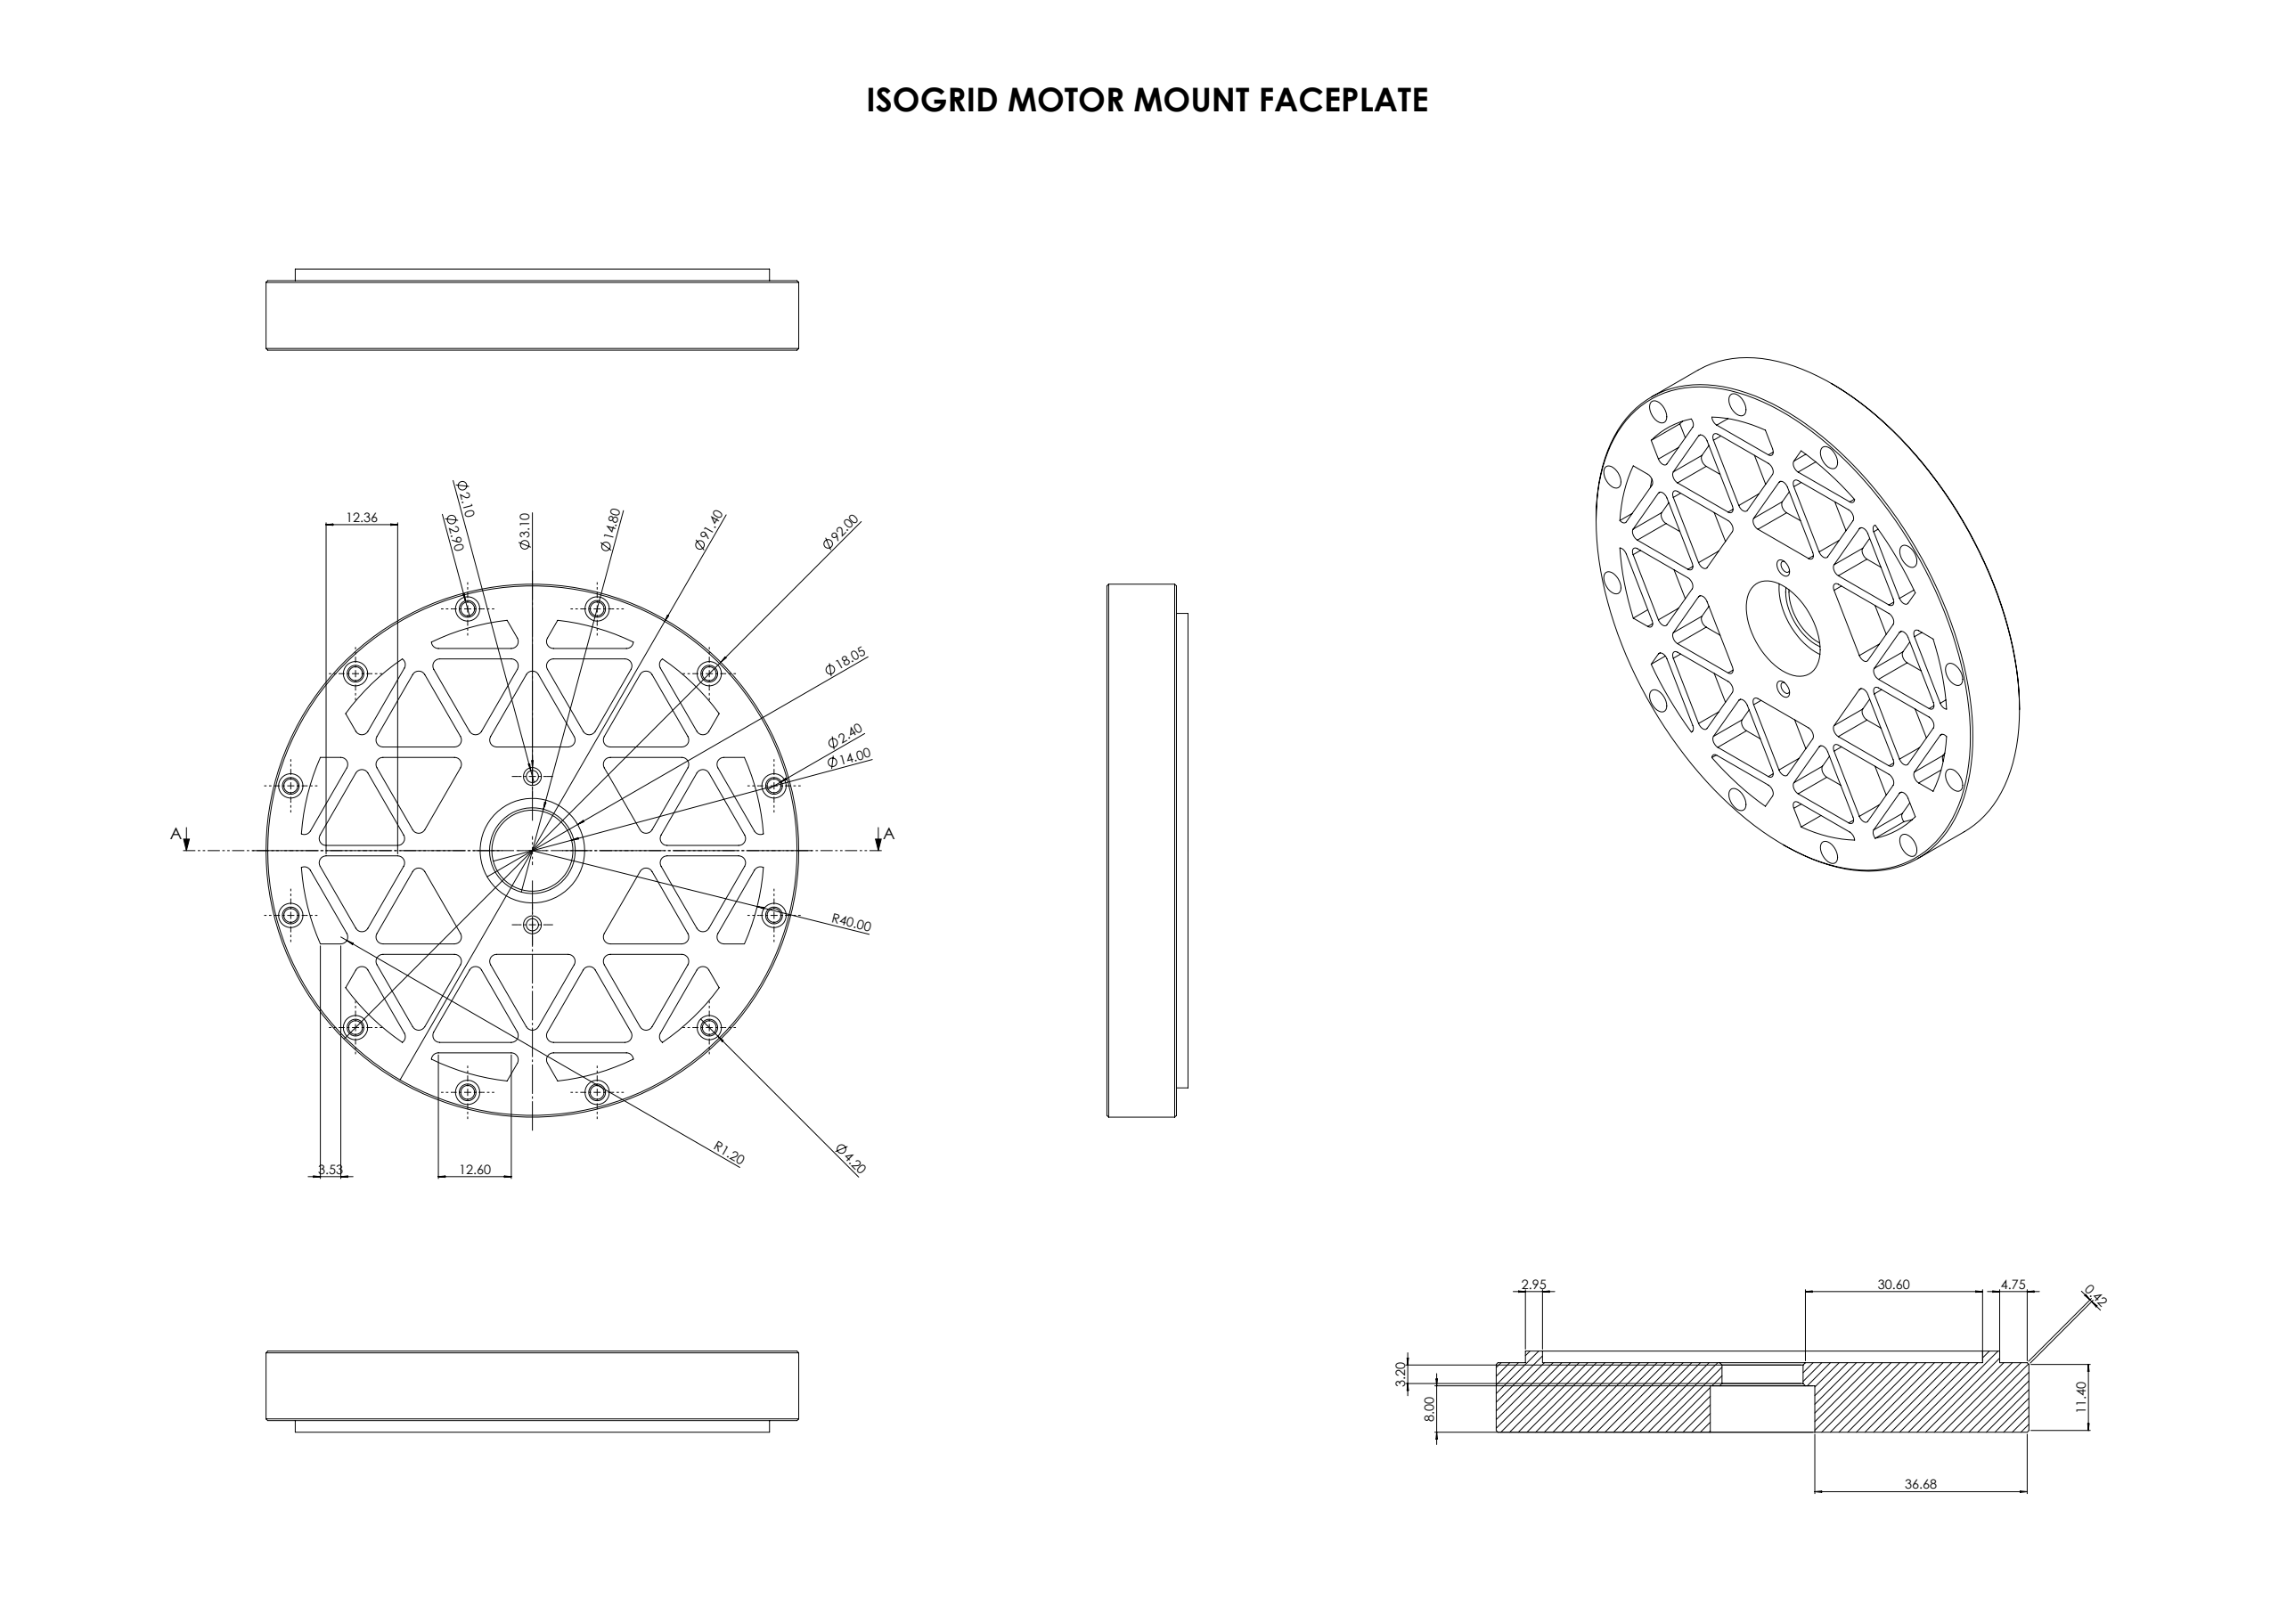
ISO-10303-21;
HEADER;
/* Generated by software containing ST-Developer
 * from STEP Tools, Inc. (www.steptools.com) 
 */

FILE_DESCRIPTION(
/* description */ (''),
/* implementation_level */ '2;1');

FILE_NAME(
/* name */ '03_Isogrid_Motor_Mount_Faceplate.step',
/* time_stamp */ '2026-10-19T23:00:43-07:00',
/* author */ (''),
/* organization */ (''),
/* preprocessor_version */ 'ST-DEVELOPER v20.2',
/* originating_system */ 'Autodesk Translation Framework v15.15.0.0',
/* authorisation */ '');

FILE_SCHEMA (('AUTOMOTIVE_DESIGN { 1 0 10303 214 3 1 1 }'));
ENDSEC;

DATA;
#10=MECHANICAL_DESIGN_GEOMETRIC_PRESENTATION_REPRESENTATION('',(#998),#55002);
#958=SHAPE_REPRESENTATION_RELATIONSHIP('SRR','None',#55106,#978);
#978=ADVANCED_BREP_SHAPE_REPRESENTATION('',(#1018),#54984);
#998=STYLED_ITEM('',(#55400),#1018);
#1018=MANIFOLD_SOLID_BREP('Isogrid Faceplate',#24531);
#1082=FACE_BOUND('',#3973,.T.);
#1083=FACE_BOUND('',#3979,.T.);
#1084=FACE_BOUND('',#3985,.T.);
#1085=FACE_BOUND('',#3991,.T.);
#1086=FACE_BOUND('',#3997,.T.);
#1087=FACE_BOUND('',#4003,.T.);
#1088=FACE_BOUND('',#4009,.T.);
#1089=FACE_BOUND('',#4015,.T.);
#1090=FACE_BOUND('',#4021,.T.);
#1091=FACE_BOUND('',#4027,.T.);
#1092=FACE_BOUND('',#4033,.T.);
#1093=FACE_BOUND('',#4039,.T.);
#1094=FACE_BOUND('',#4044,.T.);
#1095=FACE_BOUND('',#4045,.T.);
#1096=FACE_BOUND('',#4046,.T.);
#1097=FACE_BOUND('',#4047,.T.);
#1098=FACE_BOUND('',#4050,.T.);
#1099=FACE_BOUND('',#4054,.T.);
#1100=FACE_BOUND('',#4055,.T.);
#1101=FACE_BOUND('',#4056,.T.);
#1102=FACE_BOUND('',#4057,.T.);
#1103=FACE_BOUND('',#4058,.T.);
#1104=FACE_BOUND('',#4059,.T.);
#1105=FACE_BOUND('',#4060,.T.);
#1106=FACE_BOUND('',#4061,.T.);
#1107=FACE_BOUND('',#4062,.T.);
#1108=FACE_BOUND('',#4063,.T.);
#1109=FACE_BOUND('',#4064,.T.);
#1110=FACE_BOUND('',#4065,.T.);
#1111=FACE_BOUND('',#4066,.T.);
#1112=FACE_BOUND('',#4069,.T.);
#1113=FACE_BOUND('',#4070,.T.);
#1114=FACE_BOUND('',#4071,.T.);
#1115=FACE_BOUND('',#4072,.T.);
#1116=FACE_BOUND('',#4073,.T.);
#1117=FACE_BOUND('',#4074,.T.);
#1118=FACE_BOUND('',#4075,.T.);
#1119=FACE_BOUND('',#4076,.T.);
#1120=FACE_BOUND('',#4077,.T.);
#1121=FACE_BOUND('',#4078,.T.);
#1122=FACE_BOUND('',#4079,.T.);
#1123=FACE_BOUND('',#4080,.T.);
#1124=FACE_BOUND('',#4081,.T.);
#1125=FACE_BOUND('',#4082,.T.);
#1126=FACE_BOUND('',#4083,.T.);
#1127=FACE_BOUND('',#4084,.T.);
#1128=FACE_BOUND('',#4085,.T.);
#1129=FACE_BOUND('',#4086,.T.);
#1130=FACE_BOUND('',#4087,.T.);
#1131=FACE_BOUND('',#4088,.T.);
#1132=FACE_BOUND('',#4089,.T.);
#1133=FACE_BOUND('',#4090,.T.);
#1134=FACE_BOUND('',#4091,.T.);
#1135=FACE_BOUND('',#4092,.T.);
#1136=FACE_BOUND('',#4093,.T.);
#1137=FACE_BOUND('',#4094,.T.);
#1138=FACE_BOUND('',#4095,.T.);
#1139=FACE_BOUND('',#4096,.T.);
#1140=FACE_BOUND('',#4097,.T.);
#1141=FACE_BOUND('',#4098,.T.);
#1142=FACE_BOUND('',#4099,.T.);
#1143=FACE_BOUND('',#4100,.T.);
#1144=FACE_BOUND('',#4101,.T.);
#1145=FACE_BOUND('',#4102,.T.);
#1146=FACE_BOUND('',#4103,.T.);
#1147=FACE_BOUND('',#4104,.T.);
#1148=FACE_BOUND('',#4105,.T.);
#1149=FACE_BOUND('',#4106,.T.);
#1150=FACE_BOUND('',#4107,.T.);
#1151=FACE_BOUND('',#4108,.T.);
#1152=FACE_BOUND('',#4109,.T.);
#1153=FACE_BOUND('',#4110,.T.);
#1154=FACE_BOUND('',#4111,.T.);
#1155=FACE_BOUND('',#4112,.T.);
#1156=FACE_BOUND('',#4113,.T.);
#1157=FACE_BOUND('',#4314,.T.);
#1289=PLANE('',#25096);
#1290=PLANE('',#25107);
#1291=PLANE('',#25118);
#1292=PLANE('',#25129);
#1293=PLANE('',#25140);
#1294=PLANE('',#25151);
#1295=PLANE('',#25162);
#1296=PLANE('',#25173);
#1297=PLANE('',#25184);
#1298=PLANE('',#25195);
#1299=PLANE('',#25206);
#1300=PLANE('',#25217);
#1301=PLANE('',#25228);
#1302=PLANE('',#25232);
#1303=PLANE('',#25241);
#1304=PLANE('',#25245);
#1305=PLANE('',#25341);
#1306=PLANE('',#25344);
#1307=PLANE('',#25348);
#1308=PLANE('',#25351);
#1309=PLANE('',#25353);
#1310=PLANE('',#25357);
#1311=PLANE('',#25360);
#1312=PLANE('',#25362);
#1313=PLANE('',#25368);
#1314=PLANE('',#25371);
#1315=PLANE('',#25373);
#1316=PLANE('',#25377);
#1317=PLANE('',#25380);
#1318=PLANE('',#25382);
#1319=PLANE('',#25386);
#1320=PLANE('',#25389);
#1321=PLANE('',#25392);
#1322=PLANE('',#25396);
#1323=PLANE('',#25399);
#1324=PLANE('',#25401);
#1325=PLANE('',#25405);
#1326=PLANE('',#25408);
#1327=PLANE('',#25410);
#1328=PLANE('',#25414);
#1329=PLANE('',#25417);
#1330=PLANE('',#25419);
#1331=PLANE('',#25422);
#1332=PLANE('',#25425);
#1333=PLANE('',#25427);
#1334=PLANE('',#25431);
#1335=PLANE('',#25434);
#1336=PLANE('',#25436);
#1337=PLANE('',#25440);
#1338=PLANE('',#25443);
#1339=PLANE('',#25446);
#1340=PLANE('',#25450);
#1341=PLANE('',#25453);
#1342=PLANE('',#25455);
#1343=PLANE('',#25459);
#1344=PLANE('',#25462);
#1345=PLANE('',#25464);
#1346=PLANE('',#25468);
#1347=PLANE('',#25471);
#1348=PLANE('',#25473);
#1349=PLANE('',#25479);
#1350=PLANE('',#25482);
#1351=PLANE('',#25484);
#1352=PLANE('',#25488);
#1353=PLANE('',#25491);
#1354=PLANE('',#25493);
#1355=PLANE('',#25497);
#1356=PLANE('',#25500);
#1357=PLANE('',#25502);
#1358=PLANE('',#25505);
#1359=PLANE('',#25508);
#1360=PLANE('',#25510);
#1361=PLANE('',#25514);
#1362=PLANE('',#25517);
#1363=PLANE('',#25519);
#1364=PLANE('',#25525);
#1365=PLANE('',#25527);
#1366=PLANE('',#25530);
#1367=PLANE('',#25533);
#1368=PLANE('',#25535);
#1369=PLANE('',#25539);
#1370=PLANE('',#25542);
#1371=PLANE('',#25544);
#1372=PLANE('',#25548);
#1373=PLANE('',#25551);
#1374=PLANE('',#25553);
#1375=PLANE('',#25557);
#1376=PLANE('',#25559);
#1377=PLANE('',#25562);
#1378=PLANE('',#25565);
#1379=PLANE('',#25569);
#1380=PLANE('',#25571);
#1381=PLANE('',#25574);
#1382=PLANE('',#25578);
#1383=PLANE('',#25580);
#1384=PLANE('',#25583);
#1385=PLANE('',#25597);
#1386=PLANE('',#25598);
#1387=PLANE('',#25599);
#1388=PLANE('',#25600);
#1389=PLANE('',#25601);
#1390=PLANE('',#25602);
#1391=PLANE('',#25603);
#1392=PLANE('',#25604);
#1393=PLANE('',#25605);
#1394=PLANE('',#25606);
#1395=PLANE('',#25607);
#1396=PLANE('',#25608);
#1397=PLANE('',#25609);
#1398=PLANE('',#25610);
#1399=PLANE('',#25611);
#1400=PLANE('',#25612);
#1401=PLANE('',#25613);
#1402=PLANE('',#25614);
#1403=PLANE('',#25615);
#1404=PLANE('',#25616);
#1405=PLANE('',#25617);
#1406=PLANE('',#25618);
#1407=PLANE('',#25619);
#1408=PLANE('',#25620);
#1409=PLANE('',#25621);
#1410=PLANE('',#25622);
#1411=PLANE('',#25623);
#1412=PLANE('',#25624);
#1413=PLANE('',#25627);
#1992=CYLINDRICAL_SURFACE('',#25061,0.105);
#1993=CYLINDRICAL_SURFACE('',#25067,0.105);
#1994=CYLINDRICAL_SURFACE('',#25073,0.13);
#1995=CYLINDRICAL_SURFACE('',#25079,0.13);
#1996=CYLINDRICAL_SURFACE('',#25085,0.13);
#1997=CYLINDRICAL_SURFACE('',#25092,0.12);
#1998=CYLINDRICAL_SURFACE('',#25098,0.21);
#1999=CYLINDRICAL_SURFACE('',#25103,0.12);
#2000=CYLINDRICAL_SURFACE('',#25109,0.21);
#2001=CYLINDRICAL_SURFACE('',#25114,0.12);
#2002=CYLINDRICAL_SURFACE('',#25120,0.21);
#2003=CYLINDRICAL_SURFACE('',#25125,0.12);
#2004=CYLINDRICAL_SURFACE('',#25131,0.21);
#2005=CYLINDRICAL_SURFACE('',#25136,0.12);
#2006=CYLINDRICAL_SURFACE('',#25142,0.21);
#2007=CYLINDRICAL_SURFACE('',#25147,0.120000000000001);
#2008=CYLINDRICAL_SURFACE('',#25153,0.21);
#2009=CYLINDRICAL_SURFACE('',#25158,0.12);
#2010=CYLINDRICAL_SURFACE('',#25164,0.21);
#2011=CYLINDRICAL_SURFACE('',#25169,0.12);
#2012=CYLINDRICAL_SURFACE('',#25175,0.21);
#2013=CYLINDRICAL_SURFACE('',#25180,0.12);
#2014=CYLINDRICAL_SURFACE('',#25186,0.21);
#2015=CYLINDRICAL_SURFACE('',#25191,0.12);
#2016=CYLINDRICAL_SURFACE('',#25197,0.21);
#2017=CYLINDRICAL_SURFACE('',#25202,0.12);
#2018=CYLINDRICAL_SURFACE('',#25208,0.21);
#2019=CYLINDRICAL_SURFACE('',#25213,0.12);
#2020=CYLINDRICAL_SURFACE('',#25219,0.21);
#2021=CYLINDRICAL_SURFACE('',#25225,0.7);
#2022=CYLINDRICAL_SURFACE('',#25238,4.6);
#2023=CYLINDRICAL_SURFACE('',#25337,0.12);
#2024=CYLINDRICAL_SURFACE('',#25339,0.12);
#2025=CYLINDRICAL_SURFACE('',#25342,0.12);
#2026=CYLINDRICAL_SURFACE('',#25346,0.12);
#2027=CYLINDRICAL_SURFACE('',#25349,0.12);
#2028=CYLINDRICAL_SURFACE('',#25354,0.12);
#2029=CYLINDRICAL_SURFACE('',#25355,0.12);
#2030=CYLINDRICAL_SURFACE('',#25358,0.12);
#2031=CYLINDRICAL_SURFACE('',#25363,0.12);
#2032=CYLINDRICAL_SURFACE('',#25364,0.12);
#2033=CYLINDRICAL_SURFACE('',#25366,0.12);
#2034=CYLINDRICAL_SURFACE('',#25369,0.12);
#2035=CYLINDRICAL_SURFACE('',#25374,0.12);
#2036=CYLINDRICAL_SURFACE('',#25375,0.12);
#2037=CYLINDRICAL_SURFACE('',#25378,0.12);
#2038=CYLINDRICAL_SURFACE('',#25383,0.12);
#2039=CYLINDRICAL_SURFACE('',#25384,0.12);
#2040=CYLINDRICAL_SURFACE('',#25387,0.12);
#2041=CYLINDRICAL_SURFACE('',#25393,0.12);
#2042=CYLINDRICAL_SURFACE('',#25394,0.12);
#2043=CYLINDRICAL_SURFACE('',#25397,0.12);
#2044=CYLINDRICAL_SURFACE('',#25402,0.12);
#2045=CYLINDRICAL_SURFACE('',#25403,0.12);
#2046=CYLINDRICAL_SURFACE('',#25406,0.12);
#2047=CYLINDRICAL_SURFACE('',#25411,0.12);
#2048=CYLINDRICAL_SURFACE('',#25412,0.12);
#2049=CYLINDRICAL_SURFACE('',#25418,0.12);
#2050=CYLINDRICAL_SURFACE('',#25420,0.12);
#2051=CYLINDRICAL_SURFACE('',#25423,0.12);
#2052=CYLINDRICAL_SURFACE('',#25428,0.12);
#2053=CYLINDRICAL_SURFACE('',#25429,0.12);
#2054=CYLINDRICAL_SURFACE('',#25432,0.12);
#2055=CYLINDRICAL_SURFACE('',#25437,0.12);
#2056=CYLINDRICAL_SURFACE('',#25438,0.12);
#2057=CYLINDRICAL_SURFACE('',#25441,0.12);
#2058=CYLINDRICAL_SURFACE('',#25447,0.12);
#2059=CYLINDRICAL_SURFACE('',#25448,0.12);
#2060=CYLINDRICAL_SURFACE('',#25451,0.12);
#2061=CYLINDRICAL_SURFACE('',#25456,0.12);
#2062=CYLINDRICAL_SURFACE('',#25457,0.12);
#2063=CYLINDRICAL_SURFACE('',#25460,0.12);
#2064=CYLINDRICAL_SURFACE('',#25465,0.12);
#2065=CYLINDRICAL_SURFACE('',#25466,0.12);
#2066=CYLINDRICAL_SURFACE('',#25469,0.12);
#2067=CYLINDRICAL_SURFACE('',#25474,0.12);
#2068=CYLINDRICAL_SURFACE('',#25475,0.12);
#2069=CYLINDRICAL_SURFACE('',#25477,0.12);
#2070=CYLINDRICAL_SURFACE('',#25480,0.12);
#2071=CYLINDRICAL_SURFACE('',#25485,0.12);
#2072=CYLINDRICAL_SURFACE('',#25486,0.12);
#2073=CYLINDRICAL_SURFACE('',#25489,0.12);
#2074=CYLINDRICAL_SURFACE('',#25494,0.12);
#2075=CYLINDRICAL_SURFACE('',#25495,0.12);
#2076=CYLINDRICAL_SURFACE('',#25501,0.12);
#2077=CYLINDRICAL_SURFACE('',#25503,0.12);
#2078=CYLINDRICAL_SURFACE('',#25506,0.12);
#2079=CYLINDRICAL_SURFACE('',#25511,0.12);
#2080=CYLINDRICAL_SURFACE('',#25512,0.12);
#2081=CYLINDRICAL_SURFACE('',#25515,0.12);
#2082=CYLINDRICAL_SURFACE('',#25520,0.12);
#2083=CYLINDRICAL_SURFACE('',#25521,0.12);
#2084=CYLINDRICAL_SURFACE('',#25523,0.12);
#2085=CYLINDRICAL_SURFACE('',#25528,0.12);
#2086=CYLINDRICAL_SURFACE('',#25531,0.12);
#2087=CYLINDRICAL_SURFACE('',#25536,0.12);
#2088=CYLINDRICAL_SURFACE('',#25537,0.12);
#2089=CYLINDRICAL_SURFACE('',#25540,0.12);
#2090=CYLINDRICAL_SURFACE('',#25545,0.12);
#2091=CYLINDRICAL_SURFACE('',#25546,0.12);
#2092=CYLINDRICAL_SURFACE('',#25549,0.12);
#2093=CYLINDRICAL_SURFACE('',#25554,0.12);
#2094=CYLINDRICAL_SURFACE('',#25555,0.12);
#2095=CYLINDRICAL_SURFACE('',#25560,0.12);
#2096=CYLINDRICAL_SURFACE('',#25563,0.12);
#2097=CYLINDRICAL_SURFACE('',#25567,0.12);
#2098=CYLINDRICAL_SURFACE('',#25572,0.12);
#2099=CYLINDRICAL_SURFACE('',#25576,0.12);
#2100=CYLINDRICAL_SURFACE('',#25581,0.12);
#2101=CYLINDRICAL_SURFACE('',#25585,4.);
#2102=CYLINDRICAL_SURFACE('',#25586,4.);
#2103=CYLINDRICAL_SURFACE('',#25587,4.);
#2104=CYLINDRICAL_SURFACE('',#25588,4.);
#2105=CYLINDRICAL_SURFACE('',#25589,4.);
#2106=CYLINDRICAL_SURFACE('',#25590,4.);
#2107=CYLINDRICAL_SURFACE('',#25591,4.);
#2108=CYLINDRICAL_SURFACE('',#25592,4.);
#2109=CYLINDRICAL_SURFACE('',#25593,4.);
#2110=CYLINDRICAL_SURFACE('',#25594,4.);
#2111=CYLINDRICAL_SURFACE('',#25595,4.);
#2112=CYLINDRICAL_SURFACE('',#25596,4.);
#2113=CYLINDRICAL_SURFACE('',#25625,3.8);
#2114=CYLINDRICAL_SURFACE('',#25629,4.095);
#2115=CYLINDRICAL_SURFACE('',#25630,0.9025);
#2544=FACE_OUTER_BOUND('',#3954,.T.);
#2545=FACE_OUTER_BOUND('',#3955,.T.);
#2546=FACE_OUTER_BOUND('',#3956,.T.);
#2547=FACE_OUTER_BOUND('',#3957,.T.);
#2548=FACE_OUTER_BOUND('',#3958,.T.);
#2549=FACE_OUTER_BOUND('',#3959,.T.);
#2550=FACE_OUTER_BOUND('',#3960,.T.);
#2551=FACE_OUTER_BOUND('',#3961,.T.);
#2552=FACE_OUTER_BOUND('',#3962,.T.);
#2553=FACE_OUTER_BOUND('',#3963,.T.);
#2554=FACE_OUTER_BOUND('',#3964,.T.);
#2555=FACE_OUTER_BOUND('',#3965,.T.);
#2556=FACE_OUTER_BOUND('',#3966,.T.);
#2557=FACE_OUTER_BOUND('',#3967,.T.);
#2558=FACE_OUTER_BOUND('',#3968,.T.);
#2559=FACE_OUTER_BOUND('',#3969,.T.);
#2560=FACE_OUTER_BOUND('',#3970,.T.);
#2561=FACE_OUTER_BOUND('',#3971,.T.);
#2562=FACE_OUTER_BOUND('',#3972,.T.);
#2563=FACE_OUTER_BOUND('',#3974,.T.);
#2564=FACE_OUTER_BOUND('',#3975,.T.);
#2565=FACE_OUTER_BOUND('',#3976,.T.);
#2566=FACE_OUTER_BOUND('',#3977,.T.);
#2567=FACE_OUTER_BOUND('',#3978,.T.);
#2568=FACE_OUTER_BOUND('',#3980,.T.);
#2569=FACE_OUTER_BOUND('',#3981,.T.);
#2570=FACE_OUTER_BOUND('',#3982,.T.);
#2571=FACE_OUTER_BOUND('',#3983,.T.);
#2572=FACE_OUTER_BOUND('',#3984,.T.);
#2573=FACE_OUTER_BOUND('',#3986,.T.);
#2574=FACE_OUTER_BOUND('',#3987,.T.);
#2575=FACE_OUTER_BOUND('',#3988,.T.);
#2576=FACE_OUTER_BOUND('',#3989,.T.);
#2577=FACE_OUTER_BOUND('',#3990,.T.);
#2578=FACE_OUTER_BOUND('',#3992,.T.);
#2579=FACE_OUTER_BOUND('',#3993,.T.);
#2580=FACE_OUTER_BOUND('',#3994,.T.);
#2581=FACE_OUTER_BOUND('',#3995,.T.);
#2582=FACE_OUTER_BOUND('',#3996,.T.);
#2583=FACE_OUTER_BOUND('',#3998,.T.);
#2584=FACE_OUTER_BOUND('',#3999,.T.);
#2585=FACE_OUTER_BOUND('',#4000,.T.);
#2586=FACE_OUTER_BOUND('',#4001,.T.);
#2587=FACE_OUTER_BOUND('',#4002,.T.);
#2588=FACE_OUTER_BOUND('',#4004,.T.);
#2589=FACE_OUTER_BOUND('',#4005,.T.);
#2590=FACE_OUTER_BOUND('',#4006,.T.);
#2591=FACE_OUTER_BOUND('',#4007,.T.);
#2592=FACE_OUTER_BOUND('',#4008,.T.);
#2593=FACE_OUTER_BOUND('',#4010,.T.);
#2594=FACE_OUTER_BOUND('',#4011,.T.);
#2595=FACE_OUTER_BOUND('',#4012,.T.);
#2596=FACE_OUTER_BOUND('',#4013,.T.);
#2597=FACE_OUTER_BOUND('',#4014,.T.);
#2598=FACE_OUTER_BOUND('',#4016,.T.);
#2599=FACE_OUTER_BOUND('',#4017,.T.);
#2600=FACE_OUTER_BOUND('',#4018,.T.);
#2601=FACE_OUTER_BOUND('',#4019,.T.);
#2602=FACE_OUTER_BOUND('',#4020,.T.);
#2603=FACE_OUTER_BOUND('',#4022,.T.);
#2604=FACE_OUTER_BOUND('',#4023,.T.);
#2605=FACE_OUTER_BOUND('',#4024,.T.);
#2606=FACE_OUTER_BOUND('',#4025,.T.);
#2607=FACE_OUTER_BOUND('',#4026,.T.);
#2608=FACE_OUTER_BOUND('',#4028,.T.);
#2609=FACE_OUTER_BOUND('',#4029,.T.);
#2610=FACE_OUTER_BOUND('',#4030,.T.);
#2611=FACE_OUTER_BOUND('',#4031,.T.);
#2612=FACE_OUTER_BOUND('',#4032,.T.);
#2613=FACE_OUTER_BOUND('',#4034,.T.);
#2614=FACE_OUTER_BOUND('',#4035,.T.);
#2615=FACE_OUTER_BOUND('',#4036,.T.);
#2616=FACE_OUTER_BOUND('',#4037,.T.);
#2617=FACE_OUTER_BOUND('',#4038,.T.);
#2618=FACE_OUTER_BOUND('',#4040,.T.);
#2619=FACE_OUTER_BOUND('',#4041,.T.);
#2620=FACE_OUTER_BOUND('',#4042,.T.);
#2621=FACE_OUTER_BOUND('',#4043,.T.);
#2622=FACE_OUTER_BOUND('',#4048,.T.);
#2623=FACE_OUTER_BOUND('',#4049,.T.);
#2624=FACE_OUTER_BOUND('',#4051,.T.);
#2625=FACE_OUTER_BOUND('',#4052,.T.);
#2626=FACE_OUTER_BOUND('',#4053,.T.);
#2627=FACE_OUTER_BOUND('',#4067,.T.);
#2628=FACE_OUTER_BOUND('',#4068,.T.);
#2629=FACE_OUTER_BOUND('',#4114,.T.);
#2630=FACE_OUTER_BOUND('',#4115,.T.);
#2631=FACE_OUTER_BOUND('',#4116,.T.);
#2632=FACE_OUTER_BOUND('',#4117,.T.);
#2633=FACE_OUTER_BOUND('',#4118,.T.);
#2634=FACE_OUTER_BOUND('',#4119,.T.);
#2635=FACE_OUTER_BOUND('',#4120,.T.);
#2636=FACE_OUTER_BOUND('',#4121,.T.);
#2637=FACE_OUTER_BOUND('',#4122,.T.);
#2638=FACE_OUTER_BOUND('',#4123,.T.);
#2639=FACE_OUTER_BOUND('',#4124,.T.);
#2640=FACE_OUTER_BOUND('',#4125,.T.);
#2641=FACE_OUTER_BOUND('',#4126,.T.);
#2642=FACE_OUTER_BOUND('',#4127,.T.);
#2643=FACE_OUTER_BOUND('',#4128,.T.);
#2644=FACE_OUTER_BOUND('',#4129,.T.);
#2645=FACE_OUTER_BOUND('',#4130,.T.);
#2646=FACE_OUTER_BOUND('',#4131,.T.);
#2647=FACE_OUTER_BOUND('',#4132,.T.);
#2648=FACE_OUTER_BOUND('',#4133,.T.);
#2649=FACE_OUTER_BOUND('',#4134,.T.);
#2650=FACE_OUTER_BOUND('',#4135,.T.);
#2651=FACE_OUTER_BOUND('',#4136,.T.);
#2652=FACE_OUTER_BOUND('',#4137,.T.);
#2653=FACE_OUTER_BOUND('',#4138,.T.);
#2654=FACE_OUTER_BOUND('',#4139,.T.);
#2655=FACE_OUTER_BOUND('',#4140,.T.);
#2656=FACE_OUTER_BOUND('',#4141,.T.);
#2657=FACE_OUTER_BOUND('',#4142,.T.);
#2658=FACE_OUTER_BOUND('',#4143,.T.);
#2659=FACE_OUTER_BOUND('',#4144,.T.);
#2660=FACE_OUTER_BOUND('',#4145,.T.);
#2661=FACE_OUTER_BOUND('',#4146,.T.);
#2662=FACE_OUTER_BOUND('',#4147,.T.);
#2663=FACE_OUTER_BOUND('',#4148,.T.);
#2664=FACE_OUTER_BOUND('',#4149,.T.);
#2665=FACE_OUTER_BOUND('',#4150,.T.);
#2666=FACE_OUTER_BOUND('',#4151,.T.);
#2667=FACE_OUTER_BOUND('',#4152,.T.);
#2668=FACE_OUTER_BOUND('',#4153,.T.);
#2669=FACE_OUTER_BOUND('',#4154,.T.);
#2670=FACE_OUTER_BOUND('',#4155,.T.);
#2671=FACE_OUTER_BOUND('',#4156,.T.);
#2672=FACE_OUTER_BOUND('',#4157,.T.);
#2673=FACE_OUTER_BOUND('',#4158,.T.);
#2674=FACE_OUTER_BOUND('',#4159,.T.);
#2675=FACE_OUTER_BOUND('',#4160,.T.);
#2676=FACE_OUTER_BOUND('',#4161,.T.);
#2677=FACE_OUTER_BOUND('',#4162,.T.);
#2678=FACE_OUTER_BOUND('',#4163,.T.);
#2679=FACE_OUTER_BOUND('',#4164,.T.);
#2680=FACE_OUTER_BOUND('',#4165,.T.);
#2681=FACE_OUTER_BOUND('',#4166,.T.);
#2682=FACE_OUTER_BOUND('',#4167,.T.);
#2683=FACE_OUTER_BOUND('',#4168,.T.);
#2684=FACE_OUTER_BOUND('',#4169,.T.);
#2685=FACE_OUTER_BOUND('',#4170,.T.);
#2686=FACE_OUTER_BOUND('',#4171,.T.);
#2687=FACE_OUTER_BOUND('',#4172,.T.);
#2688=FACE_OUTER_BOUND('',#4173,.T.);
#2689=FACE_OUTER_BOUND('',#4174,.T.);
#2690=FACE_OUTER_BOUND('',#4175,.T.);
#2691=FACE_OUTER_BOUND('',#4176,.T.);
#2692=FACE_OUTER_BOUND('',#4177,.T.);
#2693=FACE_OUTER_BOUND('',#4178,.T.);
#2694=FACE_OUTER_BOUND('',#4179,.T.);
#2695=FACE_OUTER_BOUND('',#4180,.T.);
#2696=FACE_OUTER_BOUND('',#4181,.T.);
#2697=FACE_OUTER_BOUND('',#4182,.T.);
#2698=FACE_OUTER_BOUND('',#4183,.T.);
#2699=FACE_OUTER_BOUND('',#4184,.T.);
#2700=FACE_OUTER_BOUND('',#4185,.T.);
#2701=FACE_OUTER_BOUND('',#4186,.T.);
#2702=FACE_OUTER_BOUND('',#4187,.T.);
#2703=FACE_OUTER_BOUND('',#4188,.T.);
#2704=FACE_OUTER_BOUND('',#4189,.T.);
#2705=FACE_OUTER_BOUND('',#4190,.T.);
#2706=FACE_OUTER_BOUND('',#4191,.T.);
#2707=FACE_OUTER_BOUND('',#4192,.T.);
#2708=FACE_OUTER_BOUND('',#4193,.T.);
#2709=FACE_OUTER_BOUND('',#4194,.T.);
#2710=FACE_OUTER_BOUND('',#4195,.T.);
#2711=FACE_OUTER_BOUND('',#4196,.T.);
#2712=FACE_OUTER_BOUND('',#4197,.T.);
#2713=FACE_OUTER_BOUND('',#4198,.T.);
#2714=FACE_OUTER_BOUND('',#4199,.T.);
#2715=FACE_OUTER_BOUND('',#4200,.T.);
#2716=FACE_OUTER_BOUND('',#4201,.T.);
#2717=FACE_OUTER_BOUND('',#4202,.T.);
#2718=FACE_OUTER_BOUND('',#4203,.T.);
#2719=FACE_OUTER_BOUND('',#4204,.T.);
#2720=FACE_OUTER_BOUND('',#4205,.T.);
#2721=FACE_OUTER_BOUND('',#4206,.T.);
#2722=FACE_OUTER_BOUND('',#4207,.T.);
#2723=FACE_OUTER_BOUND('',#4208,.T.);
#2724=FACE_OUTER_BOUND('',#4209,.T.);
#2725=FACE_OUTER_BOUND('',#4210,.T.);
#2726=FACE_OUTER_BOUND('',#4211,.T.);
#2727=FACE_OUTER_BOUND('',#4212,.T.);
#2728=FACE_OUTER_BOUND('',#4213,.T.);
#2729=FACE_OUTER_BOUND('',#4214,.T.);
#2730=FACE_OUTER_BOUND('',#4215,.T.);
#2731=FACE_OUTER_BOUND('',#4216,.T.);
#2732=FACE_OUTER_BOUND('',#4217,.T.);
#2733=FACE_OUTER_BOUND('',#4218,.T.);
#2734=FACE_OUTER_BOUND('',#4219,.T.);
#2735=FACE_OUTER_BOUND('',#4220,.T.);
#2736=FACE_OUTER_BOUND('',#4221,.T.);
#2737=FACE_OUTER_BOUND('',#4222,.T.);
#2738=FACE_OUTER_BOUND('',#4223,.T.);
#2739=FACE_OUTER_BOUND('',#4224,.T.);
#2740=FACE_OUTER_BOUND('',#4225,.T.);
#2741=FACE_OUTER_BOUND('',#4226,.T.);
#2742=FACE_OUTER_BOUND('',#4227,.T.);
#2743=FACE_OUTER_BOUND('',#4228,.T.);
#2744=FACE_OUTER_BOUND('',#4229,.T.);
#2745=FACE_OUTER_BOUND('',#4230,.T.);
#2746=FACE_OUTER_BOUND('',#4231,.T.);
#2747=FACE_OUTER_BOUND('',#4232,.T.);
#2748=FACE_OUTER_BOUND('',#4233,.T.);
#2749=FACE_OUTER_BOUND('',#4234,.T.);
#2750=FACE_OUTER_BOUND('',#4235,.T.);
#2751=FACE_OUTER_BOUND('',#4236,.T.);
#2752=FACE_OUTER_BOUND('',#4237,.T.);
#2753=FACE_OUTER_BOUND('',#4238,.T.);
#2754=FACE_OUTER_BOUND('',#4239,.T.);
#2755=FACE_OUTER_BOUND('',#4240,.T.);
#2756=FACE_OUTER_BOUND('',#4241,.T.);
#2757=FACE_OUTER_BOUND('',#4242,.T.);
#2758=FACE_OUTER_BOUND('',#4243,.T.);
#2759=FACE_OUTER_BOUND('',#4244,.T.);
#2760=FACE_OUTER_BOUND('',#4245,.T.);
#2761=FACE_OUTER_BOUND('',#4246,.T.);
#2762=FACE_OUTER_BOUND('',#4247,.T.);
#2763=FACE_OUTER_BOUND('',#4248,.T.);
#2764=FACE_OUTER_BOUND('',#4249,.T.);
#2765=FACE_OUTER_BOUND('',#4250,.T.);
#2766=FACE_OUTER_BOUND('',#4251,.T.);
#2767=FACE_OUTER_BOUND('',#4252,.T.);
#2768=FACE_OUTER_BOUND('',#4253,.T.);
#2769=FACE_OUTER_BOUND('',#4254,.T.);
#2770=FACE_OUTER_BOUND('',#4255,.T.);
#2771=FACE_OUTER_BOUND('',#4256,.T.);
#2772=FACE_OUTER_BOUND('',#4257,.T.);
#2773=FACE_OUTER_BOUND('',#4258,.T.);
#2774=FACE_OUTER_BOUND('',#4259,.T.);
#2775=FACE_OUTER_BOUND('',#4260,.T.);
#2776=FACE_OUTER_BOUND('',#4261,.T.);
#2777=FACE_OUTER_BOUND('',#4262,.T.);
#2778=FACE_OUTER_BOUND('',#4263,.T.);
#2779=FACE_OUTER_BOUND('',#4264,.T.);
#2780=FACE_OUTER_BOUND('',#4265,.T.);
#2781=FACE_OUTER_BOUND('',#4266,.T.);
#2782=FACE_OUTER_BOUND('',#4267,.T.);
#2783=FACE_OUTER_BOUND('',#4268,.T.);
#2784=FACE_OUTER_BOUND('',#4269,.T.);
#2785=FACE_OUTER_BOUND('',#4270,.T.);
#2786=FACE_OUTER_BOUND('',#4271,.T.);
#2787=FACE_OUTER_BOUND('',#4272,.T.);
#2788=FACE_OUTER_BOUND('',#4273,.T.);
#2789=FACE_OUTER_BOUND('',#4274,.T.);
#2790=FACE_OUTER_BOUND('',#4275,.T.);
#2791=FACE_OUTER_BOUND('',#4276,.T.);
#2792=FACE_OUTER_BOUND('',#4277,.T.);
#2793=FACE_OUTER_BOUND('',#4278,.T.);
#2794=FACE_OUTER_BOUND('',#4279,.T.);
#2795=FACE_OUTER_BOUND('',#4280,.T.);
#2796=FACE_OUTER_BOUND('',#4281,.T.);
#2797=FACE_OUTER_BOUND('',#4282,.T.);
#2798=FACE_OUTER_BOUND('',#4283,.T.);
#2799=FACE_OUTER_BOUND('',#4284,.T.);
#2800=FACE_OUTER_BOUND('',#4285,.T.);
#2801=FACE_OUTER_BOUND('',#4286,.T.);
#2802=FACE_OUTER_BOUND('',#4287,.T.);
#2803=FACE_OUTER_BOUND('',#4288,.T.);
#2804=FACE_OUTER_BOUND('',#4289,.T.);
#2805=FACE_OUTER_BOUND('',#4290,.T.);
#2806=FACE_OUTER_BOUND('',#4291,.T.);
#2807=FACE_OUTER_BOUND('',#4292,.T.);
#2808=FACE_OUTER_BOUND('',#4293,.T.);
#2809=FACE_OUTER_BOUND('',#4294,.T.);
#2810=FACE_OUTER_BOUND('',#4295,.T.);
#2811=FACE_OUTER_BOUND('',#4296,.T.);
#2812=FACE_OUTER_BOUND('',#4297,.T.);
#2813=FACE_OUTER_BOUND('',#4298,.T.);
#2814=FACE_OUTER_BOUND('',#4299,.T.);
#2815=FACE_OUTER_BOUND('',#4300,.T.);
#2816=FACE_OUTER_BOUND('',#4301,.T.);
#2817=FACE_OUTER_BOUND('',#4302,.T.);
#2818=FACE_OUTER_BOUND('',#4303,.T.);
#2819=FACE_OUTER_BOUND('',#4304,.T.);
#2820=FACE_OUTER_BOUND('',#4305,.T.);
#2821=FACE_OUTER_BOUND('',#4306,.T.);
#2822=FACE_OUTER_BOUND('',#4307,.T.);
#2823=FACE_OUTER_BOUND('',#4308,.T.);
#2824=FACE_OUTER_BOUND('',#4309,.T.);
#2825=FACE_OUTER_BOUND('',#4310,.T.);
#2826=FACE_OUTER_BOUND('',#4311,.T.);
#2827=FACE_OUTER_BOUND('',#4312,.T.);
#2828=FACE_OUTER_BOUND('',#4313,.T.);
#2829=FACE_OUTER_BOUND('',#4315,.T.);
#2830=FACE_OUTER_BOUND('',#4316,.T.);
#3954=EDGE_LOOP('',(#16430,#16431,#16432));
#3955=EDGE_LOOP('',(#16433,#16434,#16435,#16436));
#3956=EDGE_LOOP('',(#16437,#16438,#16439,#16440));
#3957=EDGE_LOOP('',(#16441,#16442,#16443));
#3958=EDGE_LOOP('',(#16444,#16445,#16446,#16447));
#3959=EDGE_LOOP('',(#16448,#16449,#16450,#16451));
#3960=EDGE_LOOP('',(#16452,#16453,#16454));
#3961=EDGE_LOOP('',(#16455,#16456,#16457,#16458));
#3962=EDGE_LOOP('',(#16459,#16460,#16461,#16462));
#3963=EDGE_LOOP('',(#16463,#16464,#16465));
#3964=EDGE_LOOP('',(#16466,#16467,#16468,#16469));
#3965=EDGE_LOOP('',(#16470,#16471,#16472,#16473));
#3966=EDGE_LOOP('',(#16474,#16475,#16476));
#3967=EDGE_LOOP('',(#16477,#16478,#16479,#16480));
#3968=EDGE_LOOP('',(#16481,#16482,#16483,#16484));
#3969=EDGE_LOOP('',(#16485,#16486,#16487,#16488));
#3970=EDGE_LOOP('',(#16489,#16490,#16491,#16492));
#3971=EDGE_LOOP('',(#16493,#16494,#16495,#16496));
#3972=EDGE_LOOP('',(#16497));
#3973=EDGE_LOOP('',(#16498));
#3974=EDGE_LOOP('',(#16499,#16500,#16501,#16502));
#3975=EDGE_LOOP('',(#16503,#16504,#16505,#16506));
#3976=EDGE_LOOP('',(#16507,#16508,#16509,#16510));
#3977=EDGE_LOOP('',(#16511,#16512,#16513,#16514));
#3978=EDGE_LOOP('',(#16515));
#3979=EDGE_LOOP('',(#16516));
#3980=EDGE_LOOP('',(#16517,#16518,#16519,#16520));
#3981=EDGE_LOOP('',(#16521,#16522,#16523,#16524));
#3982=EDGE_LOOP('',(#16525,#16526,#16527,#16528));
#3983=EDGE_LOOP('',(#16529,#16530,#16531,#16532));
#3984=EDGE_LOOP('',(#16533));
#3985=EDGE_LOOP('',(#16534));
#3986=EDGE_LOOP('',(#16535,#16536,#16537,#16538));
#3987=EDGE_LOOP('',(#16539,#16540,#16541,#16542));
#3988=EDGE_LOOP('',(#16543,#16544,#16545,#16546));
#3989=EDGE_LOOP('',(#16547,#16548,#16549,#16550));
#3990=EDGE_LOOP('',(#16551));
#3991=EDGE_LOOP('',(#16552));
#3992=EDGE_LOOP('',(#16553,#16554,#16555,#16556));
#3993=EDGE_LOOP('',(#16557,#16558,#16559,#16560));
#3994=EDGE_LOOP('',(#16561,#16562,#16563,#16564));
#3995=EDGE_LOOP('',(#16565,#16566,#16567,#16568));
#3996=EDGE_LOOP('',(#16569));
#3997=EDGE_LOOP('',(#16570));
#3998=EDGE_LOOP('',(#16571,#16572,#16573,#16574));
#3999=EDGE_LOOP('',(#16575,#16576,#16577,#16578));
#4000=EDGE_LOOP('',(#16579,#16580,#16581,#16582));
#4001=EDGE_LOOP('',(#16583,#16584,#16585,#16586));
#4002=EDGE_LOOP('',(#16587));
#4003=EDGE_LOOP('',(#16588));
#4004=EDGE_LOOP('',(#16589,#16590,#16591,#16592));
#4005=EDGE_LOOP('',(#16593,#16594,#16595,#16596));
#4006=EDGE_LOOP('',(#16597,#16598,#16599,#16600));
#4007=EDGE_LOOP('',(#16601,#16602,#16603,#16604));
#4008=EDGE_LOOP('',(#16605));
#4009=EDGE_LOOP('',(#16606));
#4010=EDGE_LOOP('',(#16607,#16608,#16609,#16610));
#4011=EDGE_LOOP('',(#16611,#16612,#16613,#16614));
#4012=EDGE_LOOP('',(#16615,#16616,#16617,#16618));
#4013=EDGE_LOOP('',(#16619,#16620,#16621,#16622));
#4014=EDGE_LOOP('',(#16623));
#4015=EDGE_LOOP('',(#16624));
#4016=EDGE_LOOP('',(#16625,#16626,#16627,#16628));
#4017=EDGE_LOOP('',(#16629,#16630,#16631,#16632));
#4018=EDGE_LOOP('',(#16633,#16634,#16635,#16636));
#4019=EDGE_LOOP('',(#16637,#16638,#16639,#16640));
#4020=EDGE_LOOP('',(#16641));
#4021=EDGE_LOOP('',(#16642));
#4022=EDGE_LOOP('',(#16643,#16644,#16645,#16646));
#4023=EDGE_LOOP('',(#16647,#16648,#16649,#16650));
#4024=EDGE_LOOP('',(#16651,#16652,#16653,#16654));
#4025=EDGE_LOOP('',(#16655,#16656,#16657,#16658));
#4026=EDGE_LOOP('',(#16659));
#4027=EDGE_LOOP('',(#16660));
#4028=EDGE_LOOP('',(#16661,#16662,#16663,#16664));
#4029=EDGE_LOOP('',(#16665,#16666,#16667,#16668));
#4030=EDGE_LOOP('',(#16669,#16670,#16671,#16672));
#4031=EDGE_LOOP('',(#16673,#16674,#16675,#16676));
#4032=EDGE_LOOP('',(#16677));
#4033=EDGE_LOOP('',(#16678));
#4034=EDGE_LOOP('',(#16679,#16680,#16681,#16682));
#4035=EDGE_LOOP('',(#16683,#16684,#16685,#16686));
#4036=EDGE_LOOP('',(#16687,#16688,#16689,#16690));
#4037=EDGE_LOOP('',(#16691,#16692,#16693,#16694));
#4038=EDGE_LOOP('',(#16695));
#4039=EDGE_LOOP('',(#16696));
#4040=EDGE_LOOP('',(#16697,#16698,#16699,#16700));
#4041=EDGE_LOOP('',(#16701,#16702,#16703,#16704,#16705));
#4042=EDGE_LOOP('',(#16706,#16707,#16708,#16709,#16710,#16711));
#4043=EDGE_LOOP('',(#16712));
#4044=EDGE_LOOP('',(#16713));
#4045=EDGE_LOOP('',(#16714));
#4046=EDGE_LOOP('',(#16715));
#4047=EDGE_LOOP('',(#16716));
#4048=EDGE_LOOP('',(#16717,#16718,#16719,#16720,#16721));
#4049=EDGE_LOOP('',(#16722));
#4050=EDGE_LOOP('',(#16723));
#4051=EDGE_LOOP('',(#16724,#16725,#16726,#16727,#16728));
#4052=EDGE_LOOP('',(#16729,#16730,#16731,#16732,#16733,#16734));
#4053=EDGE_LOOP('',(#16735));
#4054=EDGE_LOOP('',(#16736));
#4055=EDGE_LOOP('',(#16737));
#4056=EDGE_LOOP('',(#16738));
#4057=EDGE_LOOP('',(#16739));
#4058=EDGE_LOOP('',(#16740));
#4059=EDGE_LOOP('',(#16741));
#4060=EDGE_LOOP('',(#16742));
#4061=EDGE_LOOP('',(#16743));
#4062=EDGE_LOOP('',(#16744));
#4063=EDGE_LOOP('',(#16745));
#4064=EDGE_LOOP('',(#16746));
#4065=EDGE_LOOP('',(#16747));
#4066=EDGE_LOOP('',(#16748));
#4067=EDGE_LOOP('',(#16749,#16750,#16751,#16752,#16753));
#4068=EDGE_LOOP('',(#16754));
#4069=EDGE_LOOP('',(#16755));
#4070=EDGE_LOOP('',(#16756));
#4071=EDGE_LOOP('',(#16757));
#4072=EDGE_LOOP('',(#16758));
#4073=EDGE_LOOP('',(#16759));
#4074=EDGE_LOOP('',(#16760));
#4075=EDGE_LOOP('',(#16761));
#4076=EDGE_LOOP('',(#16762,#16763,#16764,#16765,#16766));
#4077=EDGE_LOOP('',(#16767,#16768,#16769,#16770,#16771));
#4078=EDGE_LOOP('',(#16772,#16773,#16774,#16775,#16776));
#4079=EDGE_LOOP('',(#16777,#16778,#16779,#16780,#16781));
#4080=EDGE_LOOP('',(#16782,#16783,#16784,#16785,#16786));
#4081=EDGE_LOOP('',(#16787,#16788,#16789,#16790,#16791));
#4082=EDGE_LOOP('',(#16792,#16793,#16794,#16795,#16796));
#4083=EDGE_LOOP('',(#16797,#16798,#16799,#16800,#16801));
#4084=EDGE_LOOP('',(#16802,#16803,#16804,#16805,#16806));
#4085=EDGE_LOOP('',(#16807,#16808,#16809,#16810,#16811));
#4086=EDGE_LOOP('',(#16812,#16813,#16814,#16815,#16816));
#4087=EDGE_LOOP('',(#16817,#16818,#16819,#16820,#16821));
#4088=EDGE_LOOP('',(#16822,#16823,#16824,#16825,#16826,#16827));
#4089=EDGE_LOOP('',(#16828,#16829,#16830,#16831,#16832,#16833));
#4090=EDGE_LOOP('',(#16834,#16835,#16836,#16837,#16838,#16839));
#4091=EDGE_LOOP('',(#16840,#16841,#16842,#16843,#16844,#16845));
#4092=EDGE_LOOP('',(#16846,#16847,#16848,#16849,#16850,#16851));
#4093=EDGE_LOOP('',(#16852,#16853,#16854,#16855,#16856,#16857));
#4094=EDGE_LOOP('',(#16858,#16859,#16860,#16861,#16862,#16863));
#4095=EDGE_LOOP('',(#16864,#16865,#16866,#16867,#16868,#16869));
#4096=EDGE_LOOP('',(#16870,#16871,#16872,#16873,#16874,#16875));
#4097=EDGE_LOOP('',(#16876,#16877,#16878,#16879,#16880,#16881));
#4098=EDGE_LOOP('',(#16882,#16883,#16884,#16885,#16886,#16887));
#4099=EDGE_LOOP('',(#16888,#16889,#16890,#16891,#16892,#16893));
#4100=EDGE_LOOP('',(#16894,#16895,#16896,#16897,#16898,#16899));
#4101=EDGE_LOOP('',(#16900,#16901,#16902,#16903,#16904,#16905));
#4102=EDGE_LOOP('',(#16906,#16907,#16908,#16909,#16910,#16911));
#4103=EDGE_LOOP('',(#16912,#16913,#16914,#16915,#16916,#16917));
#4104=EDGE_LOOP('',(#16918,#16919,#16920,#16921,#16922,#16923));
#4105=EDGE_LOOP('',(#16924,#16925,#16926,#16927,#16928,#16929));
#4106=EDGE_LOOP('',(#16930));
#4107=EDGE_LOOP('',(#16931));
#4108=EDGE_LOOP('',(#16932));
#4109=EDGE_LOOP('',(#16933));
#4110=EDGE_LOOP('',(#16934));
#4111=EDGE_LOOP('',(#16935));
#4112=EDGE_LOOP('',(#16936));
#4113=EDGE_LOOP('',(#16937));
#4114=EDGE_LOOP('',(#16938,#16939,#16940,#16941));
#4115=EDGE_LOOP('',(#16942,#16943,#16944,#16945));
#4116=EDGE_LOOP('',(#16946,#16947,#16948,#16949));
#4117=EDGE_LOOP('',(#16950,#16951,#16952,#16953));
#4118=EDGE_LOOP('',(#16954,#16955,#16956,#16957,#16958));
#4119=EDGE_LOOP('',(#16959,#16960,#16961,#16962));
#4120=EDGE_LOOP('',(#16963,#16964,#16965,#16966));
#4121=EDGE_LOOP('',(#16967,#16968,#16969,#16970));
#4122=EDGE_LOOP('',(#16971,#16972,#16973,#16974,#16975,#16976));
#4123=EDGE_LOOP('',(#16977,#16978,#16979,#16980));
#4124=EDGE_LOOP('',(#16981,#16982,#16983,#16984));
#4125=EDGE_LOOP('',(#16985,#16986,#16987,#16988));
#4126=EDGE_LOOP('',(#16989,#16990,#16991,#16992));
#4127=EDGE_LOOP('',(#16993,#16994,#16995,#16996));
#4128=EDGE_LOOP('',(#16997,#16998,#16999,#17000,#17001,#17002));
#4129=EDGE_LOOP('',(#17003,#17004,#17005,#17006));
#4130=EDGE_LOOP('',(#17007,#17008,#17009,#17010));
#4131=EDGE_LOOP('',(#17011,#17012,#17013,#17014));
#4132=EDGE_LOOP('',(#17015,#17016,#17017,#17018));
#4133=EDGE_LOOP('',(#17019,#17020,#17021,#17022));
#4134=EDGE_LOOP('',(#17023,#17024,#17025,#17026));
#4135=EDGE_LOOP('',(#17027,#17028,#17029,#17030,#17031,#17032));
#4136=EDGE_LOOP('',(#17033,#17034,#17035,#17036));
#4137=EDGE_LOOP('',(#17037,#17038,#17039,#17040));
#4138=EDGE_LOOP('',(#17041,#17042,#17043,#17044));
#4139=EDGE_LOOP('',(#17045,#17046,#17047,#17048));
#4140=EDGE_LOOP('',(#17049,#17050,#17051,#17052));
#4141=EDGE_LOOP('',(#17053,#17054,#17055,#17056,#17057,#17058));
#4142=EDGE_LOOP('',(#17059,#17060,#17061,#17062));
#4143=EDGE_LOOP('',(#17063,#17064,#17065,#17066));
#4144=EDGE_LOOP('',(#17067,#17068,#17069,#17070));
#4145=EDGE_LOOP('',(#17071,#17072,#17073,#17074));
#4146=EDGE_LOOP('',(#17075,#17076,#17077,#17078));
#4147=EDGE_LOOP('',(#17079,#17080,#17081,#17082,#17083));
#4148=EDGE_LOOP('',(#17084,#17085,#17086,#17087));
#4149=EDGE_LOOP('',(#17088,#17089,#17090,#17091));
#4150=EDGE_LOOP('',(#17092,#17093,#17094,#17095));
#4151=EDGE_LOOP('',(#17096,#17097,#17098,#17099));
#4152=EDGE_LOOP('',(#17100,#17101,#17102,#17103));
#4153=EDGE_LOOP('',(#17104,#17105,#17106,#17107,#17108,#17109));
#4154=EDGE_LOOP('',(#17110,#17111,#17112,#17113));
#4155=EDGE_LOOP('',(#17114,#17115,#17116,#17117));
#4156=EDGE_LOOP('',(#17118,#17119,#17120,#17121));
#4157=EDGE_LOOP('',(#17122,#17123,#17124,#17125));
#4158=EDGE_LOOP('',(#17126,#17127,#17128,#17129));
#4159=EDGE_LOOP('',(#17130,#17131,#17132,#17133,#17134,#17135));
#4160=EDGE_LOOP('',(#17136,#17137,#17138,#17139));
#4161=EDGE_LOOP('',(#17140,#17141,#17142,#17143));
#4162=EDGE_LOOP('',(#17144,#17145,#17146,#17147));
#4163=EDGE_LOOP('',(#17148,#17149,#17150,#17151,#17152));
#4164=EDGE_LOOP('',(#17153,#17154,#17155,#17156));
#4165=EDGE_LOOP('',(#17157,#17158,#17159,#17160));
#4166=EDGE_LOOP('',(#17161,#17162,#17163,#17164));
#4167=EDGE_LOOP('',(#17165,#17166,#17167,#17168));
#4168=EDGE_LOOP('',(#17169,#17170,#17171,#17172));
#4169=EDGE_LOOP('',(#17173,#17174,#17175,#17176));
#4170=EDGE_LOOP('',(#17177,#17178,#17179,#17180,#17181,#17182));
#4171=EDGE_LOOP('',(#17183,#17184,#17185,#17186));
#4172=EDGE_LOOP('',(#17187,#17188,#17189,#17190));
#4173=EDGE_LOOP('',(#17191,#17192,#17193,#17194));
#4174=EDGE_LOOP('',(#17195,#17196,#17197,#17198));
#4175=EDGE_LOOP('',(#17199,#17200,#17201,#17202));
#4176=EDGE_LOOP('',(#17203,#17204,#17205,#17206,#17207,#17208));
#4177=EDGE_LOOP('',(#17209,#17210,#17211,#17212));
#4178=EDGE_LOOP('',(#17213,#17214,#17215,#17216));
#4179=EDGE_LOOP('',(#17217,#17218,#17219,#17220));
#4180=EDGE_LOOP('',(#17221,#17222,#17223,#17224));
#4181=EDGE_LOOP('',(#17225,#17226,#17227,#17228));
#4182=EDGE_LOOP('',(#17229,#17230,#17231,#17232,#17233));
#4183=EDGE_LOOP('',(#17234,#17235,#17236,#17237));
#4184=EDGE_LOOP('',(#17238,#17239,#17240,#17241));
#4185=EDGE_LOOP('',(#17242,#17243,#17244,#17245));
#4186=EDGE_LOOP('',(#17246,#17247,#17248,#17249));
#4187=EDGE_LOOP('',(#17250,#17251,#17252,#17253));
#4188=EDGE_LOOP('',(#17254,#17255,#17256,#17257,#17258,#17259));
#4189=EDGE_LOOP('',(#17260,#17261,#17262,#17263));
#4190=EDGE_LOOP('',(#17264,#17265,#17266,#17267));
#4191=EDGE_LOOP('',(#17268,#17269,#17270,#17271));
#4192=EDGE_LOOP('',(#17272,#17273,#17274,#17275));
#4193=EDGE_LOOP('',(#17276,#17277,#17278,#17279));
#4194=EDGE_LOOP('',(#17280,#17281,#17282,#17283,#17284,#17285));
#4195=EDGE_LOOP('',(#17286,#17287,#17288,#17289));
#4196=EDGE_LOOP('',(#17290,#17291,#17292,#17293));
#4197=EDGE_LOOP('',(#17294,#17295,#17296,#17297));
#4198=EDGE_LOOP('',(#17298,#17299,#17300,#17301));
#4199=EDGE_LOOP('',(#17302,#17303,#17304,#17305));
#4200=EDGE_LOOP('',(#17306,#17307,#17308,#17309,#17310,#17311));
#4201=EDGE_LOOP('',(#17312,#17313,#17314,#17315));
#4202=EDGE_LOOP('',(#17316,#17317,#17318,#17319));
#4203=EDGE_LOOP('',(#17320,#17321,#17322,#17323));
#4204=EDGE_LOOP('',(#17324,#17325,#17326,#17327));
#4205=EDGE_LOOP('',(#17328,#17329,#17330,#17331));
#4206=EDGE_LOOP('',(#17332,#17333,#17334,#17335));
#4207=EDGE_LOOP('',(#17336,#17337,#17338,#17339,#17340,#17341));
#4208=EDGE_LOOP('',(#17342,#17343,#17344,#17345));
#4209=EDGE_LOOP('',(#17346,#17347,#17348,#17349));
#4210=EDGE_LOOP('',(#17350,#17351,#17352,#17353));
#4211=EDGE_LOOP('',(#17354,#17355,#17356,#17357));
#4212=EDGE_LOOP('',(#17358,#17359,#17360,#17361));
#4213=EDGE_LOOP('',(#17362,#17363,#17364,#17365,#17366,#17367));
#4214=EDGE_LOOP('',(#17368,#17369,#17370,#17371));
#4215=EDGE_LOOP('',(#17372,#17373,#17374,#17375));
#4216=EDGE_LOOP('',(#17376,#17377,#17378,#17379));
#4217=EDGE_LOOP('',(#17380,#17381,#17382,#17383,#17384));
#4218=EDGE_LOOP('',(#17385,#17386,#17387,#17388));
#4219=EDGE_LOOP('',(#17389,#17390,#17391,#17392));
#4220=EDGE_LOOP('',(#17393,#17394,#17395,#17396));
#4221=EDGE_LOOP('',(#17397,#17398,#17399,#17400));
#4222=EDGE_LOOP('',(#17401,#17402,#17403,#17404));
#4223=EDGE_LOOP('',(#17405,#17406,#17407,#17408));
#4224=EDGE_LOOP('',(#17409,#17410,#17411,#17412,#17413,#17414));
#4225=EDGE_LOOP('',(#17415,#17416,#17417,#17418));
#4226=EDGE_LOOP('',(#17419,#17420,#17421,#17422));
#4227=EDGE_LOOP('',(#17423,#17424,#17425,#17426));
#4228=EDGE_LOOP('',(#17427,#17428,#17429,#17430));
#4229=EDGE_LOOP('',(#17431,#17432,#17433,#17434));
#4230=EDGE_LOOP('',(#17435,#17436,#17437,#17438,#17439,#17440));
#4231=EDGE_LOOP('',(#17441,#17442,#17443,#17444));
#4232=EDGE_LOOP('',(#17445,#17446,#17447,#17448));
#4233=EDGE_LOOP('',(#17449,#17450,#17451,#17452));
#4234=EDGE_LOOP('',(#17453,#17454,#17455,#17456));
#4235=EDGE_LOOP('',(#17457,#17458,#17459,#17460,#17461));
#4236=EDGE_LOOP('',(#17462,#17463,#17464,#17465));
#4237=EDGE_LOOP('',(#17466,#17467,#17468,#17469));
#4238=EDGE_LOOP('',(#17470,#17471,#17472,#17473));
#4239=EDGE_LOOP('',(#17474,#17475,#17476,#17477));
#4240=EDGE_LOOP('',(#17478,#17479,#17480,#17481,#17482,#17483));
#4241=EDGE_LOOP('',(#17484,#17485,#17486,#17487));
#4242=EDGE_LOOP('',(#17488,#17489,#17490,#17491));
#4243=EDGE_LOOP('',(#17492,#17493,#17494,#17495));
#4244=EDGE_LOOP('',(#17496,#17497,#17498,#17499));
#4245=EDGE_LOOP('',(#17500,#17501,#17502,#17503));
#4246=EDGE_LOOP('',(#17504,#17505,#17506,#17507,#17508,#17509));
#4247=EDGE_LOOP('',(#17510,#17511,#17512,#17513));
#4248=EDGE_LOOP('',(#17514,#17515,#17516,#17517));
#4249=EDGE_LOOP('',(#17518,#17519,#17520,#17521));
#4250=EDGE_LOOP('',(#17522,#17523,#17524,#17525));
#4251=EDGE_LOOP('',(#17526,#17527,#17528,#17529));
#4252=EDGE_LOOP('',(#17530,#17531,#17532,#17533,#17534,#17535));
#4253=EDGE_LOOP('',(#17536,#17537,#17538,#17539));
#4254=EDGE_LOOP('',(#17540,#17541,#17542,#17543));
#4255=EDGE_LOOP('',(#17544,#17545,#17546,#17547));
#4256=EDGE_LOOP('',(#17548,#17549,#17550,#17551,#17552));
#4257=EDGE_LOOP('',(#17553,#17554,#17555,#17556));
#4258=EDGE_LOOP('',(#17557,#17558,#17559,#17560));
#4259=EDGE_LOOP('',(#17561,#17562,#17563,#17564));
#4260=EDGE_LOOP('',(#17565,#17566,#17567,#17568));
#4261=EDGE_LOOP('',(#17569,#17570,#17571,#17572,#17573));
#4262=EDGE_LOOP('',(#17574,#17575,#17576,#17577));
#4263=EDGE_LOOP('',(#17578,#17579,#17580,#17581,#17582));
#4264=EDGE_LOOP('',(#17583,#17584,#17585,#17586));
#4265=EDGE_LOOP('',(#17587,#17588,#17589,#17590));
#4266=EDGE_LOOP('',(#17591,#17592,#17593,#17594,#17595));
#4267=EDGE_LOOP('',(#17596,#17597,#17598,#17599));
#4268=EDGE_LOOP('',(#17600,#17601,#17602,#17603,#17604));
#4269=EDGE_LOOP('',(#17605,#17606,#17607,#17608));
#4270=EDGE_LOOP('',(#17609,#17610,#17611,#17612));
#4271=EDGE_LOOP('',(#17613,#17614,#17615,#17616,#17617));
#4272=EDGE_LOOP('',(#17618,#17619,#17620,#17621));
#4273=EDGE_LOOP('',(#17622,#17623,#17624,#17625));
#4274=EDGE_LOOP('',(#17626,#17627,#17628,#17629));
#4275=EDGE_LOOP('',(#17630,#17631,#17632,#17633));
#4276=EDGE_LOOP('',(#17634,#17635,#17636,#17637));
#4277=EDGE_LOOP('',(#17638,#17639,#17640,#17641));
#4278=EDGE_LOOP('',(#17642,#17643,#17644,#17645));
#4279=EDGE_LOOP('',(#17646,#17647,#17648,#17649));
#4280=EDGE_LOOP('',(#17650,#17651,#17652,#17653));
#4281=EDGE_LOOP('',(#17654,#17655,#17656,#17657));
#4282=EDGE_LOOP('',(#17658,#17659,#17660,#17661));
#4283=EDGE_LOOP('',(#17662,#17663,#17664,#17665));
#4284=EDGE_LOOP('',(#17666,#17667,#17668,#17669));
#4285=EDGE_LOOP('',(#17670,#17671,#17672,#17673));
#4286=EDGE_LOOP('',(#17674,#17675,#17676,#17677));
#4287=EDGE_LOOP('',(#17678,#17679,#17680,#17681));
#4288=EDGE_LOOP('',(#17682,#17683,#17684,#17685));
#4289=EDGE_LOOP('',(#17686,#17687,#17688,#17689));
#4290=EDGE_LOOP('',(#17690,#17691,#17692,#17693));
#4291=EDGE_LOOP('',(#17694,#17695,#17696,#17697));
#4292=EDGE_LOOP('',(#17698,#17699,#17700,#17701));
#4293=EDGE_LOOP('',(#17702,#17703,#17704,#17705));
#4294=EDGE_LOOP('',(#17706,#17707,#17708,#17709));
#4295=EDGE_LOOP('',(#17710,#17711,#17712,#17713));
#4296=EDGE_LOOP('',(#17714,#17715,#17716,#17717));
#4297=EDGE_LOOP('',(#17718,#17719,#17720,#17721));
#4298=EDGE_LOOP('',(#17722,#17723,#17724,#17725));
#4299=EDGE_LOOP('',(#17726,#17727,#17728,#17729));
#4300=EDGE_LOOP('',(#17730,#17731,#17732,#17733));
#4301=EDGE_LOOP('',(#17734,#17735,#17736,#17737));
#4302=EDGE_LOOP('',(#17738,#17739,#17740,#17741));
#4303=EDGE_LOOP('',(#17742,#17743,#17744,#17745));
#4304=EDGE_LOOP('',(#17746,#17747,#17748,#17749));
#4305=EDGE_LOOP('',(#17750,#17751,#17752,#17753));
#4306=EDGE_LOOP('',(#17754,#17755,#17756,#17757));
#4307=EDGE_LOOP('',(#17758,#17759,#17760,#17761));
#4308=EDGE_LOOP('',(#17762,#17763,#17764,#17765));
#4309=EDGE_LOOP('',(#17766,#17767,#17768,#17769));
#4310=EDGE_LOOP('',(#17770,#17771,#17772,#17773));
#4311=EDGE_LOOP('',(#17774,#17775,#17776,#17777));
#4312=EDGE_LOOP('',(#17778,#17779,#17780,#17781));
#4313=EDGE_LOOP('',(#17782));
#4314=EDGE_LOOP('',(#17783));
#4315=EDGE_LOOP('',(#17784,#17785,#17786,#17787));
#4316=EDGE_LOOP('',(#17788,#17789,#17790,#17791));
#5499=LINE('',#34454,#7320);
#5500=LINE('',#34458,#7321);
#5501=LINE('',#34462,#7322);
#5502=LINE('',#34467,#7323);
#5503=LINE('',#34471,#7324);
#5504=LINE('',#34475,#7325);
#5505=LINE('',#34480,#7326);
#5506=LINE('',#34484,#7327);
#5507=LINE('',#34488,#7328);
#5508=LINE('',#34493,#7329);
#5509=LINE('',#34497,#7330);
#5510=LINE('',#34501,#7331);
#5511=LINE('',#34506,#7332);
#5512=LINE('',#34510,#7333);
#5513=LINE('',#34514,#7334);
#5514=LINE('',#34520,#7335);
#5515=LINE('',#34524,#7336);
#5516=LINE('',#34528,#7337);
#5517=LINE('',#34535,#7338);
#5518=LINE('',#34541,#7339);
#5519=LINE('',#34545,#7340);
#5520=LINE('',#34549,#7341);
#5521=LINE('',#34556,#7342);
#5522=LINE('',#34562,#7343);
#5523=LINE('',#34566,#7344);
#5524=LINE('',#34570,#7345);
#5525=LINE('',#34577,#7346);
#5526=LINE('',#34583,#7347);
#5527=LINE('',#34587,#7348);
#5528=LINE('',#34591,#7349);
#5529=LINE('',#34598,#7350);
#5530=LINE('',#34604,#7351);
#5531=LINE('',#34608,#7352);
#5532=LINE('',#34612,#7353);
#5533=LINE('',#34619,#7354);
#5534=LINE('',#34625,#7355);
#5535=LINE('',#34629,#7356);
#5536=LINE('',#34633,#7357);
#5537=LINE('',#34640,#7358);
#5538=LINE('',#34646,#7359);
#5539=LINE('',#34650,#7360);
#5540=LINE('',#34654,#7361);
#5541=LINE('',#34661,#7362);
#5542=LINE('',#34667,#7363);
#5543=LINE('',#34671,#7364);
#5544=LINE('',#34675,#7365);
#5545=LINE('',#34682,#7366);
#5546=LINE('',#34688,#7367);
#5547=LINE('',#34692,#7368);
#5548=LINE('',#34696,#7369);
#5549=LINE('',#34703,#7370);
#5550=LINE('',#34709,#7371);
#5551=LINE('',#34713,#7372);
#5552=LINE('',#34717,#7373);
#5553=LINE('',#34724,#7374);
#5554=LINE('',#34730,#7375);
#5555=LINE('',#34734,#7376);
#5556=LINE('',#34738,#7377);
#5557=LINE('',#34745,#7378);
#5558=LINE('',#34751,#7379);
#5559=LINE('',#34755,#7380);
#5560=LINE('',#34759,#7381);
#5561=LINE('',#34766,#7382);
#5562=LINE('',#34772,#7383);
#5563=LINE('',#34781,#7384);
#5564=LINE('',#34787,#7385);
#5565=LINE('',#34798,#7386);
#5566=LINE('',#34805,#7387);
#5567=LINE('',#34812,#7388);
#5568=LINE('',#34816,#7389);
#5569=LINE('',#34820,#7390);
#5570=LINE('',#34828,#7391);
#5571=LINE('',#34832,#7392);
#5572=LINE('',#34836,#7393);
#5573=LINE('',#34840,#7394);
#5574=LINE('',#34850,#7395);
#5575=LINE('',#34853,#7396);
#5576=LINE('',#34856,#7397);
#5577=LINE('',#34860,#7398);
#5578=LINE('',#34868,#7399);
#5579=LINE('',#34872,#7400);
#5580=LINE('',#34876,#7401);
#5581=LINE('',#34880,#7402);
#5582=LINE('',#34890,#7403);
#5583=LINE('',#34893,#7404);
#5584=LINE('',#34896,#7405);
#5585=LINE('',#34900,#7406);
#5586=LINE('',#34908,#7407);
#5587=LINE('',#34912,#7408);
#5588=LINE('',#34916,#7409);
#5589=LINE('',#34920,#7410);
#5590=LINE('',#34930,#7411);
#5591=LINE('',#34933,#7412);
#5592=LINE('',#34936,#7413);
#5593=LINE('',#34940,#7414);
#5594=LINE('',#34944,#7415);
#5595=LINE('',#34948,#7416);
#5596=LINE('',#34952,#7417);
#5597=LINE('',#34956,#7418);
#5598=LINE('',#34960,#7419);
#5599=LINE('',#34964,#7420);
#5600=LINE('',#34968,#7421);
#5601=LINE('',#34972,#7422);
#5602=LINE('',#34976,#7423);
#5603=LINE('',#34980,#7424);
#5604=LINE('',#34984,#7425);
#5605=LINE('',#34988,#7426);
#5606=LINE('',#34992,#7427);
#5607=LINE('',#34996,#7428);
#5608=LINE('',#35000,#7429);
#5609=LINE('',#35004,#7430);
#5610=LINE('',#35008,#7431);
#5611=LINE('',#35012,#7432);
#5612=LINE('',#35016,#7433);
#5613=LINE('',#35020,#7434);
#5614=LINE('',#35024,#7435);
#5615=LINE('',#35028,#7436);
#5616=LINE('',#35032,#7437);
#5617=LINE('',#35036,#7438);
#5618=LINE('',#35040,#7439);
#5619=LINE('',#35044,#7440);
#5620=LINE('',#35048,#7441);
#5621=LINE('',#35052,#7442);
#5622=LINE('',#35056,#7443);
#5623=LINE('',#35060,#7444);
#5624=LINE('',#35064,#7445);
#5625=LINE('',#35068,#7446);
#5626=LINE('',#35072,#7447);
#5627=LINE('',#35076,#7448);
#5628=LINE('',#35080,#7449);
#5629=LINE('',#35084,#7450);
#5630=LINE('',#35088,#7451);
#5631=LINE('',#35092,#7452);
#5632=LINE('',#35096,#7453);
#5633=LINE('',#35100,#7454);
#5634=LINE('',#35104,#7455);
#5635=LINE('',#35108,#7456);
#5636=LINE('',#35112,#7457);
#5637=LINE('',#35116,#7458);
#5638=LINE('',#35120,#7459);
#5639=LINE('',#35124,#7460);
#5640=LINE('',#35128,#7461);
#5641=LINE('',#35132,#7462);
#5642=LINE('',#35136,#7463);
#5643=LINE('',#35140,#7464);
#5644=LINE('',#35144,#7465);
#5645=LINE('',#35148,#7466);
#5646=LINE('',#35154,#7467);
#5647=LINE('',#35157,#7468);
#5648=LINE('',#35162,#7469);
#5649=LINE('',#35163,#7470);
#5650=LINE('',#35166,#7471);
#5651=LINE('',#35167,#7472);
#5652=LINE('',#35172,#7473);
#5653=LINE('',#35173,#7474);
#5654=LINE('',#35175,#7475);
#5655=LINE('',#35181,#7476);
#5656=LINE('',#35182,#7477);
#5657=LINE('',#35185,#7478);
#5658=LINE('',#35186,#7479);
#5659=LINE('',#35191,#7480);
#5660=LINE('',#35192,#7481);
#5661=LINE('',#35194,#7482);
#5662=LINE('',#35196,#7483);
#5663=LINE('',#35199,#7484);
#5664=LINE('',#35205,#7485);
#5665=LINE('',#35206,#7486);
#5666=LINE('',#35209,#7487);
#5667=LINE('',#35210,#7488);
#5668=LINE('',#35215,#7489);
#5669=LINE('',#35216,#7490);
#5670=LINE('',#35218,#7491);
#5671=LINE('',#35220,#7492);
#5672=LINE('',#35223,#7493);
#5673=LINE('',#35227,#7494);
#5674=LINE('',#35230,#7495);
#5675=LINE('',#35235,#7496);
#5676=LINE('',#35236,#7497);
#5677=LINE('',#35239,#7498);
#5678=LINE('',#35240,#7499);
#5679=LINE('',#35245,#7500);
#5680=LINE('',#35246,#7501);
#5681=LINE('',#35248,#7502);
#5682=LINE('',#35250,#7503);
#5683=LINE('',#35253,#7504);
#5684=LINE('',#35259,#7505);
#5685=LINE('',#35260,#7506);
#5686=LINE('',#35263,#7507);
#5687=LINE('',#35264,#7508);
#5688=LINE('',#35269,#7509);
#5689=LINE('',#35270,#7510);
#5690=LINE('',#35272,#7511);
#5691=LINE('',#35274,#7512);
#5692=LINE('',#35277,#7513);
#5693=LINE('',#35283,#7514);
#5694=LINE('',#35284,#7515);
#5695=LINE('',#35287,#7516);
#5696=LINE('',#35288,#7517);
#5697=LINE('',#35293,#7518);
#5698=LINE('',#35294,#7519);
#5699=LINE('',#35297,#7520);
#5700=LINE('',#35302,#7521);
#5701=LINE('',#35304,#7522);
#5702=LINE('',#35306,#7523);
#5703=LINE('',#35311,#7524);
#5704=LINE('',#35312,#7525);
#5705=LINE('',#35315,#7526);
#5706=LINE('',#35316,#7527);
#5707=LINE('',#35321,#7528);
#5708=LINE('',#35322,#7529);
#5709=LINE('',#35324,#7530);
#5710=LINE('',#35326,#7531);
#5711=LINE('',#35329,#7532);
#5712=LINE('',#35335,#7533);
#5713=LINE('',#35336,#7534);
#5714=LINE('',#35339,#7535);
#5715=LINE('',#35340,#7536);
#5716=LINE('',#35345,#7537);
#5717=LINE('',#35346,#7538);
#5718=LINE('',#35348,#7539);
#5719=LINE('',#35350,#7540);
#5720=LINE('',#35353,#7541);
#5721=LINE('',#35357,#7542);
#5722=LINE('',#35360,#7543);
#5723=LINE('',#35363,#7544);
#5724=LINE('',#35367,#7545);
#5725=LINE('',#35370,#7546);
#5726=LINE('',#35372,#7547);
#5727=LINE('',#35374,#7548);
#5728=LINE('',#35379,#7549);
#5729=LINE('',#35380,#7550);
#5730=LINE('',#35383,#7551);
#5731=LINE('',#35384,#7552);
#5732=LINE('',#35389,#7553);
#5733=LINE('',#35390,#7554);
#5734=LINE('',#35392,#7555);
#5735=LINE('',#35394,#7556);
#5736=LINE('',#35397,#7557);
#5737=LINE('',#35403,#7558);
#5738=LINE('',#35404,#7559);
#5739=LINE('',#35407,#7560);
#5740=LINE('',#35408,#7561);
#5741=LINE('',#35413,#7562);
#5742=LINE('',#35414,#7563);
#5743=LINE('',#35416,#7564);
#5744=LINE('',#35418,#7565);
#5745=LINE('',#35421,#7566);
#5746=LINE('',#35427,#7567);
#5747=LINE('',#35428,#7568);
#5748=LINE('',#35431,#7569);
#5749=LINE('',#35432,#7570);
#5750=LINE('',#35437,#7571);
#5751=LINE('',#35438,#7572);
#5752=LINE('',#35441,#7573);
#5753=LINE('',#35446,#7574);
#5754=LINE('',#35448,#7575);
#5755=LINE('',#35450,#7576);
#5756=LINE('',#35455,#7577);
#5757=LINE('',#35456,#7578);
#5758=LINE('',#35459,#7579);
#5759=LINE('',#35460,#7580);
#5760=LINE('',#35465,#7581);
#5761=LINE('',#35466,#7582);
#5762=LINE('',#35468,#7583);
#5763=LINE('',#35470,#7584);
#5764=LINE('',#35473,#7585);
#5765=LINE('',#35479,#7586);
#5766=LINE('',#35480,#7587);
#5767=LINE('',#35483,#7588);
#5768=LINE('',#35484,#7589);
#5769=LINE('',#35489,#7590);
#5770=LINE('',#35490,#7591);
#5771=LINE('',#35492,#7592);
#5772=LINE('',#35494,#7593);
#5773=LINE('',#35497,#7594);
#5774=LINE('',#35503,#7595);
#5775=LINE('',#35504,#7596);
#5776=LINE('',#35507,#7597);
#5777=LINE('',#35508,#7598);
#5778=LINE('',#35513,#7599);
#5779=LINE('',#35514,#7600);
#5780=LINE('',#35516,#7601);
#5781=LINE('',#35518,#7602);
#5782=LINE('',#35521,#7603);
#5783=LINE('',#35525,#7604);
#5784=LINE('',#35528,#7605);
#5785=LINE('',#35533,#7606);
#5786=LINE('',#35534,#7607);
#5787=LINE('',#35537,#7608);
#5788=LINE('',#35538,#7609);
#5789=LINE('',#35543,#7610);
#5790=LINE('',#35544,#7611);
#5791=LINE('',#35546,#7612);
#5792=LINE('',#35548,#7613);
#5793=LINE('',#35551,#7614);
#5794=LINE('',#35557,#7615);
#5795=LINE('',#35558,#7616);
#5796=LINE('',#35561,#7617);
#5797=LINE('',#35562,#7618);
#5798=LINE('',#35567,#7619);
#5799=LINE('',#35568,#7620);
#5800=LINE('',#35570,#7621);
#5801=LINE('',#35572,#7622);
#5802=LINE('',#35575,#7623);
#5803=LINE('',#35579,#7624);
#5804=LINE('',#35582,#7625);
#5805=LINE('',#35585,#7626);
#5806=LINE('',#35589,#7627);
#5807=LINE('',#35592,#7628);
#5808=LINE('',#35594,#7629);
#5809=LINE('',#35596,#7630);
#5810=LINE('',#35601,#7631);
#5811=LINE('',#35602,#7632);
#5812=LINE('',#35605,#7633);
#5813=LINE('',#35606,#7634);
#5814=LINE('',#35611,#7635);
#5815=LINE('',#35612,#7636);
#5816=LINE('',#35614,#7637);
#5817=LINE('',#35616,#7638);
#5818=LINE('',#35619,#7639);
#5819=LINE('',#35625,#7640);
#5820=LINE('',#35626,#7641);
#5821=LINE('',#35629,#7642);
#5822=LINE('',#35630,#7643);
#5823=LINE('',#35635,#7644);
#5824=LINE('',#35636,#7645);
#5825=LINE('',#35638,#7646);
#5826=LINE('',#35640,#7647);
#5827=LINE('',#35643,#7648);
#5828=LINE('',#35647,#7649);
#5829=LINE('',#35650,#7650);
#5830=LINE('',#35655,#7651);
#5831=LINE('',#35656,#7652);
#5832=LINE('',#35658,#7653);
#5833=LINE('',#35660,#7654);
#5834=LINE('',#35663,#7655);
#5835=LINE('',#35668,#7656);
#5836=LINE('',#35669,#7657);
#5837=LINE('',#35672,#7658);
#5838=LINE('',#35673,#7659);
#5839=LINE('',#35678,#7660);
#5840=LINE('',#35679,#7661);
#5841=LINE('',#35681,#7662);
#5842=LINE('',#35683,#7663);
#5843=LINE('',#35686,#7664);
#5844=LINE('',#35692,#7665);
#5845=LINE('',#35693,#7666);
#5846=LINE('',#35696,#7667);
#5847=LINE('',#35697,#7668);
#5848=LINE('',#35702,#7669);
#5849=LINE('',#35703,#7670);
#5850=LINE('',#35705,#7671);
#5851=LINE('',#35707,#7672);
#5852=LINE('',#35710,#7673);
#5853=LINE('',#35716,#7674);
#5854=LINE('',#35717,#7675);
#5855=LINE('',#35720,#7676);
#5856=LINE('',#35721,#7677);
#5857=LINE('',#35726,#7678);
#5858=LINE('',#35727,#7679);
#5859=LINE('',#35729,#7680);
#5860=LINE('',#35731,#7681);
#5861=LINE('',#35734,#7682);
#5862=LINE('',#35740,#7683);
#5863=LINE('',#35741,#7684);
#5864=LINE('',#35743,#7685);
#5865=LINE('',#35745,#7686);
#5866=LINE('',#35748,#7687);
#5867=LINE('',#35753,#7688);
#5868=LINE('',#35754,#7689);
#5869=LINE('',#35757,#7690);
#5870=LINE('',#35758,#7691);
#5871=LINE('',#35763,#7692);
#5872=LINE('',#35764,#7693);
#5873=LINE('',#35766,#7694);
#5874=LINE('',#35772,#7695);
#5875=LINE('',#35773,#7696);
#5876=LINE('',#35775,#7697);
#5877=LINE('',#35777,#7698);
#5878=LINE('',#35780,#7699);
#5879=LINE('',#35785,#7700);
#5880=LINE('',#35786,#7701);
#5881=LINE('',#35788,#7702);
#5882=LINE('',#35794,#7703);
#5883=LINE('',#35795,#7704);
#5884=LINE('',#35797,#7705);
#5885=LINE('',#35799,#7706);
#5886=LINE('',#35802,#7707);
#5887=LINE('',#35807,#7708);
#5888=LINE('',#35808,#7709);
#5889=LINE('',#35810,#7710);
#5890=LINE('',#35818,#7711);
#5891=LINE('',#35823,#7712);
#5892=LINE('',#35856,#7713);
#5893=LINE('',#35862,#7714);
#5894=LINE('',#35864,#7715);
#7320=VECTOR('',#27895,0.0525);
#7321=VECTOR('',#27900,0.105);
#7322=VECTOR('',#27905,0.155);
#7323=VECTOR('',#27910,0.0525);
#7324=VECTOR('',#27915,0.105);
#7325=VECTOR('',#27920,0.155);
#7326=VECTOR('',#27925,0.0650000000000004);
#7327=VECTOR('',#27930,0.13);
#7328=VECTOR('',#27935,0.180000000000001);
#7329=VECTOR('',#27940,0.0649999999999999);
#7330=VECTOR('',#27945,0.13);
#7331=VECTOR('',#27950,0.18);
#7332=VECTOR('',#27955,0.065);
#7333=VECTOR('',#27960,0.13);
#7334=VECTOR('',#27965,0.18);
#7335=VECTOR('',#27972,0.1325);
#7336=VECTOR('',#27977,0.12);
#7337=VECTOR('',#27982,0.1325);
#7338=VECTOR('',#27991,0.21);
#7339=VECTOR('',#27998,0.1325);
#7340=VECTOR('',#28003,0.12);
#7341=VECTOR('',#28008,0.1325);
#7342=VECTOR('',#28017,0.21);
#7343=VECTOR('',#28024,0.1325);
#7344=VECTOR('',#28029,0.12);
#7345=VECTOR('',#28034,0.1325);
#7346=VECTOR('',#28043,0.21);
#7347=VECTOR('',#28050,0.1325);
#7348=VECTOR('',#28055,0.12);
#7349=VECTOR('',#28060,0.1325);
#7350=VECTOR('',#28069,0.21);
#7351=VECTOR('',#28076,0.1325);
#7352=VECTOR('',#28081,0.12);
#7353=VECTOR('',#28086,0.1325);
#7354=VECTOR('',#28095,0.21);
#7355=VECTOR('',#28102,0.1325);
#7356=VECTOR('',#28107,0.120000000000001);
#7357=VECTOR('',#28112,0.1325);
#7358=VECTOR('',#28121,0.21);
#7359=VECTOR('',#28128,0.1325);
#7360=VECTOR('',#28133,0.12);
#7361=VECTOR('',#28138,0.1325);
#7362=VECTOR('',#28147,0.21);
#7363=VECTOR('',#28154,0.132499999999999);
#7364=VECTOR('',#28159,0.12);
#7365=VECTOR('',#28164,0.132499999999999);
#7366=VECTOR('',#28173,0.21);
#7367=VECTOR('',#28180,0.1325);
#7368=VECTOR('',#28185,0.12);
#7369=VECTOR('',#28190,0.1325);
#7370=VECTOR('',#28199,0.21);
#7371=VECTOR('',#28206,0.1325);
#7372=VECTOR('',#28211,0.12);
#7373=VECTOR('',#28216,0.1325);
#7374=VECTOR('',#28225,0.21);
#7375=VECTOR('',#28232,0.1325);
#7376=VECTOR('',#28237,0.12);
#7377=VECTOR('',#28242,0.1325);
#7378=VECTOR('',#28251,0.21);
#7379=VECTOR('',#28258,0.1325);
#7380=VECTOR('',#28263,0.12);
#7381=VECTOR('',#28268,0.1325);
#7382=VECTOR('',#28277,0.21);
#7383=VECTOR('',#28284,0.72);
#7384=VECTOR('',#28295,0.7);
#7385=VECTOR('',#28302,0.72);
#7386=VECTOR('',#28315,4.585);
#7387=VECTOR('',#28324,4.6);
#7388=VECTOR('',#28333,4.585);
#7389=VECTOR('',#28336,1.);
#7390=VECTOR('',#28339,1.);
#7391=VECTOR('',#28346,1.);
#7392=VECTOR('',#28349,1.);
#7393=VECTOR('',#28352,1.);
#7394=VECTOR('',#28355,1.);
#7395=VECTOR('',#28364,1.);
#7396=VECTOR('',#28367,1.);
#7397=VECTOR('',#28368,1.);
#7398=VECTOR('',#28371,1.);
#7399=VECTOR('',#28378,1.);
#7400=VECTOR('',#28381,1.);
#7401=VECTOR('',#28384,1.);
#7402=VECTOR('',#28387,1.);
#7403=VECTOR('',#28396,1.);
#7404=VECTOR('',#28399,1.);
#7405=VECTOR('',#28400,1.);
#7406=VECTOR('',#28403,1.);
#7407=VECTOR('',#28410,1.);
#7408=VECTOR('',#28413,1.);
#7409=VECTOR('',#28416,1.);
#7410=VECTOR('',#28419,1.);
#7411=VECTOR('',#28428,1.);
#7412=VECTOR('',#28431,1.);
#7413=VECTOR('',#28432,1.);
#7414=VECTOR('',#28435,1.);
#7415=VECTOR('',#28438,1.);
#7416=VECTOR('',#28441,1.);
#7417=VECTOR('',#28444,1.);
#7418=VECTOR('',#28447,1.);
#7419=VECTOR('',#28450,1.);
#7420=VECTOR('',#28453,1.);
#7421=VECTOR('',#28456,1.);
#7422=VECTOR('',#28459,1.);
#7423=VECTOR('',#28462,1.);
#7424=VECTOR('',#28465,1.);
#7425=VECTOR('',#28468,1.);
#7426=VECTOR('',#28471,1.);
#7427=VECTOR('',#28474,1.);
#7428=VECTOR('',#28477,1.);
#7429=VECTOR('',#28480,1.);
#7430=VECTOR('',#28483,1.);
#7431=VECTOR('',#28486,1.);
#7432=VECTOR('',#28489,1.);
#7433=VECTOR('',#28492,1.);
#7434=VECTOR('',#28495,1.);
#7435=VECTOR('',#28498,1.);
#7436=VECTOR('',#28501,1.);
#7437=VECTOR('',#28504,1.);
#7438=VECTOR('',#28507,1.);
#7439=VECTOR('',#28510,1.);
#7440=VECTOR('',#28513,1.);
#7441=VECTOR('',#28516,1.);
#7442=VECTOR('',#28519,1.);
#7443=VECTOR('',#28522,1.);
#7444=VECTOR('',#28525,1.);
#7445=VECTOR('',#28528,1.);
#7446=VECTOR('',#28531,1.);
#7447=VECTOR('',#28534,1.);
#7448=VECTOR('',#28537,1.);
#7449=VECTOR('',#28540,1.);
#7450=VECTOR('',#28543,1.);
#7451=VECTOR('',#28546,1.);
#7452=VECTOR('',#28549,1.);
#7453=VECTOR('',#28552,1.);
#7454=VECTOR('',#28555,1.);
#7455=VECTOR('',#28558,1.);
#7456=VECTOR('',#28561,1.);
#7457=VECTOR('',#28564,1.);
#7458=VECTOR('',#28567,1.);
#7459=VECTOR('',#28570,1.);
#7460=VECTOR('',#28573,1.);
#7461=VECTOR('',#28576,1.);
#7462=VECTOR('',#28579,1.);
#7463=VECTOR('',#28582,1.);
#7464=VECTOR('',#28585,1.);
#7465=VECTOR('',#28588,1.);
#7466=VECTOR('',#28591,1.);
#7467=VECTOR('',#28598,0.12);
#7468=VECTOR('',#28601,1.);
#7469=VECTOR('',#28606,1.);
#7470=VECTOR('',#28607,1.);
#7471=VECTOR('',#28610,1.);
#7472=VECTOR('',#28611,1.);
#7473=VECTOR('',#28616,0.12);
#7474=VECTOR('',#28617,1.);
#7475=VECTOR('',#28620,1.);
#7476=VECTOR('',#28627,1.);
#7477=VECTOR('',#28628,1.);
#7478=VECTOR('',#28631,1.);
#7479=VECTOR('',#28632,1.);
#7480=VECTOR('',#28637,1.);
#7481=VECTOR('',#28638,1.);
#7482=VECTOR('',#28641,1.);
#7483=VECTOR('',#28642,1.);
#7484=VECTOR('',#28647,1.);
#7485=VECTOR('',#28654,1.);
#7486=VECTOR('',#28655,1.);
#7487=VECTOR('',#28658,1.);
#7488=VECTOR('',#28659,1.);
#7489=VECTOR('',#28664,1.);
#7490=VECTOR('',#28665,1.);
#7491=VECTOR('',#28668,1.);
#7492=VECTOR('',#28669,1.);
#7493=VECTOR('',#28674,1.);
#7494=VECTOR('',#28679,0.12);
#7495=VECTOR('',#28682,1.);
#7496=VECTOR('',#28687,1.);
#7497=VECTOR('',#28688,1.);
#7498=VECTOR('',#28691,1.);
#7499=VECTOR('',#28692,1.);
#7500=VECTOR('',#28697,1.);
#7501=VECTOR('',#28698,1.);
#7502=VECTOR('',#28701,1.);
#7503=VECTOR('',#28702,1.);
#7504=VECTOR('',#28707,1.);
#7505=VECTOR('',#28714,1.);
#7506=VECTOR('',#28715,1.);
#7507=VECTOR('',#28718,1.);
#7508=VECTOR('',#28719,1.);
#7509=VECTOR('',#28724,1.);
#7510=VECTOR('',#28725,1.);
#7511=VECTOR('',#28728,1.);
#7512=VECTOR('',#28729,1.);
#7513=VECTOR('',#28734,1.);
#7514=VECTOR('',#28741,1.);
#7515=VECTOR('',#28742,1.);
#7516=VECTOR('',#28745,1.);
#7517=VECTOR('',#28746,1.);
#7518=VECTOR('',#28751,1.);
#7519=VECTOR('',#28752,1.);
#7520=VECTOR('',#28755,1.);
#7521=VECTOR('',#28760,1.);
#7522=VECTOR('',#28763,0.12);
#7523=VECTOR('',#28766,1.);
#7524=VECTOR('',#28771,1.);
#7525=VECTOR('',#28772,1.);
#7526=VECTOR('',#28775,1.);
#7527=VECTOR('',#28776,1.);
#7528=VECTOR('',#28781,1.);
#7529=VECTOR('',#28782,1.);
#7530=VECTOR('',#28785,1.);
#7531=VECTOR('',#28786,1.);
#7532=VECTOR('',#28791,1.);
#7533=VECTOR('',#28798,1.);
#7534=VECTOR('',#28799,1.);
#7535=VECTOR('',#28802,1.);
#7536=VECTOR('',#28803,1.);
#7537=VECTOR('',#28808,1.);
#7538=VECTOR('',#28809,1.);
#7539=VECTOR('',#28812,1.);
#7540=VECTOR('',#28813,1.);
#7541=VECTOR('',#28818,1.);
#7542=VECTOR('',#28823,0.12);
#7543=VECTOR('',#28826,1.);
#7544=VECTOR('',#28829,1.);
#7545=VECTOR('',#28832,1.);
#7546=VECTOR('',#28837,1.);
#7547=VECTOR('',#28840,1.);
#7548=VECTOR('',#28843,1.);
#7549=VECTOR('',#28848,1.);
#7550=VECTOR('',#28849,1.);
#7551=VECTOR('',#28852,1.);
#7552=VECTOR('',#28853,1.);
#7553=VECTOR('',#28858,1.);
#7554=VECTOR('',#28859,1.);
#7555=VECTOR('',#28862,1.);
#7556=VECTOR('',#28863,1.);
#7557=VECTOR('',#28868,1.);
#7558=VECTOR('',#28875,1.);
#7559=VECTOR('',#28876,1.);
#7560=VECTOR('',#28879,1.);
#7561=VECTOR('',#28880,1.);
#7562=VECTOR('',#28885,1.);
#7563=VECTOR('',#28886,1.);
#7564=VECTOR('',#28889,1.);
#7565=VECTOR('',#28890,1.);
#7566=VECTOR('',#28895,1.);
#7567=VECTOR('',#28902,1.);
#7568=VECTOR('',#28903,1.);
#7569=VECTOR('',#28906,1.);
#7570=VECTOR('',#28907,1.);
#7571=VECTOR('',#28912,1.);
#7572=VECTOR('',#28913,1.);
#7573=VECTOR('',#28916,1.);
#7574=VECTOR('',#28921,1.);
#7575=VECTOR('',#28924,0.12);
#7576=VECTOR('',#28927,1.);
#7577=VECTOR('',#28932,1.);
#7578=VECTOR('',#28933,1.);
#7579=VECTOR('',#28936,1.);
#7580=VECTOR('',#28937,1.);
#7581=VECTOR('',#28942,1.);
#7582=VECTOR('',#28943,1.);
#7583=VECTOR('',#28946,1.);
#7584=VECTOR('',#28947,1.);
#7585=VECTOR('',#28952,1.);
#7586=VECTOR('',#28959,1.);
#7587=VECTOR('',#28960,1.);
#7588=VECTOR('',#28963,1.);
#7589=VECTOR('',#28964,1.);
#7590=VECTOR('',#28969,1.);
#7591=VECTOR('',#28970,1.);
#7592=VECTOR('',#28973,1.);
#7593=VECTOR('',#28974,1.);
#7594=VECTOR('',#28979,1.);
#7595=VECTOR('',#28986,1.);
#7596=VECTOR('',#28987,1.);
#7597=VECTOR('',#28990,1.);
#7598=VECTOR('',#28991,1.);
#7599=VECTOR('',#28996,1.);
#7600=VECTOR('',#28997,1.);
#7601=VECTOR('',#29000,1.);
#7602=VECTOR('',#29001,1.);
#7603=VECTOR('',#29006,1.);
#7604=VECTOR('',#29011,0.12);
#7605=VECTOR('',#29014,1.);
#7606=VECTOR('',#29019,1.);
#7607=VECTOR('',#29020,1.);
#7608=VECTOR('',#29023,1.);
#7609=VECTOR('',#29024,1.);
#7610=VECTOR('',#29029,1.);
#7611=VECTOR('',#29030,1.);
#7612=VECTOR('',#29033,1.);
#7613=VECTOR('',#29034,1.);
#7614=VECTOR('',#29039,1.);
#7615=VECTOR('',#29046,1.);
#7616=VECTOR('',#29047,1.);
#7617=VECTOR('',#29050,1.);
#7618=VECTOR('',#29051,1.);
#7619=VECTOR('',#29056,1.);
#7620=VECTOR('',#29057,1.);
#7621=VECTOR('',#29060,1.);
#7622=VECTOR('',#29061,1.);
#7623=VECTOR('',#29066,1.);
#7624=VECTOR('',#29071,0.12);
#7625=VECTOR('',#29074,1.);
#7626=VECTOR('',#29077,1.);
#7627=VECTOR('',#29080,1.);
#7628=VECTOR('',#29085,1.);
#7629=VECTOR('',#29088,1.);
#7630=VECTOR('',#29091,1.);
#7631=VECTOR('',#29096,1.);
#7632=VECTOR('',#29097,1.);
#7633=VECTOR('',#29100,1.);
#7634=VECTOR('',#29101,1.);
#7635=VECTOR('',#29106,1.);
#7636=VECTOR('',#29107,1.);
#7637=VECTOR('',#29110,1.);
#7638=VECTOR('',#29111,1.);
#7639=VECTOR('',#29116,1.);
#7640=VECTOR('',#29123,1.);
#7641=VECTOR('',#29124,1.);
#7642=VECTOR('',#29127,1.);
#7643=VECTOR('',#29128,1.);
#7644=VECTOR('',#29133,1.);
#7645=VECTOR('',#29134,1.);
#7646=VECTOR('',#29137,1.);
#7647=VECTOR('',#29138,1.);
#7648=VECTOR('',#29143,1.);
#7649=VECTOR('',#29148,0.12);
#7650=VECTOR('',#29151,1.);
#7651=VECTOR('',#29156,1.);
#7652=VECTOR('',#29157,1.);
#7653=VECTOR('',#29160,1.);
#7654=VECTOR('',#29161,1.);
#7655=VECTOR('',#29166,1.);
#7656=VECTOR('',#29171,1.);
#7657=VECTOR('',#29172,1.);
#7658=VECTOR('',#29175,1.);
#7659=VECTOR('',#29176,1.);
#7660=VECTOR('',#29181,1.);
#7661=VECTOR('',#29182,1.);
#7662=VECTOR('',#29185,1.);
#7663=VECTOR('',#29186,1.);
#7664=VECTOR('',#29191,1.);
#7665=VECTOR('',#29198,1.);
#7666=VECTOR('',#29199,1.);
#7667=VECTOR('',#29202,1.);
#7668=VECTOR('',#29203,1.);
#7669=VECTOR('',#29208,1.);
#7670=VECTOR('',#29209,1.);
#7671=VECTOR('',#29212,1.);
#7672=VECTOR('',#29213,1.);
#7673=VECTOR('',#29218,1.);
#7674=VECTOR('',#29225,1.);
#7675=VECTOR('',#29226,1.);
#7676=VECTOR('',#29229,1.);
#7677=VECTOR('',#29230,1.);
#7678=VECTOR('',#29235,1.);
#7679=VECTOR('',#29236,1.);
#7680=VECTOR('',#29239,1.);
#7681=VECTOR('',#29240,1.);
#7682=VECTOR('',#29245,1.);
#7683=VECTOR('',#29252,1.);
#7684=VECTOR('',#29253,1.);
#7685=VECTOR('',#29256,1.);
#7686=VECTOR('',#29257,1.);
#7687=VECTOR('',#29262,1.);
#7688=VECTOR('',#29267,1.);
#7689=VECTOR('',#29268,1.);
#7690=VECTOR('',#29271,1.);
#7691=VECTOR('',#29272,1.);
#7692=VECTOR('',#29277,0.12);
#7693=VECTOR('',#29278,1.);
#7694=VECTOR('',#29281,1.);
#7695=VECTOR('',#29288,1.);
#7696=VECTOR('',#29289,1.);
#7697=VECTOR('',#29292,1.);
#7698=VECTOR('',#29293,1.);
#7699=VECTOR('',#29298,1.);
#7700=VECTOR('',#29303,0.12);
#7701=VECTOR('',#29304,1.);
#7702=VECTOR('',#29307,1.);
#7703=VECTOR('',#29314,1.);
#7704=VECTOR('',#29315,1.);
#7705=VECTOR('',#29318,1.);
#7706=VECTOR('',#29319,1.);
#7707=VECTOR('',#29324,1.);
#7708=VECTOR('',#29329,0.12);
#7709=VECTOR('',#29330,1.);
#7710=VECTOR('',#29333,1.);
#7711=VECTOR('',#29348,1.);
#7712=VECTOR('',#29357,1.);
#7713=VECTOR('',#29420,3.8);
#7714=VECTOR('',#29429,4.095);
#7715=VECTOR('',#29432,0.9025);
#9175=CIRCLE('',#25060,0.105);
#9176=CIRCLE('',#25062,0.105);
#9177=CIRCLE('',#25064,0.155);
#9178=CIRCLE('',#25066,0.105);
#9179=CIRCLE('',#25068,0.105);
#9180=CIRCLE('',#25070,0.155);
#9181=CIRCLE('',#25072,0.13);
#9182=CIRCLE('',#25074,0.13);
#9183=CIRCLE('',#25076,0.180000000000001);
#9184=CIRCLE('',#25078,0.13);
#9185=CIRCLE('',#25080,0.13);
#9186=CIRCLE('',#25082,0.18);
#9187=CIRCLE('',#25084,0.13);
#9188=CIRCLE('',#25086,0.13);
#9189=CIRCLE('',#25088,0.18);
#9190=CIRCLE('',#25090,0.128333333333333);
#9191=CIRCLE('',#25091,0.12);
#9192=CIRCLE('',#25093,0.12);
#9193=CIRCLE('',#25095,0.145);
#9194=CIRCLE('',#25097,0.21);
#9195=CIRCLE('',#25099,0.21);
#9196=CIRCLE('',#25101,0.128333333333333);
#9197=CIRCLE('',#25102,0.12);
#9198=CIRCLE('',#25104,0.12);
#9199=CIRCLE('',#25106,0.145);
#9200=CIRCLE('',#25108,0.21);
#9201=CIRCLE('',#25110,0.21);
#9202=CIRCLE('',#25112,0.128333333333333);
#9203=CIRCLE('',#25113,0.12);
#9204=CIRCLE('',#25115,0.12);
#9205=CIRCLE('',#25117,0.145);
#9206=CIRCLE('',#25119,0.21);
#9207=CIRCLE('',#25121,0.21);
#9208=CIRCLE('',#25123,0.128333333333333);
#9209=CIRCLE('',#25124,0.12);
#9210=CIRCLE('',#25126,0.12);
#9211=CIRCLE('',#25128,0.145);
#9212=CIRCLE('',#25130,0.21);
#9213=CIRCLE('',#25132,0.21);
#9214=CIRCLE('',#25134,0.128333333333333);
#9215=CIRCLE('',#25135,0.12);
#9216=CIRCLE('',#25137,0.12);
#9217=CIRCLE('',#25139,0.145);
#9218=CIRCLE('',#25141,0.21);
#9219=CIRCLE('',#25143,0.21);
#9220=CIRCLE('',#25145,0.128333333333333);
#9221=CIRCLE('',#25146,0.120000000000001);
#9222=CIRCLE('',#25148,0.120000000000001);
#9223=CIRCLE('',#25150,0.145);
#9224=CIRCLE('',#25152,0.21);
#9225=CIRCLE('',#25154,0.21);
#9226=CIRCLE('',#25156,0.128333333333333);
#9227=CIRCLE('',#25157,0.12);
#9228=CIRCLE('',#25159,0.12);
#9229=CIRCLE('',#25161,0.145);
#9230=CIRCLE('',#25163,0.21);
#9231=CIRCLE('',#25165,0.21);
#9232=CIRCLE('',#25167,0.128333333333332);
#9233=CIRCLE('',#25168,0.12);
#9234=CIRCLE('',#25170,0.12);
#9235=CIRCLE('',#25172,0.145);
#9236=CIRCLE('',#25174,0.21);
#9237=CIRCLE('',#25176,0.21);
#9238=CIRCLE('',#25178,0.128333333333333);
#9239=CIRCLE('',#25179,0.12);
#9240=CIRCLE('',#25181,0.12);
#9241=CIRCLE('',#25183,0.145);
#9242=CIRCLE('',#25185,0.21);
#9243=CIRCLE('',#25187,0.21);
#9244=CIRCLE('',#25189,0.128333333333333);
#9245=CIRCLE('',#25190,0.12);
#9246=CIRCLE('',#25192,0.12);
#9247=CIRCLE('',#25194,0.145);
#9248=CIRCLE('',#25196,0.21);
#9249=CIRCLE('',#25198,0.21);
#9250=CIRCLE('',#25200,0.128333333333333);
#9251=CIRCLE('',#25201,0.12);
#9252=CIRCLE('',#25203,0.12);
#9253=CIRCLE('',#25205,0.145);
#9254=CIRCLE('',#25207,0.21);
#9255=CIRCLE('',#25209,0.21);
#9256=CIRCLE('',#25211,0.128333333333333);
#9257=CIRCLE('',#25212,0.12);
#9258=CIRCLE('',#25214,0.12);
#9259=CIRCLE('',#25216,0.145);
#9260=CIRCLE('',#25218,0.21);
#9261=CIRCLE('',#25220,0.21);
#9262=CIRCLE('',#25222,0.74);
#9263=CIRCLE('',#25223,0.7);
#9264=CIRCLE('',#25224,0.7);
#9265=CIRCLE('',#25226,0.7);
#9266=CIRCLE('',#25227,0.7);
#9267=CIRCLE('',#25229,3.8);
#9268=CIRCLE('',#25231,0.74);
#9269=CIRCLE('',#25233,0.9025);
#9270=CIRCLE('',#25235,4.6);
#9271=CIRCLE('',#25236,4.6);
#9272=CIRCLE('',#25237,4.57);
#9273=CIRCLE('',#25239,4.6);
#9274=CIRCLE('',#25240,4.6);
#9275=CIRCLE('',#25242,4.095);
#9276=CIRCLE('',#25244,4.57);
#9277=CIRCLE('',#25246,0.12);
#9278=CIRCLE('',#25247,4.);
#9279=CIRCLE('',#25248,0.12);
#9280=CIRCLE('',#25249,4.);
#9281=CIRCLE('',#25250,0.12);
#9282=CIRCLE('',#25251,0.12);
#9283=CIRCLE('',#25252,0.12);
#9284=CIRCLE('',#25253,0.12);
#9285=CIRCLE('',#25254,4.);
#9286=CIRCLE('',#25255,4.);
#9287=CIRCLE('',#25256,0.12);
#9288=CIRCLE('',#25257,0.12);
#9289=CIRCLE('',#25258,0.12);
#9290=CIRCLE('',#25259,4.);
#9291=CIRCLE('',#25260,0.12);
#9292=CIRCLE('',#25261,4.);
#9293=CIRCLE('',#25262,0.12);
#9294=CIRCLE('',#25263,0.12);
#9295=CIRCLE('',#25264,0.12);
#9296=CIRCLE('',#25265,0.12);
#9297=CIRCLE('',#25266,4.);
#9298=CIRCLE('',#25267,4.);
#9299=CIRCLE('',#25268,0.12);
#9300=CIRCLE('',#25269,0.12);
#9301=CIRCLE('',#25270,0.12);
#9302=CIRCLE('',#25271,4.);
#9303=CIRCLE('',#25272,0.12);
#9304=CIRCLE('',#25273,4.);
#9305=CIRCLE('',#25274,0.12);
#9306=CIRCLE('',#25275,0.12);
#9307=CIRCLE('',#25276,0.12);
#9308=CIRCLE('',#25277,0.12);
#9309=CIRCLE('',#25278,4.);
#9310=CIRCLE('',#25279,4.);
#9311=CIRCLE('',#25280,0.12);
#9312=CIRCLE('',#25281,0.12);
#9313=CIRCLE('',#25282,0.12);
#9314=CIRCLE('',#25283,0.12);
#9315=CIRCLE('',#25284,0.12);
#9316=CIRCLE('',#25285,0.12);
#9317=CIRCLE('',#25286,0.12);
#9318=CIRCLE('',#25287,0.12);
#9319=CIRCLE('',#25288,0.12);
#9320=CIRCLE('',#25289,0.12);
#9321=CIRCLE('',#25290,0.12);
#9322=CIRCLE('',#25291,0.12);
#9323=CIRCLE('',#25292,0.12);
#9324=CIRCLE('',#25293,0.12);
#9325=CIRCLE('',#25294,0.12);
#9326=CIRCLE('',#25295,0.12);
#9327=CIRCLE('',#25296,0.12);
#9328=CIRCLE('',#25297,0.12);
#9329=CIRCLE('',#25298,0.12);
#9330=CIRCLE('',#25299,0.12);
#9331=CIRCLE('',#25300,0.12);
#9332=CIRCLE('',#25301,0.12);
#9333=CIRCLE('',#25302,0.12);
#9334=CIRCLE('',#25303,0.12);
#9335=CIRCLE('',#25304,0.12);
#9336=CIRCLE('',#25305,0.12);
#9337=CIRCLE('',#25306,0.12);
#9338=CIRCLE('',#25307,0.12);
#9339=CIRCLE('',#25308,0.12);
#9340=CIRCLE('',#25309,0.12);
#9341=CIRCLE('',#25310,0.12);
#9342=CIRCLE('',#25311,0.12);
#9343=CIRCLE('',#25312,0.12);
#9344=CIRCLE('',#25313,0.12);
#9345=CIRCLE('',#25314,0.12);
#9346=CIRCLE('',#25315,0.12);
#9347=CIRCLE('',#25316,0.12);
#9348=CIRCLE('',#25317,0.12);
#9349=CIRCLE('',#25318,0.12);
#9350=CIRCLE('',#25319,0.12);
#9351=CIRCLE('',#25320,0.12);
#9352=CIRCLE('',#25321,0.12);
#9353=CIRCLE('',#25322,0.12);
#9354=CIRCLE('',#25323,0.12);
#9355=CIRCLE('',#25324,0.12);
#9356=CIRCLE('',#25325,0.12);
#9357=CIRCLE('',#25326,0.12);
#9358=CIRCLE('',#25327,0.12);
#9359=CIRCLE('',#25328,0.12);
#9360=CIRCLE('',#25329,0.12);
#9361=CIRCLE('',#25330,0.12);
#9362=CIRCLE('',#25331,0.12);
#9363=CIRCLE('',#25332,0.12);
#9364=CIRCLE('',#25333,0.12);
#9365=CIRCLE('',#25334,0.12);
#9366=CIRCLE('',#25335,0.12);
#9367=CIRCLE('',#25336,0.9025);
#9368=CIRCLE('',#25338,0.12);
#9369=CIRCLE('',#25340,0.12);
#9370=CIRCLE('',#25343,0.12);
#9371=CIRCLE('',#25345,4.);
#9372=CIRCLE('',#25347,0.12);
#9373=CIRCLE('',#25350,0.12);
#9374=CIRCLE('',#25352,0.12);
#9375=CIRCLE('',#25356,0.12);
#9376=CIRCLE('',#25359,0.12);
#9377=CIRCLE('',#25361,0.12);
#9378=CIRCLE('',#25365,0.12);
#9379=CIRCLE('',#25367,0.12);
#9380=CIRCLE('',#25370,0.12);
#9381=CIRCLE('',#25372,0.12);
#9382=CIRCLE('',#25376,0.12);
#9383=CIRCLE('',#25379,0.12);
#9384=CIRCLE('',#25381,0.12);
#9385=CIRCLE('',#25385,0.12);
#9386=CIRCLE('',#25388,0.12);
#9387=CIRCLE('',#25390,0.12);
#9388=CIRCLE('',#25391,4.);
#9389=CIRCLE('',#25395,0.12);
#9390=CIRCLE('',#25398,0.12);
#9391=CIRCLE('',#25400,0.12);
#9392=CIRCLE('',#25404,0.12);
#9393=CIRCLE('',#25407,0.12);
#9394=CIRCLE('',#25409,0.12);
#9395=CIRCLE('',#25413,0.12);
#9396=CIRCLE('',#25415,0.12);
#9397=CIRCLE('',#25416,4.);
#9398=CIRCLE('',#25421,0.12);
#9399=CIRCLE('',#25424,0.12);
#9400=CIRCLE('',#25426,0.12);
#9401=CIRCLE('',#25430,0.12);
#9402=CIRCLE('',#25433,0.12);
#9403=CIRCLE('',#25435,0.12);
#9404=CIRCLE('',#25439,0.12);
#9405=CIRCLE('',#25442,0.12);
#9406=CIRCLE('',#25444,0.12);
#9407=CIRCLE('',#25445,4.);
#9408=CIRCLE('',#25449,0.12);
#9409=CIRCLE('',#25452,0.12);
#9410=CIRCLE('',#25454,0.12);
#9411=CIRCLE('',#25458,0.12);
#9412=CIRCLE('',#25461,0.12);
#9413=CIRCLE('',#25463,0.12);
#9414=CIRCLE('',#25467,0.12);
#9415=CIRCLE('',#25470,0.12);
#9416=CIRCLE('',#25472,0.12);
#9417=CIRCLE('',#25476,0.12);
#9418=CIRCLE('',#25478,0.12);
#9419=CIRCLE('',#25481,0.12);
#9420=CIRCLE('',#25483,0.12);
#9421=CIRCLE('',#25487,0.12);
#9422=CIRCLE('',#25490,0.12);
#9423=CIRCLE('',#25492,0.12);
#9424=CIRCLE('',#25496,0.12);
#9425=CIRCLE('',#25498,0.12);
#9426=CIRCLE('',#25499,4.);
#9427=CIRCLE('',#25504,0.12);
#9428=CIRCLE('',#25507,0.12);
#9429=CIRCLE('',#25509,0.12);
#9430=CIRCLE('',#25513,0.12);
#9431=CIRCLE('',#25516,0.12);
#9432=CIRCLE('',#25518,0.12);
#9433=CIRCLE('',#25522,0.12);
#9434=CIRCLE('',#25524,0.12);
#9435=CIRCLE('',#25526,4.);
#9436=CIRCLE('',#25529,0.12);
#9437=CIRCLE('',#25532,0.12);
#9438=CIRCLE('',#25534,0.12);
#9439=CIRCLE('',#25538,0.12);
#9440=CIRCLE('',#25541,0.12);
#9441=CIRCLE('',#25543,0.12);
#9442=CIRCLE('',#25547,0.12);
#9443=CIRCLE('',#25550,0.12);
#9444=CIRCLE('',#25552,0.12);
#9445=CIRCLE('',#25556,0.12);
#9446=CIRCLE('',#25558,4.);
#9447=CIRCLE('',#25561,0.12);
#9448=CIRCLE('',#25564,0.12);
#9449=CIRCLE('',#25566,4.);
#9450=CIRCLE('',#25568,0.12);
#9451=CIRCLE('',#25570,4.);
#9452=CIRCLE('',#25573,0.12);
#9453=CIRCLE('',#25575,4.);
#9454=CIRCLE('',#25577,0.12);
#9455=CIRCLE('',#25579,4.);
#9456=CIRCLE('',#25582,0.12);
#9457=CIRCLE('',#25584,4.);
#9458=CIRCLE('',#25626,3.8);
#9459=CIRCLE('',#25628,4.095);
#10200=VERTEX_POINT('',#34452);
#10201=VERTEX_POINT('',#34453);
#10202=VERTEX_POINT('',#34457);
#10203=VERTEX_POINT('',#34461);
#10204=VERTEX_POINT('',#34465);
#10205=VERTEX_POINT('',#34466);
#10206=VERTEX_POINT('',#34470);
#10207=VERTEX_POINT('',#34474);
#10208=VERTEX_POINT('',#34478);
#10209=VERTEX_POINT('',#34479);
#10210=VERTEX_POINT('',#34483);
#10211=VERTEX_POINT('',#34487);
#10212=VERTEX_POINT('',#34491);
#10213=VERTEX_POINT('',#34492);
#10214=VERTEX_POINT('',#34496);
#10215=VERTEX_POINT('',#34500);
#10216=VERTEX_POINT('',#34504);
#10217=VERTEX_POINT('',#34505);
#10218=VERTEX_POINT('',#34509);
#10219=VERTEX_POINT('',#34513);
#10220=VERTEX_POINT('',#34517);
#10221=VERTEX_POINT('',#34519);
#10222=VERTEX_POINT('',#34523);
#10223=VERTEX_POINT('',#34527);
#10224=VERTEX_POINT('',#34531);
#10225=VERTEX_POINT('',#34534);
#10226=VERTEX_POINT('',#34538);
#10227=VERTEX_POINT('',#34540);
#10228=VERTEX_POINT('',#34544);
#10229=VERTEX_POINT('',#34548);
#10230=VERTEX_POINT('',#34552);
#10231=VERTEX_POINT('',#34555);
#10232=VERTEX_POINT('',#34559);
#10233=VERTEX_POINT('',#34561);
#10234=VERTEX_POINT('',#34565);
#10235=VERTEX_POINT('',#34569);
#10236=VERTEX_POINT('',#34573);
#10237=VERTEX_POINT('',#34576);
#10238=VERTEX_POINT('',#34580);
#10239=VERTEX_POINT('',#34582);
#10240=VERTEX_POINT('',#34586);
#10241=VERTEX_POINT('',#34590);
#10242=VERTEX_POINT('',#34594);
#10243=VERTEX_POINT('',#34597);
#10244=VERTEX_POINT('',#34601);
#10245=VERTEX_POINT('',#34603);
#10246=VERTEX_POINT('',#34607);
#10247=VERTEX_POINT('',#34611);
#10248=VERTEX_POINT('',#34615);
#10249=VERTEX_POINT('',#34618);
#10250=VERTEX_POINT('',#34622);
#10251=VERTEX_POINT('',#34624);
#10252=VERTEX_POINT('',#34628);
#10253=VERTEX_POINT('',#34632);
#10254=VERTEX_POINT('',#34636);
#10255=VERTEX_POINT('',#34639);
#10256=VERTEX_POINT('',#34643);
#10257=VERTEX_POINT('',#34645);
#10258=VERTEX_POINT('',#34649);
#10259=VERTEX_POINT('',#34653);
#10260=VERTEX_POINT('',#34657);
#10261=VERTEX_POINT('',#34660);
#10262=VERTEX_POINT('',#34664);
#10263=VERTEX_POINT('',#34666);
#10264=VERTEX_POINT('',#34670);
#10265=VERTEX_POINT('',#34674);
#10266=VERTEX_POINT('',#34678);
#10267=VERTEX_POINT('',#34681);
#10268=VERTEX_POINT('',#34685);
#10269=VERTEX_POINT('',#34687);
#10270=VERTEX_POINT('',#34691);
#10271=VERTEX_POINT('',#34695);
#10272=VERTEX_POINT('',#34699);
#10273=VERTEX_POINT('',#34702);
#10274=VERTEX_POINT('',#34706);
#10275=VERTEX_POINT('',#34708);
#10276=VERTEX_POINT('',#34712);
#10277=VERTEX_POINT('',#34716);
#10278=VERTEX_POINT('',#34720);
#10279=VERTEX_POINT('',#34723);
#10280=VERTEX_POINT('',#34727);
#10281=VERTEX_POINT('',#34729);
#10282=VERTEX_POINT('',#34733);
#10283=VERTEX_POINT('',#34737);
#10284=VERTEX_POINT('',#34741);
#10285=VERTEX_POINT('',#34744);
#10286=VERTEX_POINT('',#34748);
#10287=VERTEX_POINT('',#34750);
#10288=VERTEX_POINT('',#34754);
#10289=VERTEX_POINT('',#34758);
#10290=VERTEX_POINT('',#34762);
#10291=VERTEX_POINT('',#34765);
#10292=VERTEX_POINT('',#34769);
#10293=VERTEX_POINT('',#34771);
#10294=VERTEX_POINT('',#34773);
#10295=VERTEX_POINT('',#34777);
#10296=VERTEX_POINT('',#34778);
#10297=VERTEX_POINT('',#34783);
#10298=VERTEX_POINT('',#34786);
#10299=VERTEX_POINT('',#34790);
#10300=VERTEX_POINT('',#34793);
#10301=VERTEX_POINT('',#34794);
#10302=VERTEX_POINT('',#34797);
#10303=VERTEX_POINT('',#34801);
#10304=VERTEX_POINT('',#34802);
#10305=VERTEX_POINT('',#34807);
#10306=VERTEX_POINT('',#34810);
#10307=VERTEX_POINT('',#34814);
#10308=VERTEX_POINT('',#34815);
#10309=VERTEX_POINT('',#34817);
#10310=VERTEX_POINT('',#34819);
#10311=VERTEX_POINT('',#34821);
#10312=VERTEX_POINT('',#34824);
#10313=VERTEX_POINT('',#34825);
#10314=VERTEX_POINT('',#34827);
#10315=VERTEX_POINT('',#34829);
#10316=VERTEX_POINT('',#34831);
#10317=VERTEX_POINT('',#34834);
#10318=VERTEX_POINT('',#34835);
#10319=VERTEX_POINT('',#34837);
#10320=VERTEX_POINT('',#34839);
#10321=VERTEX_POINT('',#34841);
#10322=VERTEX_POINT('',#34844);
#10323=VERTEX_POINT('',#34845);
#10324=VERTEX_POINT('',#34847);
#10325=VERTEX_POINT('',#34849);
#10326=VERTEX_POINT('',#34851);
#10327=VERTEX_POINT('',#34854);
#10328=VERTEX_POINT('',#34855);
#10329=VERTEX_POINT('',#34857);
#10330=VERTEX_POINT('',#34859);
#10331=VERTEX_POINT('',#34861);
#10332=VERTEX_POINT('',#34864);
#10333=VERTEX_POINT('',#34865);
#10334=VERTEX_POINT('',#34867);
#10335=VERTEX_POINT('',#34869);
#10336=VERTEX_POINT('',#34871);
#10337=VERTEX_POINT('',#34874);
#10338=VERTEX_POINT('',#34875);
#10339=VERTEX_POINT('',#34877);
#10340=VERTEX_POINT('',#34879);
#10341=VERTEX_POINT('',#34881);
#10342=VERTEX_POINT('',#34884);
#10343=VERTEX_POINT('',#34885);
#10344=VERTEX_POINT('',#34887);
#10345=VERTEX_POINT('',#34889);
#10346=VERTEX_POINT('',#34891);
#10347=VERTEX_POINT('',#34894);
#10348=VERTEX_POINT('',#34895);
#10349=VERTEX_POINT('',#34897);
#10350=VERTEX_POINT('',#34899);
#10351=VERTEX_POINT('',#34901);
#10352=VERTEX_POINT('',#34904);
#10353=VERTEX_POINT('',#34905);
#10354=VERTEX_POINT('',#34907);
#10355=VERTEX_POINT('',#34909);
#10356=VERTEX_POINT('',#34911);
#10357=VERTEX_POINT('',#34914);
#10358=VERTEX_POINT('',#34915);
#10359=VERTEX_POINT('',#34917);
#10360=VERTEX_POINT('',#34919);
#10361=VERTEX_POINT('',#34921);
#10362=VERTEX_POINT('',#34924);
#10363=VERTEX_POINT('',#34925);
#10364=VERTEX_POINT('',#34927);
#10365=VERTEX_POINT('',#34929);
#10366=VERTEX_POINT('',#34931);
#10367=VERTEX_POINT('',#34934);
#10368=VERTEX_POINT('',#34935);
#10369=VERTEX_POINT('',#34937);
#10370=VERTEX_POINT('',#34939);
#10371=VERTEX_POINT('',#34941);
#10372=VERTEX_POINT('',#34943);
#10373=VERTEX_POINT('',#34946);
#10374=VERTEX_POINT('',#34947);
#10375=VERTEX_POINT('',#34949);
#10376=VERTEX_POINT('',#34951);
#10377=VERTEX_POINT('',#34953);
#10378=VERTEX_POINT('',#34955);
#10379=VERTEX_POINT('',#34958);
#10380=VERTEX_POINT('',#34959);
#10381=VERTEX_POINT('',#34961);
#10382=VERTEX_POINT('',#34963);
#10383=VERTEX_POINT('',#34965);
#10384=VERTEX_POINT('',#34967);
#10385=VERTEX_POINT('',#34970);
#10386=VERTEX_POINT('',#34971);
#10387=VERTEX_POINT('',#34973);
#10388=VERTEX_POINT('',#34975);
#10389=VERTEX_POINT('',#34977);
#10390=VERTEX_POINT('',#34979);
#10391=VERTEX_POINT('',#34982);
#10392=VERTEX_POINT('',#34983);
#10393=VERTEX_POINT('',#34985);
#10394=VERTEX_POINT('',#34987);
#10395=VERTEX_POINT('',#34989);
#10396=VERTEX_POINT('',#34991);
#10397=VERTEX_POINT('',#34994);
#10398=VERTEX_POINT('',#34995);
#10399=VERTEX_POINT('',#34997);
#10400=VERTEX_POINT('',#34999);
#10401=VERTEX_POINT('',#35001);
#10402=VERTEX_POINT('',#35003);
#10403=VERTEX_POINT('',#35006);
#10404=VERTEX_POINT('',#35007);
#10405=VERTEX_POINT('',#35009);
#10406=VERTEX_POINT('',#35011);
#10407=VERTEX_POINT('',#35013);
#10408=VERTEX_POINT('',#35015);
#10409=VERTEX_POINT('',#35018);
#10410=VERTEX_POINT('',#35019);
#10411=VERTEX_POINT('',#35021);
#10412=VERTEX_POINT('',#35023);
#10413=VERTEX_POINT('',#35025);
#10414=VERTEX_POINT('',#35027);
#10415=VERTEX_POINT('',#35030);
#10416=VERTEX_POINT('',#35031);
#10417=VERTEX_POINT('',#35033);
#10418=VERTEX_POINT('',#35035);
#10419=VERTEX_POINT('',#35037);
#10420=VERTEX_POINT('',#35039);
#10421=VERTEX_POINT('',#35042);
#10422=VERTEX_POINT('',#35043);
#10423=VERTEX_POINT('',#35045);
#10424=VERTEX_POINT('',#35047);
#10425=VERTEX_POINT('',#35049);
#10426=VERTEX_POINT('',#35051);
#10427=VERTEX_POINT('',#35054);
#10428=VERTEX_POINT('',#35055);
#10429=VERTEX_POINT('',#35057);
#10430=VERTEX_POINT('',#35059);
#10431=VERTEX_POINT('',#35061);
#10432=VERTEX_POINT('',#35063);
#10433=VERTEX_POINT('',#35066);
#10434=VERTEX_POINT('',#35067);
#10435=VERTEX_POINT('',#35069);
#10436=VERTEX_POINT('',#35071);
#10437=VERTEX_POINT('',#35073);
#10438=VERTEX_POINT('',#35075);
#10439=VERTEX_POINT('',#35078);
#10440=VERTEX_POINT('',#35079);
#10441=VERTEX_POINT('',#35081);
#10442=VERTEX_POINT('',#35083);
#10443=VERTEX_POINT('',#35085);
#10444=VERTEX_POINT('',#35087);
#10445=VERTEX_POINT('',#35090);
#10446=VERTEX_POINT('',#35091);
#10447=VERTEX_POINT('',#35093);
#10448=VERTEX_POINT('',#35095);
#10449=VERTEX_POINT('',#35097);
#10450=VERTEX_POINT('',#35099);
#10451=VERTEX_POINT('',#35102);
#10452=VERTEX_POINT('',#35103);
#10453=VERTEX_POINT('',#35105);
#10454=VERTEX_POINT('',#35107);
#10455=VERTEX_POINT('',#35109);
#10456=VERTEX_POINT('',#35111);
#10457=VERTEX_POINT('',#35114);
#10458=VERTEX_POINT('',#35115);
#10459=VERTEX_POINT('',#35117);
#10460=VERTEX_POINT('',#35119);
#10461=VERTEX_POINT('',#35121);
#10462=VERTEX_POINT('',#35123);
#10463=VERTEX_POINT('',#35126);
#10464=VERTEX_POINT('',#35127);
#10465=VERTEX_POINT('',#35129);
#10466=VERTEX_POINT('',#35131);
#10467=VERTEX_POINT('',#35133);
#10468=VERTEX_POINT('',#35135);
#10469=VERTEX_POINT('',#35138);
#10470=VERTEX_POINT('',#35139);
#10471=VERTEX_POINT('',#35141);
#10472=VERTEX_POINT('',#35143);
#10473=VERTEX_POINT('',#35145);
#10474=VERTEX_POINT('',#35147);
#10475=VERTEX_POINT('',#35150);
#10476=VERTEX_POINT('',#35153);
#10477=VERTEX_POINT('',#35155);
#10478=VERTEX_POINT('',#35159);
#10479=VERTEX_POINT('',#35160);
#10480=VERTEX_POINT('',#35165);
#10481=VERTEX_POINT('',#35169);
#10482=VERTEX_POINT('',#35170);
#10483=VERTEX_POINT('',#35178);
#10484=VERTEX_POINT('',#35179);
#10485=VERTEX_POINT('',#35184);
#10486=VERTEX_POINT('',#35188);
#10487=VERTEX_POINT('',#35189);
#10488=VERTEX_POINT('',#35195);
#10489=VERTEX_POINT('',#35202);
#10490=VERTEX_POINT('',#35203);
#10491=VERTEX_POINT('',#35208);
#10492=VERTEX_POINT('',#35212);
#10493=VERTEX_POINT('',#35213);
#10494=VERTEX_POINT('',#35219);
#10495=VERTEX_POINT('',#35226);
#10496=VERTEX_POINT('',#35228);
#10497=VERTEX_POINT('',#35232);
#10498=VERTEX_POINT('',#35233);
#10499=VERTEX_POINT('',#35238);
#10500=VERTEX_POINT('',#35242);
#10501=VERTEX_POINT('',#35243);
#10502=VERTEX_POINT('',#35249);
#10503=VERTEX_POINT('',#35256);
#10504=VERTEX_POINT('',#35257);
#10505=VERTEX_POINT('',#35262);
#10506=VERTEX_POINT('',#35266);
#10507=VERTEX_POINT('',#35267);
#10508=VERTEX_POINT('',#35273);
#10509=VERTEX_POINT('',#35280);
#10510=VERTEX_POINT('',#35281);
#10511=VERTEX_POINT('',#35286);
#10512=VERTEX_POINT('',#35290);
#10513=VERTEX_POINT('',#35291);
#10514=VERTEX_POINT('',#35296);
#10515=VERTEX_POINT('',#35298);
#10516=VERTEX_POINT('',#35300);
#10517=VERTEX_POINT('',#35308);
#10518=VERTEX_POINT('',#35309);
#10519=VERTEX_POINT('',#35314);
#10520=VERTEX_POINT('',#35318);
#10521=VERTEX_POINT('',#35319);
#10522=VERTEX_POINT('',#35325);
#10523=VERTEX_POINT('',#35332);
#10524=VERTEX_POINT('',#35333);
#10525=VERTEX_POINT('',#35338);
#10526=VERTEX_POINT('',#35342);
#10527=VERTEX_POINT('',#35343);
#10528=VERTEX_POINT('',#35349);
#10529=VERTEX_POINT('',#35356);
#10530=VERTEX_POINT('',#35358);
#10531=VERTEX_POINT('',#35362);
#10532=VERTEX_POINT('',#35364);
#10533=VERTEX_POINT('',#35366);
#10534=VERTEX_POINT('',#35376);
#10535=VERTEX_POINT('',#35377);
#10536=VERTEX_POINT('',#35382);
#10537=VERTEX_POINT('',#35386);
#10538=VERTEX_POINT('',#35387);
#10539=VERTEX_POINT('',#35393);
#10540=VERTEX_POINT('',#35400);
#10541=VERTEX_POINT('',#35401);
#10542=VERTEX_POINT('',#35406);
#10543=VERTEX_POINT('',#35410);
#10544=VERTEX_POINT('',#35411);
#10545=VERTEX_POINT('',#35417);
#10546=VERTEX_POINT('',#35424);
#10547=VERTEX_POINT('',#35425);
#10548=VERTEX_POINT('',#35430);
#10549=VERTEX_POINT('',#35434);
#10550=VERTEX_POINT('',#35435);
#10551=VERTEX_POINT('',#35440);
#10552=VERTEX_POINT('',#35442);
#10553=VERTEX_POINT('',#35444);
#10554=VERTEX_POINT('',#35452);
#10555=VERTEX_POINT('',#35453);
#10556=VERTEX_POINT('',#35458);
#10557=VERTEX_POINT('',#35462);
#10558=VERTEX_POINT('',#35463);
#10559=VERTEX_POINT('',#35469);
#10560=VERTEX_POINT('',#35476);
#10561=VERTEX_POINT('',#35477);
#10562=VERTEX_POINT('',#35482);
#10563=VERTEX_POINT('',#35486);
#10564=VERTEX_POINT('',#35487);
#10565=VERTEX_POINT('',#35493);
#10566=VERTEX_POINT('',#35500);
#10567=VERTEX_POINT('',#35501);
#10568=VERTEX_POINT('',#35506);
#10569=VERTEX_POINT('',#35510);
#10570=VERTEX_POINT('',#35511);
#10571=VERTEX_POINT('',#35517);
#10572=VERTEX_POINT('',#35524);
#10573=VERTEX_POINT('',#35526);
#10574=VERTEX_POINT('',#35530);
#10575=VERTEX_POINT('',#35531);
#10576=VERTEX_POINT('',#35536);
#10577=VERTEX_POINT('',#35540);
#10578=VERTEX_POINT('',#35541);
#10579=VERTEX_POINT('',#35547);
#10580=VERTEX_POINT('',#35554);
#10581=VERTEX_POINT('',#35555);
#10582=VERTEX_POINT('',#35560);
#10583=VERTEX_POINT('',#35564);
#10584=VERTEX_POINT('',#35565);
#10585=VERTEX_POINT('',#35571);
#10586=VERTEX_POINT('',#35578);
#10587=VERTEX_POINT('',#35580);
#10588=VERTEX_POINT('',#35584);
#10589=VERTEX_POINT('',#35586);
#10590=VERTEX_POINT('',#35588);
#10591=VERTEX_POINT('',#35598);
#10592=VERTEX_POINT('',#35599);
#10593=VERTEX_POINT('',#35604);
#10594=VERTEX_POINT('',#35608);
#10595=VERTEX_POINT('',#35609);
#10596=VERTEX_POINT('',#35615);
#10597=VERTEX_POINT('',#35622);
#10598=VERTEX_POINT('',#35623);
#10599=VERTEX_POINT('',#35628);
#10600=VERTEX_POINT('',#35632);
#10601=VERTEX_POINT('',#35633);
#10602=VERTEX_POINT('',#35639);
#10603=VERTEX_POINT('',#35646);
#10604=VERTEX_POINT('',#35648);
#10605=VERTEX_POINT('',#35652);
#10606=VERTEX_POINT('',#35653);
#10607=VERTEX_POINT('',#35659);
#10608=VERTEX_POINT('',#35665);
#10609=VERTEX_POINT('',#35666);
#10610=VERTEX_POINT('',#35671);
#10611=VERTEX_POINT('',#35675);
#10612=VERTEX_POINT('',#35676);
#10613=VERTEX_POINT('',#35682);
#10614=VERTEX_POINT('',#35689);
#10615=VERTEX_POINT('',#35690);
#10616=VERTEX_POINT('',#35695);
#10617=VERTEX_POINT('',#35699);
#10618=VERTEX_POINT('',#35700);
#10619=VERTEX_POINT('',#35706);
#10620=VERTEX_POINT('',#35713);
#10621=VERTEX_POINT('',#35714);
#10622=VERTEX_POINT('',#35719);
#10623=VERTEX_POINT('',#35723);
#10624=VERTEX_POINT('',#35724);
#10625=VERTEX_POINT('',#35730);
#10626=VERTEX_POINT('',#35737);
#10627=VERTEX_POINT('',#35738);
#10628=VERTEX_POINT('',#35744);
#10629=VERTEX_POINT('',#35750);
#10630=VERTEX_POINT('',#35751);
#10631=VERTEX_POINT('',#35756);
#10632=VERTEX_POINT('',#35760);
#10633=VERTEX_POINT('',#35761);
#10634=VERTEX_POINT('',#35769);
#10635=VERTEX_POINT('',#35770);
#10636=VERTEX_POINT('',#35776);
#10637=VERTEX_POINT('',#35782);
#10638=VERTEX_POINT('',#35783);
#10639=VERTEX_POINT('',#35791);
#10640=VERTEX_POINT('',#35792);
#10641=VERTEX_POINT('',#35798);
#10642=VERTEX_POINT('',#35804);
#10643=VERTEX_POINT('',#35805);
#10644=VERTEX_POINT('',#35855);
#10645=VERTEX_POINT('',#35859);
#12623=EDGE_CURVE('',#10200,#10201,#5499,.T.);
#12624=EDGE_CURVE('',#10201,#10201,#9175,.T.);
#12625=EDGE_CURVE('',#10201,#10202,#5500,.T.);
#12626=EDGE_CURVE('',#10202,#10202,#9176,.T.);
#12627=EDGE_CURVE('',#10202,#10203,#5501,.T.);
#12628=EDGE_CURVE('',#10203,#10203,#9177,.T.);
#12629=EDGE_CURVE('',#10204,#10205,#5502,.T.);
#12630=EDGE_CURVE('',#10205,#10205,#9178,.T.);
#12631=EDGE_CURVE('',#10205,#10206,#5503,.T.);
#12632=EDGE_CURVE('',#10206,#10206,#9179,.T.);
#12633=EDGE_CURVE('',#10206,#10207,#5504,.T.);
#12634=EDGE_CURVE('',#10207,#10207,#9180,.T.);
#12635=EDGE_CURVE('',#10208,#10209,#5505,.T.);
#12636=EDGE_CURVE('',#10209,#10209,#9181,.T.);
#12637=EDGE_CURVE('',#10209,#10210,#5506,.T.);
#12638=EDGE_CURVE('',#10210,#10210,#9182,.T.);
#12639=EDGE_CURVE('',#10210,#10211,#5507,.T.);
#12640=EDGE_CURVE('',#10211,#10211,#9183,.T.);
#12641=EDGE_CURVE('',#10212,#10213,#5508,.T.);
#12642=EDGE_CURVE('',#10213,#10213,#9184,.T.);
#12643=EDGE_CURVE('',#10213,#10214,#5509,.T.);
#12644=EDGE_CURVE('',#10214,#10214,#9185,.T.);
#12645=EDGE_CURVE('',#10214,#10215,#5510,.T.);
#12646=EDGE_CURVE('',#10215,#10215,#9186,.T.);
#12647=EDGE_CURVE('',#10216,#10217,#5511,.T.);
#12648=EDGE_CURVE('',#10217,#10217,#9187,.T.);
#12649=EDGE_CURVE('',#10217,#10218,#5512,.T.);
#12650=EDGE_CURVE('',#10218,#10218,#9188,.T.);
#12651=EDGE_CURVE('',#10218,#10219,#5513,.T.);
#12652=EDGE_CURVE('',#10219,#10219,#9189,.T.);
#12653=EDGE_CURVE('',#10220,#10220,#9190,.T.);
#12654=EDGE_CURVE('',#10220,#10221,#5514,.T.);
#12655=EDGE_CURVE('',#10221,#10221,#9191,.T.);
#12656=EDGE_CURVE('',#10221,#10222,#5515,.T.);
#12657=EDGE_CURVE('',#10222,#10222,#9192,.T.);
#12658=EDGE_CURVE('',#10222,#10223,#5516,.T.);
#12659=EDGE_CURVE('',#10223,#10223,#9193,.T.);
#12660=EDGE_CURVE('',#10224,#10224,#9194,.T.);
#12661=EDGE_CURVE('',#10224,#10225,#5517,.T.);
#12662=EDGE_CURVE('',#10225,#10225,#9195,.T.);
#12663=EDGE_CURVE('',#10226,#10226,#9196,.T.);
#12664=EDGE_CURVE('',#10226,#10227,#5518,.T.);
#12665=EDGE_CURVE('',#10227,#10227,#9197,.T.);
#12666=EDGE_CURVE('',#10227,#10228,#5519,.T.);
#12667=EDGE_CURVE('',#10228,#10228,#9198,.T.);
#12668=EDGE_CURVE('',#10228,#10229,#5520,.T.);
#12669=EDGE_CURVE('',#10229,#10229,#9199,.T.);
#12670=EDGE_CURVE('',#10230,#10230,#9200,.T.);
#12671=EDGE_CURVE('',#10230,#10231,#5521,.T.);
#12672=EDGE_CURVE('',#10231,#10231,#9201,.T.);
#12673=EDGE_CURVE('',#10232,#10232,#9202,.T.);
#12674=EDGE_CURVE('',#10232,#10233,#5522,.T.);
#12675=EDGE_CURVE('',#10233,#10233,#9203,.T.);
#12676=EDGE_CURVE('',#10233,#10234,#5523,.T.);
#12677=EDGE_CURVE('',#10234,#10234,#9204,.T.);
#12678=EDGE_CURVE('',#10234,#10235,#5524,.T.);
#12679=EDGE_CURVE('',#10235,#10235,#9205,.T.);
#12680=EDGE_CURVE('',#10236,#10236,#9206,.T.);
#12681=EDGE_CURVE('',#10236,#10237,#5525,.T.);
#12682=EDGE_CURVE('',#10237,#10237,#9207,.T.);
#12683=EDGE_CURVE('',#10238,#10238,#9208,.T.);
#12684=EDGE_CURVE('',#10238,#10239,#5526,.T.);
#12685=EDGE_CURVE('',#10239,#10239,#9209,.T.);
#12686=EDGE_CURVE('',#10239,#10240,#5527,.T.);
#12687=EDGE_CURVE('',#10240,#10240,#9210,.T.);
#12688=EDGE_CURVE('',#10240,#10241,#5528,.T.);
#12689=EDGE_CURVE('',#10241,#10241,#9211,.T.);
#12690=EDGE_CURVE('',#10242,#10242,#9212,.T.);
#12691=EDGE_CURVE('',#10242,#10243,#5529,.T.);
#12692=EDGE_CURVE('',#10243,#10243,#9213,.T.);
#12693=EDGE_CURVE('',#10244,#10244,#9214,.T.);
#12694=EDGE_CURVE('',#10244,#10245,#5530,.T.);
#12695=EDGE_CURVE('',#10245,#10245,#9215,.T.);
#12696=EDGE_CURVE('',#10245,#10246,#5531,.T.);
#12697=EDGE_CURVE('',#10246,#10246,#9216,.T.);
#12698=EDGE_CURVE('',#10246,#10247,#5532,.T.);
#12699=EDGE_CURVE('',#10247,#10247,#9217,.T.);
#12700=EDGE_CURVE('',#10248,#10248,#9218,.T.);
#12701=EDGE_CURVE('',#10248,#10249,#5533,.T.);
#12702=EDGE_CURVE('',#10249,#10249,#9219,.T.);
#12703=EDGE_CURVE('',#10250,#10250,#9220,.T.);
#12704=EDGE_CURVE('',#10250,#10251,#5534,.T.);
#12705=EDGE_CURVE('',#10251,#10251,#9221,.T.);
#12706=EDGE_CURVE('',#10251,#10252,#5535,.T.);
#12707=EDGE_CURVE('',#10252,#10252,#9222,.T.);
#12708=EDGE_CURVE('',#10252,#10253,#5536,.T.);
#12709=EDGE_CURVE('',#10253,#10253,#9223,.T.);
#12710=EDGE_CURVE('',#10254,#10254,#9224,.T.);
#12711=EDGE_CURVE('',#10254,#10255,#5537,.T.);
#12712=EDGE_CURVE('',#10255,#10255,#9225,.T.);
#12713=EDGE_CURVE('',#10256,#10256,#9226,.T.);
#12714=EDGE_CURVE('',#10256,#10257,#5538,.T.);
#12715=EDGE_CURVE('',#10257,#10257,#9227,.T.);
#12716=EDGE_CURVE('',#10257,#10258,#5539,.T.);
#12717=EDGE_CURVE('',#10258,#10258,#9228,.T.);
#12718=EDGE_CURVE('',#10258,#10259,#5540,.T.);
#12719=EDGE_CURVE('',#10259,#10259,#9229,.T.);
#12720=EDGE_CURVE('',#10260,#10260,#9230,.T.);
#12721=EDGE_CURVE('',#10260,#10261,#5541,.T.);
#12722=EDGE_CURVE('',#10261,#10261,#9231,.T.);
#12723=EDGE_CURVE('',#10262,#10262,#9232,.T.);
#12724=EDGE_CURVE('',#10262,#10263,#5542,.T.);
#12725=EDGE_CURVE('',#10263,#10263,#9233,.T.);
#12726=EDGE_CURVE('',#10263,#10264,#5543,.T.);
#12727=EDGE_CURVE('',#10264,#10264,#9234,.T.);
#12728=EDGE_CURVE('',#10264,#10265,#5544,.T.);
#12729=EDGE_CURVE('',#10265,#10265,#9235,.T.);
#12730=EDGE_CURVE('',#10266,#10266,#9236,.T.);
#12731=EDGE_CURVE('',#10266,#10267,#5545,.T.);
#12732=EDGE_CURVE('',#10267,#10267,#9237,.T.);
#12733=EDGE_CURVE('',#10268,#10268,#9238,.T.);
#12734=EDGE_CURVE('',#10268,#10269,#5546,.T.);
#12735=EDGE_CURVE('',#10269,#10269,#9239,.T.);
#12736=EDGE_CURVE('',#10269,#10270,#5547,.T.);
#12737=EDGE_CURVE('',#10270,#10270,#9240,.T.);
#12738=EDGE_CURVE('',#10270,#10271,#5548,.T.);
#12739=EDGE_CURVE('',#10271,#10271,#9241,.T.);
#12740=EDGE_CURVE('',#10272,#10272,#9242,.T.);
#12741=EDGE_CURVE('',#10272,#10273,#5549,.T.);
#12742=EDGE_CURVE('',#10273,#10273,#9243,.T.);
#12743=EDGE_CURVE('',#10274,#10274,#9244,.T.);
#12744=EDGE_CURVE('',#10274,#10275,#5550,.T.);
#12745=EDGE_CURVE('',#10275,#10275,#9245,.T.);
#12746=EDGE_CURVE('',#10275,#10276,#5551,.T.);
#12747=EDGE_CURVE('',#10276,#10276,#9246,.T.);
#12748=EDGE_CURVE('',#10276,#10277,#5552,.T.);
#12749=EDGE_CURVE('',#10277,#10277,#9247,.T.);
#12750=EDGE_CURVE('',#10278,#10278,#9248,.T.);
#12751=EDGE_CURVE('',#10278,#10279,#5553,.T.);
#12752=EDGE_CURVE('',#10279,#10279,#9249,.T.);
#12753=EDGE_CURVE('',#10280,#10280,#9250,.T.);
#12754=EDGE_CURVE('',#10280,#10281,#5554,.T.);
#12755=EDGE_CURVE('',#10281,#10281,#9251,.T.);
#12756=EDGE_CURVE('',#10281,#10282,#5555,.T.);
#12757=EDGE_CURVE('',#10282,#10282,#9252,.T.);
#12758=EDGE_CURVE('',#10282,#10283,#5556,.T.);
#12759=EDGE_CURVE('',#10283,#10283,#9253,.T.);
#12760=EDGE_CURVE('',#10284,#10284,#9254,.T.);
#12761=EDGE_CURVE('',#10284,#10285,#5557,.T.);
#12762=EDGE_CURVE('',#10285,#10285,#9255,.T.);
#12763=EDGE_CURVE('',#10286,#10286,#9256,.T.);
#12764=EDGE_CURVE('',#10286,#10287,#5558,.T.);
#12765=EDGE_CURVE('',#10287,#10287,#9257,.T.);
#12766=EDGE_CURVE('',#10287,#10288,#5559,.T.);
#12767=EDGE_CURVE('',#10288,#10288,#9258,.T.);
#12768=EDGE_CURVE('',#10288,#10289,#5560,.T.);
#12769=EDGE_CURVE('',#10289,#10289,#9259,.T.);
#12770=EDGE_CURVE('',#10290,#10290,#9260,.T.);
#12771=EDGE_CURVE('',#10290,#10291,#5561,.T.);
#12772=EDGE_CURVE('',#10291,#10291,#9261,.T.);
#12773=EDGE_CURVE('',#10292,#10292,#9262,.T.);
#12774=EDGE_CURVE('',#10292,#10293,#5562,.T.);
#12775=EDGE_CURVE('',#10293,#10294,#9263,.T.);
#12776=EDGE_CURVE('',#10294,#10293,#9264,.T.);
#12777=EDGE_CURVE('',#10295,#10296,#9265,.T.);
#12778=EDGE_CURVE('',#10296,#10295,#9266,.T.);
#12779=EDGE_CURVE('',#10296,#10294,#5563,.T.);
#12780=EDGE_CURVE('',#10297,#10297,#9267,.T.);
#12781=EDGE_CURVE('',#10295,#10298,#5564,.T.);
#12782=EDGE_CURVE('',#10298,#10298,#9268,.T.);
#12783=EDGE_CURVE('',#10299,#10299,#9269,.T.);
#12784=EDGE_CURVE('',#10300,#10301,#9270,.T.);
#12785=EDGE_CURVE('',#10301,#10300,#9271,.T.);
#12786=EDGE_CURVE('',#10300,#10302,#5565,.T.);
#12787=EDGE_CURVE('',#10302,#10302,#9272,.T.);
#12788=EDGE_CURVE('',#10303,#10304,#9273,.T.);
#12789=EDGE_CURVE('',#10304,#10303,#9274,.T.);
#12790=EDGE_CURVE('',#10304,#10301,#5566,.T.);
#12791=EDGE_CURVE('',#10305,#10305,#9275,.T.);
#12792=EDGE_CURVE('',#10306,#10306,#9276,.T.);
#12793=EDGE_CURVE('',#10306,#10303,#5567,.T.);
#12794=EDGE_CURVE('',#10307,#10308,#5568,.T.);
#12795=EDGE_CURVE('',#10309,#10308,#9277,.T.);
#12796=EDGE_CURVE('',#10309,#10310,#5569,.T.);
#12797=EDGE_CURVE('',#10311,#10310,#9278,.T.);
#12798=EDGE_CURVE('',#10311,#10307,#9279,.F.);
#12799=EDGE_CURVE('',#10312,#10313,#9280,.T.);
#12800=EDGE_CURVE('',#10312,#10314,#5570,.T.);
#12801=EDGE_CURVE('',#10315,#10314,#9281,.T.);
#12802=EDGE_CURVE('',#10315,#10316,#5571,.T.);
#12803=EDGE_CURVE('',#10316,#10313,#9282,.F.);
#12804=EDGE_CURVE('',#10317,#10318,#5572,.T.);
#12805=EDGE_CURVE('',#10319,#10318,#9283,.T.);
#12806=EDGE_CURVE('',#10319,#10320,#5573,.T.);
#12807=EDGE_CURVE('',#10320,#10321,#9284,.F.);
#12808=EDGE_CURVE('',#10317,#10321,#9285,.T.);
#12809=EDGE_CURVE('',#10322,#10323,#9286,.T.);
#12810=EDGE_CURVE('',#10322,#10324,#9287,.F.);
#12811=EDGE_CURVE('',#10324,#10325,#5574,.T.);
#12812=EDGE_CURVE('',#10326,#10325,#9288,.T.);
#12813=EDGE_CURVE('',#10326,#10323,#5575,.T.);
#12814=EDGE_CURVE('',#10327,#10328,#5576,.T.);
#12815=EDGE_CURVE('',#10329,#10328,#9289,.T.);
#12816=EDGE_CURVE('',#10329,#10330,#5577,.T.);
#12817=EDGE_CURVE('',#10331,#10330,#9290,.T.);
#12818=EDGE_CURVE('',#10331,#10327,#9291,.F.);
#12819=EDGE_CURVE('',#10332,#10333,#9292,.T.);
#12820=EDGE_CURVE('',#10332,#10334,#5578,.T.);
#12821=EDGE_CURVE('',#10335,#10334,#9293,.T.);
#12822=EDGE_CURVE('',#10335,#10336,#5579,.T.);
#12823=EDGE_CURVE('',#10336,#10333,#9294,.F.);
#12824=EDGE_CURVE('',#10337,#10338,#5580,.T.);
#12825=EDGE_CURVE('',#10339,#10338,#9295,.T.);
#12826=EDGE_CURVE('',#10339,#10340,#5581,.T.);
#12827=EDGE_CURVE('',#10340,#10341,#9296,.F.);
#12828=EDGE_CURVE('',#10337,#10341,#9297,.T.);
#12829=EDGE_CURVE('',#10342,#10343,#9298,.T.);
#12830=EDGE_CURVE('',#10342,#10344,#9299,.F.);
#12831=EDGE_CURVE('',#10344,#10345,#5582,.T.);
#12832=EDGE_CURVE('',#10346,#10345,#9300,.T.);
#12833=EDGE_CURVE('',#10346,#10343,#5583,.T.);
#12834=EDGE_CURVE('',#10347,#10348,#5584,.T.);
#12835=EDGE_CURVE('',#10349,#10348,#9301,.T.);
#12836=EDGE_CURVE('',#10349,#10350,#5585,.T.);
#12837=EDGE_CURVE('',#10351,#10350,#9302,.T.);
#12838=EDGE_CURVE('',#10351,#10347,#9303,.F.);
#12839=EDGE_CURVE('',#10352,#10353,#9304,.T.);
#12840=EDGE_CURVE('',#10352,#10354,#5586,.T.);
#12841=EDGE_CURVE('',#10355,#10354,#9305,.T.);
#12842=EDGE_CURVE('',#10355,#10356,#5587,.T.);
#12843=EDGE_CURVE('',#10356,#10353,#9306,.F.);
#12844=EDGE_CURVE('',#10357,#10358,#5588,.T.);
#12845=EDGE_CURVE('',#10359,#10358,#9307,.T.);
#12846=EDGE_CURVE('',#10359,#10360,#5589,.T.);
#12847=EDGE_CURVE('',#10360,#10361,#9308,.F.);
#12848=EDGE_CURVE('',#10357,#10361,#9309,.T.);
#12849=EDGE_CURVE('',#10362,#10363,#9310,.T.);
#12850=EDGE_CURVE('',#10362,#10364,#9311,.F.);
#12851=EDGE_CURVE('',#10364,#10365,#5590,.T.);
#12852=EDGE_CURVE('',#10366,#10365,#9312,.T.);
#12853=EDGE_CURVE('',#10366,#10363,#5591,.T.);
#12854=EDGE_CURVE('',#10367,#10368,#5592,.T.);
#12855=EDGE_CURVE('',#10369,#10368,#9313,.T.);
#12856=EDGE_CURVE('',#10369,#10370,#5593,.T.);
#12857=EDGE_CURVE('',#10371,#10370,#9314,.T.);
#12858=EDGE_CURVE('',#10371,#10372,#5594,.T.);
#12859=EDGE_CURVE('',#10367,#10372,#9315,.T.);
#12860=EDGE_CURVE('',#10373,#10374,#5595,.T.);
#12861=EDGE_CURVE('',#10375,#10374,#9316,.T.);
#12862=EDGE_CURVE('',#10375,#10376,#5596,.T.);
#12863=EDGE_CURVE('',#10377,#10376,#9317,.T.);
#12864=EDGE_CURVE('',#10377,#10378,#5597,.T.);
#12865=EDGE_CURVE('',#10373,#10378,#9318,.T.);
#12866=EDGE_CURVE('',#10379,#10380,#5598,.T.);
#12867=EDGE_CURVE('',#10381,#10380,#9319,.T.);
#12868=EDGE_CURVE('',#10381,#10382,#5599,.T.);
#12869=EDGE_CURVE('',#10383,#10382,#9320,.T.);
#12870=EDGE_CURVE('',#10383,#10384,#5600,.T.);
#12871=EDGE_CURVE('',#10379,#10384,#9321,.T.);
#12872=EDGE_CURVE('',#10385,#10386,#5601,.T.);
#12873=EDGE_CURVE('',#10387,#10386,#9322,.T.);
#12874=EDGE_CURVE('',#10387,#10388,#5602,.T.);
#12875=EDGE_CURVE('',#10389,#10388,#9323,.T.);
#12876=EDGE_CURVE('',#10389,#10390,#5603,.T.);
#12877=EDGE_CURVE('',#10385,#10390,#9324,.T.);
#12878=EDGE_CURVE('',#10391,#10392,#5604,.T.);
#12879=EDGE_CURVE('',#10393,#10392,#9325,.T.);
#12880=EDGE_CURVE('',#10393,#10394,#5605,.T.);
#12881=EDGE_CURVE('',#10395,#10394,#9326,.T.);
#12882=EDGE_CURVE('',#10395,#10396,#5606,.T.);
#12883=EDGE_CURVE('',#10391,#10396,#9327,.T.);
#12884=EDGE_CURVE('',#10397,#10398,#5607,.T.);
#12885=EDGE_CURVE('',#10399,#10398,#9328,.T.);
#12886=EDGE_CURVE('',#10399,#10400,#5608,.T.);
#12887=EDGE_CURVE('',#10401,#10400,#9329,.T.);
#12888=EDGE_CURVE('',#10401,#10402,#5609,.T.);
#12889=EDGE_CURVE('',#10397,#10402,#9330,.T.);
#12890=EDGE_CURVE('',#10403,#10404,#5610,.T.);
#12891=EDGE_CURVE('',#10405,#10404,#9331,.T.);
#12892=EDGE_CURVE('',#10405,#10406,#5611,.T.);
#12893=EDGE_CURVE('',#10407,#10406,#9332,.T.);
#12894=EDGE_CURVE('',#10407,#10408,#5612,.T.);
#12895=EDGE_CURVE('',#10403,#10408,#9333,.T.);
#12896=EDGE_CURVE('',#10409,#10410,#5613,.T.);
#12897=EDGE_CURVE('',#10411,#10410,#9334,.T.);
#12898=EDGE_CURVE('',#10411,#10412,#5614,.T.);
#12899=EDGE_CURVE('',#10413,#10412,#9335,.T.);
#12900=EDGE_CURVE('',#10413,#10414,#5615,.T.);
#12901=EDGE_CURVE('',#10409,#10414,#9336,.T.);
#12902=EDGE_CURVE('',#10415,#10416,#5616,.T.);
#12903=EDGE_CURVE('',#10417,#10416,#9337,.T.);
#12904=EDGE_CURVE('',#10417,#10418,#5617,.T.);
#12905=EDGE_CURVE('',#10419,#10418,#9338,.T.);
#12906=EDGE_CURVE('',#10419,#10420,#5618,.T.);
#12907=EDGE_CURVE('',#10415,#10420,#9339,.T.);
#12908=EDGE_CURVE('',#10421,#10422,#5619,.T.);
#12909=EDGE_CURVE('',#10423,#10422,#9340,.T.);
#12910=EDGE_CURVE('',#10423,#10424,#5620,.T.);
#12911=EDGE_CURVE('',#10425,#10424,#9341,.T.);
#12912=EDGE_CURVE('',#10425,#10426,#5621,.T.);
#12913=EDGE_CURVE('',#10421,#10426,#9342,.T.);
#12914=EDGE_CURVE('',#10427,#10428,#5622,.T.);
#12915=EDGE_CURVE('',#10429,#10428,#9343,.T.);
#12916=EDGE_CURVE('',#10429,#10430,#5623,.T.);
#12917=EDGE_CURVE('',#10431,#10430,#9344,.T.);
#12918=EDGE_CURVE('',#10431,#10432,#5624,.T.);
#12919=EDGE_CURVE('',#10427,#10432,#9345,.T.);
#12920=EDGE_CURVE('',#10433,#10434,#5625,.T.);
#12921=EDGE_CURVE('',#10435,#10434,#9346,.T.);
#12922=EDGE_CURVE('',#10435,#10436,#5626,.T.);
#12923=EDGE_CURVE('',#10437,#10436,#9347,.T.);
#12924=EDGE_CURVE('',#10437,#10438,#5627,.T.);
#12925=EDGE_CURVE('',#10433,#10438,#9348,.T.);
#12926=EDGE_CURVE('',#10439,#10440,#5628,.T.);
#12927=EDGE_CURVE('',#10441,#10440,#9349,.T.);
#12928=EDGE_CURVE('',#10441,#10442,#5629,.T.);
#12929=EDGE_CURVE('',#10443,#10442,#9350,.T.);
#12930=EDGE_CURVE('',#10443,#10444,#5630,.T.);
#12931=EDGE_CURVE('',#10439,#10444,#9351,.T.);
#12932=EDGE_CURVE('',#10445,#10446,#5631,.T.);
#12933=EDGE_CURVE('',#10447,#10446,#9352,.T.);
#12934=EDGE_CURVE('',#10447,#10448,#5632,.T.);
#12935=EDGE_CURVE('',#10449,#10448,#9353,.T.);
#12936=EDGE_CURVE('',#10449,#10450,#5633,.T.);
#12937=EDGE_CURVE('',#10445,#10450,#9354,.T.);
#12938=EDGE_CURVE('',#10451,#10452,#5634,.T.);
#12939=EDGE_CURVE('',#10453,#10452,#9355,.T.);
#12940=EDGE_CURVE('',#10453,#10454,#5635,.T.);
#12941=EDGE_CURVE('',#10455,#10454,#9356,.T.);
#12942=EDGE_CURVE('',#10455,#10456,#5636,.T.);
#12943=EDGE_CURVE('',#10451,#10456,#9357,.T.);
#12944=EDGE_CURVE('',#10457,#10458,#5637,.T.);
#12945=EDGE_CURVE('',#10459,#10458,#9358,.T.);
#12946=EDGE_CURVE('',#10459,#10460,#5638,.T.);
#12947=EDGE_CURVE('',#10461,#10460,#9359,.T.);
#12948=EDGE_CURVE('',#10461,#10462,#5639,.T.);
#12949=EDGE_CURVE('',#10457,#10462,#9360,.T.);
#12950=EDGE_CURVE('',#10463,#10464,#5640,.T.);
#12951=EDGE_CURVE('',#10465,#10464,#9361,.T.);
#12952=EDGE_CURVE('',#10465,#10466,#5641,.T.);
#12953=EDGE_CURVE('',#10467,#10466,#9362,.T.);
#12954=EDGE_CURVE('',#10467,#10468,#5642,.T.);
#12955=EDGE_CURVE('',#10463,#10468,#9363,.T.);
#12956=EDGE_CURVE('',#10469,#10470,#5643,.T.);
#12957=EDGE_CURVE('',#10471,#10470,#9364,.T.);
#12958=EDGE_CURVE('',#10471,#10472,#5644,.T.);
#12959=EDGE_CURVE('',#10473,#10472,#9365,.T.);
#12960=EDGE_CURVE('',#10473,#10474,#5645,.T.);
#12961=EDGE_CURVE('',#10469,#10474,#9366,.T.);
#12962=EDGE_CURVE('',#10475,#10475,#9367,.T.);
#12963=EDGE_CURVE('',#10360,#10476,#5646,.T.);
#12964=EDGE_CURVE('',#10477,#10476,#9368,.T.);
#12965=EDGE_CURVE('',#10477,#10361,#5647,.T.);
#12966=EDGE_CURVE('',#10478,#10479,#9369,.T.);
#12967=EDGE_CURVE('',#10478,#10366,#5648,.T.);
#12968=EDGE_CURVE('',#10365,#10479,#5649,.T.);
#12969=EDGE_CURVE('',#10478,#10480,#5650,.T.);
#12970=EDGE_CURVE('',#10480,#10363,#5651,.T.);
#12971=EDGE_CURVE('',#10481,#10482,#9370,.T.);
#12972=EDGE_CURVE('',#10481,#10364,#5652,.T.);
#12973=EDGE_CURVE('',#10362,#10482,#5653,.T.);
#12974=EDGE_CURVE('',#10481,#10479,#5654,.T.);
#12975=EDGE_CURVE('',#10482,#10480,#9371,.T.);
#12976=EDGE_CURVE('',#10483,#10484,#9372,.T.);
#12977=EDGE_CURVE('',#10483,#10473,#5655,.T.);
#12978=EDGE_CURVE('',#10472,#10484,#5656,.T.);
#12979=EDGE_CURVE('',#10483,#10485,#5657,.T.);
#12980=EDGE_CURVE('',#10474,#10485,#5658,.T.);
#12981=EDGE_CURVE('',#10486,#10487,#9373,.T.);
#12982=EDGE_CURVE('',#10486,#10471,#5659,.T.);
#12983=EDGE_CURVE('',#10470,#10487,#5660,.T.);
#12984=EDGE_CURVE('',#10486,#10484,#5661,.T.);
#12985=EDGE_CURVE('',#10488,#10487,#5662,.T.);
#12986=EDGE_CURVE('',#10488,#10485,#9374,.T.);
#12987=EDGE_CURVE('',#10488,#10469,#5663,.T.);
#12988=EDGE_CURVE('',#10489,#10490,#9375,.T.);
#12989=EDGE_CURVE('',#10489,#10467,#5664,.T.);
#12990=EDGE_CURVE('',#10466,#10490,#5665,.T.);
#12991=EDGE_CURVE('',#10489,#10491,#5666,.T.);
#12992=EDGE_CURVE('',#10468,#10491,#5667,.T.);
#12993=EDGE_CURVE('',#10492,#10493,#9376,.T.);
#12994=EDGE_CURVE('',#10492,#10465,#5668,.T.);
#12995=EDGE_CURVE('',#10464,#10493,#5669,.T.);
#12996=EDGE_CURVE('',#10492,#10490,#5670,.T.);
#12997=EDGE_CURVE('',#10494,#10493,#5671,.T.);
#12998=EDGE_CURVE('',#10494,#10491,#9377,.T.);
#12999=EDGE_CURVE('',#10494,#10463,#5672,.T.);
#13000=EDGE_CURVE('',#10340,#10495,#5673,.T.);
#13001=EDGE_CURVE('',#10496,#10495,#9378,.T.);
#13002=EDGE_CURVE('',#10496,#10341,#5674,.T.);
#13003=EDGE_CURVE('',#10497,#10498,#9379,.T.);
#13004=EDGE_CURVE('',#10497,#10461,#5675,.T.);
#13005=EDGE_CURVE('',#10460,#10498,#5676,.T.);
#13006=EDGE_CURVE('',#10497,#10499,#5677,.T.);
#13007=EDGE_CURVE('',#10462,#10499,#5678,.T.);
#13008=EDGE_CURVE('',#10500,#10501,#9380,.T.);
#13009=EDGE_CURVE('',#10500,#10459,#5679,.T.);
#13010=EDGE_CURVE('',#10458,#10501,#5680,.T.);
#13011=EDGE_CURVE('',#10500,#10498,#5681,.T.);
#13012=EDGE_CURVE('',#10502,#10501,#5682,.T.);
#13013=EDGE_CURVE('',#10502,#10499,#9381,.T.);
#13014=EDGE_CURVE('',#10502,#10457,#5683,.T.);
#13015=EDGE_CURVE('',#10503,#10504,#9382,.T.);
#13016=EDGE_CURVE('',#10503,#10455,#5684,.T.);
#13017=EDGE_CURVE('',#10454,#10504,#5685,.T.);
#13018=EDGE_CURVE('',#10503,#10505,#5686,.T.);
#13019=EDGE_CURVE('',#10456,#10505,#5687,.T.);
#13020=EDGE_CURVE('',#10506,#10507,#9383,.T.);
#13021=EDGE_CURVE('',#10506,#10453,#5688,.T.);
#13022=EDGE_CURVE('',#10452,#10507,#5689,.T.);
#13023=EDGE_CURVE('',#10506,#10504,#5690,.T.);
#13024=EDGE_CURVE('',#10508,#10507,#5691,.T.);
#13025=EDGE_CURVE('',#10508,#10505,#9384,.T.);
#13026=EDGE_CURVE('',#10508,#10451,#5692,.T.);
#13027=EDGE_CURVE('',#10509,#10510,#9385,.T.);
#13028=EDGE_CURVE('',#10509,#10329,#5693,.T.);
#13029=EDGE_CURVE('',#10328,#10510,#5694,.T.);
#13030=EDGE_CURVE('',#10509,#10511,#5695,.T.);
#13031=EDGE_CURVE('',#10511,#10330,#5696,.T.);
#13032=EDGE_CURVE('',#10512,#10513,#9386,.T.);
#13033=EDGE_CURVE('',#10512,#10346,#5697,.T.);
#13034=EDGE_CURVE('',#10345,#10513,#5698,.T.);
#13035=EDGE_CURVE('',#10514,#10513,#5699,.T.);
#13036=EDGE_CURVE('',#10514,#10515,#9387,.T.);
#13037=EDGE_CURVE('',#10515,#10516,#9388,.T.);
#13038=EDGE_CURVE('',#10512,#10516,#5700,.T.);
#13039=EDGE_CURVE('',#10514,#10344,#5701,.T.);
#13040=EDGE_CURVE('',#10342,#10515,#5702,.T.);
#13041=EDGE_CURVE('',#10517,#10518,#9389,.T.);
#13042=EDGE_CURVE('',#10517,#10449,#5703,.T.);
#13043=EDGE_CURVE('',#10448,#10518,#5704,.T.);
#13044=EDGE_CURVE('',#10517,#10519,#5705,.T.);
#13045=EDGE_CURVE('',#10450,#10519,#5706,.T.);
#13046=EDGE_CURVE('',#10520,#10521,#9390,.T.);
#13047=EDGE_CURVE('',#10520,#10447,#5707,.T.);
#13048=EDGE_CURVE('',#10446,#10521,#5708,.T.);
#13049=EDGE_CURVE('',#10520,#10518,#5709,.T.);
#13050=EDGE_CURVE('',#10522,#10521,#5710,.T.);
#13051=EDGE_CURVE('',#10522,#10519,#9391,.T.);
#13052=EDGE_CURVE('',#10522,#10445,#5711,.T.);
#13053=EDGE_CURVE('',#10523,#10524,#9392,.T.);
#13054=EDGE_CURVE('',#10523,#10443,#5712,.T.);
#13055=EDGE_CURVE('',#10442,#10524,#5713,.T.);
#13056=EDGE_CURVE('',#10523,#10525,#5714,.T.);
#13057=EDGE_CURVE('',#10444,#10525,#5715,.T.);
#13058=EDGE_CURVE('',#10526,#10527,#9393,.T.);
#13059=EDGE_CURVE('',#10526,#10441,#5716,.T.);
#13060=EDGE_CURVE('',#10440,#10527,#5717,.T.);
#13061=EDGE_CURVE('',#10526,#10524,#5718,.T.);
#13062=EDGE_CURVE('',#10528,#10527,#5719,.T.);
#13063=EDGE_CURVE('',#10528,#10525,#9394,.T.);
#13064=EDGE_CURVE('',#10528,#10439,#5720,.T.);
#13065=EDGE_CURVE('',#10336,#10529,#5721,.T.);
#13066=EDGE_CURVE('',#10530,#10529,#9395,.T.);
#13067=EDGE_CURVE('',#10530,#10333,#5722,.T.);
#13068=EDGE_CURVE('',#10531,#10529,#5723,.T.);
#13069=EDGE_CURVE('',#10531,#10532,#9396,.T.);
#13070=EDGE_CURVE('',#10533,#10532,#5724,.T.);
#13071=EDGE_CURVE('',#10533,#10530,#9397,.T.);
#13072=EDGE_CURVE('',#10531,#10335,#5725,.T.);
#13073=EDGE_CURVE('',#10334,#10532,#5726,.T.);
#13074=EDGE_CURVE('',#10332,#10533,#5727,.T.);
#13075=EDGE_CURVE('',#10534,#10535,#9398,.T.);
#13076=EDGE_CURVE('',#10534,#10437,#5728,.T.);
#13077=EDGE_CURVE('',#10436,#10535,#5729,.T.);
#13078=EDGE_CURVE('',#10534,#10536,#5730,.T.);
#13079=EDGE_CURVE('',#10438,#10536,#5731,.T.);
#13080=EDGE_CURVE('',#10537,#10538,#9399,.T.);
#13081=EDGE_CURVE('',#10537,#10435,#5732,.T.);
#13082=EDGE_CURVE('',#10434,#10538,#5733,.T.);
#13083=EDGE_CURVE('',#10537,#10535,#5734,.T.);
#13084=EDGE_CURVE('',#10539,#10538,#5735,.T.);
#13085=EDGE_CURVE('',#10539,#10536,#9400,.T.);
#13086=EDGE_CURVE('',#10539,#10433,#5736,.T.);
#13087=EDGE_CURVE('',#10540,#10541,#9401,.T.);
#13088=EDGE_CURVE('',#10540,#10431,#5737,.T.);
#13089=EDGE_CURVE('',#10430,#10541,#5738,.T.);
#13090=EDGE_CURVE('',#10540,#10542,#5739,.T.);
#13091=EDGE_CURVE('',#10432,#10542,#5740,.T.);
#13092=EDGE_CURVE('',#10543,#10544,#9402,.T.);
#13093=EDGE_CURVE('',#10543,#10429,#5741,.T.);
#13094=EDGE_CURVE('',#10428,#10544,#5742,.T.);
#13095=EDGE_CURVE('',#10543,#10541,#5743,.T.);
#13096=EDGE_CURVE('',#10545,#10544,#5744,.T.);
#13097=EDGE_CURVE('',#10545,#10542,#9403,.T.);
#13098=EDGE_CURVE('',#10545,#10427,#5745,.T.);
#13099=EDGE_CURVE('',#10546,#10547,#9404,.T.);
#13100=EDGE_CURVE('',#10546,#10309,#5746,.T.);
#13101=EDGE_CURVE('',#10308,#10547,#5747,.T.);
#13102=EDGE_CURVE('',#10546,#10548,#5748,.T.);
#13103=EDGE_CURVE('',#10548,#10310,#5749,.T.);
#13104=EDGE_CURVE('',#10549,#10550,#9405,.T.);
#13105=EDGE_CURVE('',#10549,#10326,#5750,.T.);
#13106=EDGE_CURVE('',#10325,#10550,#5751,.T.);
#13107=EDGE_CURVE('',#10551,#10550,#5752,.T.);
#13108=EDGE_CURVE('',#10551,#10552,#9406,.T.);
#13109=EDGE_CURVE('',#10552,#10553,#9407,.T.);
#13110=EDGE_CURVE('',#10549,#10553,#5753,.T.);
#13111=EDGE_CURVE('',#10551,#10324,#5754,.T.);
#13112=EDGE_CURVE('',#10322,#10552,#5755,.T.);
#13113=EDGE_CURVE('',#10554,#10555,#9408,.T.);
#13114=EDGE_CURVE('',#10554,#10425,#5756,.T.);
#13115=EDGE_CURVE('',#10424,#10555,#5757,.T.);
#13116=EDGE_CURVE('',#10554,#10556,#5758,.T.);
#13117=EDGE_CURVE('',#10426,#10556,#5759,.T.);
#13118=EDGE_CURVE('',#10557,#10558,#9409,.T.);
#13119=EDGE_CURVE('',#10557,#10423,#5760,.T.);
#13120=EDGE_CURVE('',#10422,#10558,#5761,.T.);
#13121=EDGE_CURVE('',#10557,#10555,#5762,.T.);
#13122=EDGE_CURVE('',#10559,#10558,#5763,.T.);
#13123=EDGE_CURVE('',#10559,#10556,#9410,.T.);
#13124=EDGE_CURVE('',#10559,#10421,#5764,.T.);
#13125=EDGE_CURVE('',#10560,#10561,#9411,.T.);
#13126=EDGE_CURVE('',#10560,#10419,#5765,.T.);
#13127=EDGE_CURVE('',#10418,#10561,#5766,.T.);
#13128=EDGE_CURVE('',#10560,#10562,#5767,.T.);
#13129=EDGE_CURVE('',#10420,#10562,#5768,.T.);
#13130=EDGE_CURVE('',#10563,#10564,#9412,.T.);
#13131=EDGE_CURVE('',#10563,#10417,#5769,.T.);
#13132=EDGE_CURVE('',#10416,#10564,#5770,.T.);
#13133=EDGE_CURVE('',#10563,#10561,#5771,.T.);
#13134=EDGE_CURVE('',#10565,#10564,#5772,.T.);
#13135=EDGE_CURVE('',#10565,#10562,#9413,.T.);
#13136=EDGE_CURVE('',#10565,#10415,#5773,.T.);
#13137=EDGE_CURVE('',#10566,#10567,#9414,.T.);
#13138=EDGE_CURVE('',#10566,#10413,#5774,.T.);
#13139=EDGE_CURVE('',#10412,#10567,#5775,.T.);
#13140=EDGE_CURVE('',#10566,#10568,#5776,.T.);
#13141=EDGE_CURVE('',#10414,#10568,#5777,.T.);
#13142=EDGE_CURVE('',#10569,#10570,#9415,.T.);
#13143=EDGE_CURVE('',#10569,#10411,#5778,.T.);
#13144=EDGE_CURVE('',#10410,#10570,#5779,.T.);
#13145=EDGE_CURVE('',#10569,#10567,#5780,.T.);
#13146=EDGE_CURVE('',#10571,#10570,#5781,.T.);
#13147=EDGE_CURVE('',#10571,#10568,#9416,.T.);
#13148=EDGE_CURVE('',#10571,#10409,#5782,.T.);
#13149=EDGE_CURVE('',#10320,#10572,#5783,.T.);
#13150=EDGE_CURVE('',#10573,#10572,#9417,.T.);
#13151=EDGE_CURVE('',#10573,#10321,#5784,.T.);
#13152=EDGE_CURVE('',#10574,#10575,#9418,.T.);
#13153=EDGE_CURVE('',#10574,#10407,#5785,.T.);
#13154=EDGE_CURVE('',#10406,#10575,#5786,.T.);
#13155=EDGE_CURVE('',#10574,#10576,#5787,.T.);
#13156=EDGE_CURVE('',#10408,#10576,#5788,.T.);
#13157=EDGE_CURVE('',#10577,#10578,#9419,.T.);
#13158=EDGE_CURVE('',#10577,#10405,#5789,.T.);
#13159=EDGE_CURVE('',#10404,#10578,#5790,.T.);
#13160=EDGE_CURVE('',#10577,#10575,#5791,.T.);
#13161=EDGE_CURVE('',#10579,#10578,#5792,.T.);
#13162=EDGE_CURVE('',#10579,#10576,#9420,.T.);
#13163=EDGE_CURVE('',#10579,#10403,#5793,.T.);
#13164=EDGE_CURVE('',#10580,#10581,#9421,.T.);
#13165=EDGE_CURVE('',#10580,#10401,#5794,.T.);
#13166=EDGE_CURVE('',#10400,#10581,#5795,.T.);
#13167=EDGE_CURVE('',#10580,#10582,#5796,.T.);
#13168=EDGE_CURVE('',#10402,#10582,#5797,.T.);
#13169=EDGE_CURVE('',#10583,#10584,#9422,.T.);
#13170=EDGE_CURVE('',#10583,#10399,#5798,.T.);
#13171=EDGE_CURVE('',#10398,#10584,#5799,.T.);
#13172=EDGE_CURVE('',#10583,#10581,#5800,.T.);
#13173=EDGE_CURVE('',#10585,#10584,#5801,.T.);
#13174=EDGE_CURVE('',#10585,#10582,#9423,.T.);
#13175=EDGE_CURVE('',#10585,#10397,#5802,.T.);
#13176=EDGE_CURVE('',#10316,#10586,#5803,.T.);
#13177=EDGE_CURVE('',#10587,#10586,#9424,.T.);
#13178=EDGE_CURVE('',#10587,#10313,#5804,.T.);
#13179=EDGE_CURVE('',#10588,#10586,#5805,.T.);
#13180=EDGE_CURVE('',#10588,#10589,#9425,.T.);
#13181=EDGE_CURVE('',#10590,#10589,#5806,.T.);
#13182=EDGE_CURVE('',#10590,#10587,#9426,.T.);
#13183=EDGE_CURVE('',#10588,#10315,#5807,.T.);
#13184=EDGE_CURVE('',#10314,#10589,#5808,.T.);
#13185=EDGE_CURVE('',#10312,#10590,#5809,.T.);
#13186=EDGE_CURVE('',#10591,#10592,#9427,.T.);
#13187=EDGE_CURVE('',#10591,#10395,#5810,.T.);
#13188=EDGE_CURVE('',#10394,#10592,#5811,.T.);
#13189=EDGE_CURVE('',#10591,#10593,#5812,.T.);
#13190=EDGE_CURVE('',#10396,#10593,#5813,.T.);
#13191=EDGE_CURVE('',#10594,#10595,#9428,.T.);
#13192=EDGE_CURVE('',#10594,#10393,#5814,.T.);
#13193=EDGE_CURVE('',#10392,#10595,#5815,.T.);
#13194=EDGE_CURVE('',#10594,#10592,#5816,.T.);
#13195=EDGE_CURVE('',#10596,#10595,#5817,.T.);
#13196=EDGE_CURVE('',#10596,#10593,#9429,.T.);
#13197=EDGE_CURVE('',#10596,#10391,#5818,.T.);
#13198=EDGE_CURVE('',#10597,#10598,#9430,.T.);
#13199=EDGE_CURVE('',#10597,#10389,#5819,.T.);
#13200=EDGE_CURVE('',#10388,#10598,#5820,.T.);
#13201=EDGE_CURVE('',#10597,#10599,#5821,.T.);
#13202=EDGE_CURVE('',#10390,#10599,#5822,.T.);
#13203=EDGE_CURVE('',#10600,#10601,#9431,.T.);
#13204=EDGE_CURVE('',#10600,#10387,#5823,.T.);
#13205=EDGE_CURVE('',#10386,#10601,#5824,.T.);
#13206=EDGE_CURVE('',#10600,#10598,#5825,.T.);
#13207=EDGE_CURVE('',#10602,#10601,#5826,.T.);
#13208=EDGE_CURVE('',#10602,#10599,#9432,.T.);
#13209=EDGE_CURVE('',#10602,#10385,#5827,.T.);
#13210=EDGE_CURVE('',#10356,#10603,#5828,.T.);
#13211=EDGE_CURVE('',#10604,#10603,#9433,.T.);
#13212=EDGE_CURVE('',#10604,#10353,#5829,.T.);
#13213=EDGE_CURVE('',#10605,#10606,#9434,.T.);
#13214=EDGE_CURVE('',#10605,#10355,#5830,.T.);
#13215=EDGE_CURVE('',#10354,#10606,#5831,.T.);
#13216=EDGE_CURVE('',#10605,#10603,#5832,.T.);
#13217=EDGE_CURVE('',#10607,#10606,#5833,.T.);
#13218=EDGE_CURVE('',#10607,#10604,#9435,.T.);
#13219=EDGE_CURVE('',#10352,#10607,#5834,.T.);
#13220=EDGE_CURVE('',#10608,#10609,#9436,.T.);
#13221=EDGE_CURVE('',#10608,#10383,#5835,.T.);
#13222=EDGE_CURVE('',#10382,#10609,#5836,.T.);
#13223=EDGE_CURVE('',#10608,#10610,#5837,.T.);
#13224=EDGE_CURVE('',#10384,#10610,#5838,.T.);
#13225=EDGE_CURVE('',#10611,#10612,#9437,.T.);
#13226=EDGE_CURVE('',#10611,#10381,#5839,.T.);
#13227=EDGE_CURVE('',#10380,#10612,#5840,.T.);
#13228=EDGE_CURVE('',#10611,#10609,#5841,.T.);
#13229=EDGE_CURVE('',#10613,#10612,#5842,.T.);
#13230=EDGE_CURVE('',#10613,#10610,#9438,.T.);
#13231=EDGE_CURVE('',#10613,#10379,#5843,.T.);
#13232=EDGE_CURVE('',#10614,#10615,#9439,.T.);
#13233=EDGE_CURVE('',#10614,#10377,#5844,.T.);
#13234=EDGE_CURVE('',#10376,#10615,#5845,.T.);
#13235=EDGE_CURVE('',#10614,#10616,#5846,.T.);
#13236=EDGE_CURVE('',#10378,#10616,#5847,.T.);
#13237=EDGE_CURVE('',#10617,#10618,#9440,.T.);
#13238=EDGE_CURVE('',#10617,#10375,#5848,.T.);
#13239=EDGE_CURVE('',#10374,#10618,#5849,.T.);
#13240=EDGE_CURVE('',#10617,#10615,#5850,.T.);
#13241=EDGE_CURVE('',#10619,#10618,#5851,.T.);
#13242=EDGE_CURVE('',#10619,#10616,#9441,.T.);
#13243=EDGE_CURVE('',#10619,#10373,#5852,.T.);
#13244=EDGE_CURVE('',#10620,#10621,#9442,.T.);
#13245=EDGE_CURVE('',#10620,#10371,#5853,.T.);
#13246=EDGE_CURVE('',#10370,#10621,#5854,.T.);
#13247=EDGE_CURVE('',#10620,#10622,#5855,.T.);
#13248=EDGE_CURVE('',#10372,#10622,#5856,.T.);
#13249=EDGE_CURVE('',#10623,#10624,#9443,.T.);
#13250=EDGE_CURVE('',#10623,#10369,#5857,.T.);
#13251=EDGE_CURVE('',#10368,#10624,#5858,.T.);
#13252=EDGE_CURVE('',#10623,#10621,#5859,.T.);
#13253=EDGE_CURVE('',#10625,#10624,#5860,.T.);
#13254=EDGE_CURVE('',#10625,#10622,#9444,.T.);
#13255=EDGE_CURVE('',#10625,#10367,#5861,.T.);
#13256=EDGE_CURVE('',#10626,#10627,#9445,.T.);
#13257=EDGE_CURVE('',#10626,#10359,#5862,.T.);
#13258=EDGE_CURVE('',#10358,#10627,#5863,.T.);
#13259=EDGE_CURVE('',#10626,#10476,#5864,.T.);
#13260=EDGE_CURVE('',#10628,#10627,#5865,.T.);
#13261=EDGE_CURVE('',#10628,#10477,#9446,.T.);
#13262=EDGE_CURVE('',#10357,#10628,#5866,.T.);
#13263=EDGE_CURVE('',#10629,#10630,#9447,.T.);
#13264=EDGE_CURVE('',#10629,#10349,#5867,.T.);
#13265=EDGE_CURVE('',#10348,#10630,#5868,.T.);
#13266=EDGE_CURVE('',#10629,#10631,#5869,.T.);
#13267=EDGE_CURVE('',#10631,#10350,#5870,.T.);
#13268=EDGE_CURVE('',#10632,#10633,#9448,.T.);
#13269=EDGE_CURVE('',#10632,#10347,#5871,.T.);
#13270=EDGE_CURVE('',#10351,#10633,#5872,.T.);
#13271=EDGE_CURVE('',#10632,#10630,#5873,.T.);
#13272=EDGE_CURVE('',#10633,#10631,#9449,.T.);
#13273=EDGE_CURVE('',#10634,#10635,#9450,.T.);
#13274=EDGE_CURVE('',#10634,#10339,#5874,.T.);
#13275=EDGE_CURVE('',#10338,#10635,#5875,.T.);
#13276=EDGE_CURVE('',#10634,#10495,#5876,.T.);
#13277=EDGE_CURVE('',#10636,#10635,#5877,.T.);
#13278=EDGE_CURVE('',#10636,#10496,#9451,.T.);
#13279=EDGE_CURVE('',#10337,#10636,#5878,.T.);
#13280=EDGE_CURVE('',#10637,#10638,#9452,.T.);
#13281=EDGE_CURVE('',#10637,#10327,#5879,.T.);
#13282=EDGE_CURVE('',#10331,#10638,#5880,.T.);
#13283=EDGE_CURVE('',#10637,#10510,#5881,.T.);
#13284=EDGE_CURVE('',#10638,#10511,#9453,.T.);
#13285=EDGE_CURVE('',#10639,#10640,#9454,.T.);
#13286=EDGE_CURVE('',#10639,#10319,#5882,.T.);
#13287=EDGE_CURVE('',#10318,#10640,#5883,.T.);
#13288=EDGE_CURVE('',#10639,#10572,#5884,.T.);
#13289=EDGE_CURVE('',#10641,#10640,#5885,.T.);
#13290=EDGE_CURVE('',#10641,#10573,#9455,.T.);
#13291=EDGE_CURVE('',#10317,#10641,#5886,.T.);
#13292=EDGE_CURVE('',#10642,#10643,#9456,.T.);
#13293=EDGE_CURVE('',#10642,#10307,#5887,.T.);
#13294=EDGE_CURVE('',#10311,#10643,#5888,.T.);
#13295=EDGE_CURVE('',#10642,#10547,#5889,.T.);
#13296=EDGE_CURVE('',#10643,#10548,#9457,.T.);
#13297=EDGE_CURVE('',#10516,#10343,#5890,.T.);
#13298=EDGE_CURVE('',#10553,#10323,#5891,.T.);
#13299=EDGE_CURVE('',#10297,#10644,#5892,.T.);
#13300=EDGE_CURVE('',#10644,#10644,#9458,.T.);
#13301=EDGE_CURVE('',#10645,#10645,#9459,.T.);
#13302=EDGE_CURVE('',#10305,#10645,#5893,.T.);
#13303=EDGE_CURVE('',#10475,#10299,#5894,.T.);
#16430=ORIENTED_EDGE('',*,*,#12623,.T.);
#16431=ORIENTED_EDGE('',*,*,#12624,.T.);
#16432=ORIENTED_EDGE('',*,*,#12623,.F.);
#16433=ORIENTED_EDGE('',*,*,#12624,.F.);
#16434=ORIENTED_EDGE('',*,*,#12625,.T.);
#16435=ORIENTED_EDGE('',*,*,#12626,.T.);
#16436=ORIENTED_EDGE('',*,*,#12625,.F.);
#16437=ORIENTED_EDGE('',*,*,#12626,.F.);
#16438=ORIENTED_EDGE('',*,*,#12627,.T.);
#16439=ORIENTED_EDGE('',*,*,#12628,.F.);
#16440=ORIENTED_EDGE('',*,*,#12627,.F.);
#16441=ORIENTED_EDGE('',*,*,#12629,.T.);
#16442=ORIENTED_EDGE('',*,*,#12630,.T.);
#16443=ORIENTED_EDGE('',*,*,#12629,.F.);
#16444=ORIENTED_EDGE('',*,*,#12630,.F.);
#16445=ORIENTED_EDGE('',*,*,#12631,.T.);
#16446=ORIENTED_EDGE('',*,*,#12632,.T.);
#16447=ORIENTED_EDGE('',*,*,#12631,.F.);
#16448=ORIENTED_EDGE('',*,*,#12632,.F.);
#16449=ORIENTED_EDGE('',*,*,#12633,.T.);
#16450=ORIENTED_EDGE('',*,*,#12634,.F.);
#16451=ORIENTED_EDGE('',*,*,#12633,.F.);
#16452=ORIENTED_EDGE('',*,*,#12635,.T.);
#16453=ORIENTED_EDGE('',*,*,#12636,.T.);
#16454=ORIENTED_EDGE('',*,*,#12635,.F.);
#16455=ORIENTED_EDGE('',*,*,#12636,.F.);
#16456=ORIENTED_EDGE('',*,*,#12637,.T.);
#16457=ORIENTED_EDGE('',*,*,#12638,.T.);
#16458=ORIENTED_EDGE('',*,*,#12637,.F.);
#16459=ORIENTED_EDGE('',*,*,#12638,.F.);
#16460=ORIENTED_EDGE('',*,*,#12639,.T.);
#16461=ORIENTED_EDGE('',*,*,#12640,.F.);
#16462=ORIENTED_EDGE('',*,*,#12639,.F.);
#16463=ORIENTED_EDGE('',*,*,#12641,.T.);
#16464=ORIENTED_EDGE('',*,*,#12642,.T.);
#16465=ORIENTED_EDGE('',*,*,#12641,.F.);
#16466=ORIENTED_EDGE('',*,*,#12642,.F.);
#16467=ORIENTED_EDGE('',*,*,#12643,.T.);
#16468=ORIENTED_EDGE('',*,*,#12644,.T.);
#16469=ORIENTED_EDGE('',*,*,#12643,.F.);
#16470=ORIENTED_EDGE('',*,*,#12644,.F.);
#16471=ORIENTED_EDGE('',*,*,#12645,.T.);
#16472=ORIENTED_EDGE('',*,*,#12646,.F.);
#16473=ORIENTED_EDGE('',*,*,#12645,.F.);
#16474=ORIENTED_EDGE('',*,*,#12647,.T.);
#16475=ORIENTED_EDGE('',*,*,#12648,.T.);
#16476=ORIENTED_EDGE('',*,*,#12647,.F.);
#16477=ORIENTED_EDGE('',*,*,#12648,.F.);
#16478=ORIENTED_EDGE('',*,*,#12649,.T.);
#16479=ORIENTED_EDGE('',*,*,#12650,.T.);
#16480=ORIENTED_EDGE('',*,*,#12649,.F.);
#16481=ORIENTED_EDGE('',*,*,#12650,.F.);
#16482=ORIENTED_EDGE('',*,*,#12651,.T.);
#16483=ORIENTED_EDGE('',*,*,#12652,.F.);
#16484=ORIENTED_EDGE('',*,*,#12651,.F.);
#16485=ORIENTED_EDGE('',*,*,#12653,.F.);
#16486=ORIENTED_EDGE('',*,*,#12654,.T.);
#16487=ORIENTED_EDGE('',*,*,#12655,.T.);
#16488=ORIENTED_EDGE('',*,*,#12654,.F.);
#16489=ORIENTED_EDGE('',*,*,#12655,.F.);
#16490=ORIENTED_EDGE('',*,*,#12656,.T.);
#16491=ORIENTED_EDGE('',*,*,#12657,.T.);
#16492=ORIENTED_EDGE('',*,*,#12656,.F.);
#16493=ORIENTED_EDGE('',*,*,#12657,.F.);
#16494=ORIENTED_EDGE('',*,*,#12658,.T.);
#16495=ORIENTED_EDGE('',*,*,#12659,.T.);
#16496=ORIENTED_EDGE('',*,*,#12658,.F.);
#16497=ORIENTED_EDGE('',*,*,#12660,.T.);
#16498=ORIENTED_EDGE('',*,*,#12659,.F.);
#16499=ORIENTED_EDGE('',*,*,#12660,.F.);
#16500=ORIENTED_EDGE('',*,*,#12661,.T.);
#16501=ORIENTED_EDGE('',*,*,#12662,.F.);
#16502=ORIENTED_EDGE('',*,*,#12661,.F.);
#16503=ORIENTED_EDGE('',*,*,#12663,.F.);
#16504=ORIENTED_EDGE('',*,*,#12664,.T.);
#16505=ORIENTED_EDGE('',*,*,#12665,.T.);
#16506=ORIENTED_EDGE('',*,*,#12664,.F.);
#16507=ORIENTED_EDGE('',*,*,#12665,.F.);
#16508=ORIENTED_EDGE('',*,*,#12666,.T.);
#16509=ORIENTED_EDGE('',*,*,#12667,.T.);
#16510=ORIENTED_EDGE('',*,*,#12666,.F.);
#16511=ORIENTED_EDGE('',*,*,#12667,.F.);
#16512=ORIENTED_EDGE('',*,*,#12668,.T.);
#16513=ORIENTED_EDGE('',*,*,#12669,.T.);
#16514=ORIENTED_EDGE('',*,*,#12668,.F.);
#16515=ORIENTED_EDGE('',*,*,#12670,.T.);
#16516=ORIENTED_EDGE('',*,*,#12669,.F.);
#16517=ORIENTED_EDGE('',*,*,#12670,.F.);
#16518=ORIENTED_EDGE('',*,*,#12671,.T.);
#16519=ORIENTED_EDGE('',*,*,#12672,.F.);
#16520=ORIENTED_EDGE('',*,*,#12671,.F.);
#16521=ORIENTED_EDGE('',*,*,#12673,.F.);
#16522=ORIENTED_EDGE('',*,*,#12674,.T.);
#16523=ORIENTED_EDGE('',*,*,#12675,.T.);
#16524=ORIENTED_EDGE('',*,*,#12674,.F.);
#16525=ORIENTED_EDGE('',*,*,#12675,.F.);
#16526=ORIENTED_EDGE('',*,*,#12676,.T.);
#16527=ORIENTED_EDGE('',*,*,#12677,.T.);
#16528=ORIENTED_EDGE('',*,*,#12676,.F.);
#16529=ORIENTED_EDGE('',*,*,#12677,.F.);
#16530=ORIENTED_EDGE('',*,*,#12678,.T.);
#16531=ORIENTED_EDGE('',*,*,#12679,.T.);
#16532=ORIENTED_EDGE('',*,*,#12678,.F.);
#16533=ORIENTED_EDGE('',*,*,#12680,.T.);
#16534=ORIENTED_EDGE('',*,*,#12679,.F.);
#16535=ORIENTED_EDGE('',*,*,#12680,.F.);
#16536=ORIENTED_EDGE('',*,*,#12681,.T.);
#16537=ORIENTED_EDGE('',*,*,#12682,.F.);
#16538=ORIENTED_EDGE('',*,*,#12681,.F.);
#16539=ORIENTED_EDGE('',*,*,#12683,.F.);
#16540=ORIENTED_EDGE('',*,*,#12684,.T.);
#16541=ORIENTED_EDGE('',*,*,#12685,.T.);
#16542=ORIENTED_EDGE('',*,*,#12684,.F.);
#16543=ORIENTED_EDGE('',*,*,#12685,.F.);
#16544=ORIENTED_EDGE('',*,*,#12686,.T.);
#16545=ORIENTED_EDGE('',*,*,#12687,.T.);
#16546=ORIENTED_EDGE('',*,*,#12686,.F.);
#16547=ORIENTED_EDGE('',*,*,#12687,.F.);
#16548=ORIENTED_EDGE('',*,*,#12688,.T.);
#16549=ORIENTED_EDGE('',*,*,#12689,.T.);
#16550=ORIENTED_EDGE('',*,*,#12688,.F.);
#16551=ORIENTED_EDGE('',*,*,#12690,.T.);
#16552=ORIENTED_EDGE('',*,*,#12689,.F.);
#16553=ORIENTED_EDGE('',*,*,#12690,.F.);
#16554=ORIENTED_EDGE('',*,*,#12691,.T.);
#16555=ORIENTED_EDGE('',*,*,#12692,.F.);
#16556=ORIENTED_EDGE('',*,*,#12691,.F.);
#16557=ORIENTED_EDGE('',*,*,#12693,.F.);
#16558=ORIENTED_EDGE('',*,*,#12694,.T.);
#16559=ORIENTED_EDGE('',*,*,#12695,.T.);
#16560=ORIENTED_EDGE('',*,*,#12694,.F.);
#16561=ORIENTED_EDGE('',*,*,#12695,.F.);
#16562=ORIENTED_EDGE('',*,*,#12696,.T.);
#16563=ORIENTED_EDGE('',*,*,#12697,.T.);
#16564=ORIENTED_EDGE('',*,*,#12696,.F.);
#16565=ORIENTED_EDGE('',*,*,#12697,.F.);
#16566=ORIENTED_EDGE('',*,*,#12698,.T.);
#16567=ORIENTED_EDGE('',*,*,#12699,.T.);
#16568=ORIENTED_EDGE('',*,*,#12698,.F.);
#16569=ORIENTED_EDGE('',*,*,#12700,.T.);
#16570=ORIENTED_EDGE('',*,*,#12699,.F.);
#16571=ORIENTED_EDGE('',*,*,#12700,.F.);
#16572=ORIENTED_EDGE('',*,*,#12701,.T.);
#16573=ORIENTED_EDGE('',*,*,#12702,.F.);
#16574=ORIENTED_EDGE('',*,*,#12701,.F.);
#16575=ORIENTED_EDGE('',*,*,#12703,.F.);
#16576=ORIENTED_EDGE('',*,*,#12704,.T.);
#16577=ORIENTED_EDGE('',*,*,#12705,.T.);
#16578=ORIENTED_EDGE('',*,*,#12704,.F.);
#16579=ORIENTED_EDGE('',*,*,#12705,.F.);
#16580=ORIENTED_EDGE('',*,*,#12706,.T.);
#16581=ORIENTED_EDGE('',*,*,#12707,.T.);
#16582=ORIENTED_EDGE('',*,*,#12706,.F.);
#16583=ORIENTED_EDGE('',*,*,#12707,.F.);
#16584=ORIENTED_EDGE('',*,*,#12708,.T.);
#16585=ORIENTED_EDGE('',*,*,#12709,.T.);
#16586=ORIENTED_EDGE('',*,*,#12708,.F.);
#16587=ORIENTED_EDGE('',*,*,#12710,.T.);
#16588=ORIENTED_EDGE('',*,*,#12709,.F.);
#16589=ORIENTED_EDGE('',*,*,#12710,.F.);
#16590=ORIENTED_EDGE('',*,*,#12711,.T.);
#16591=ORIENTED_EDGE('',*,*,#12712,.F.);
#16592=ORIENTED_EDGE('',*,*,#12711,.F.);
#16593=ORIENTED_EDGE('',*,*,#12713,.F.);
#16594=ORIENTED_EDGE('',*,*,#12714,.T.);
#16595=ORIENTED_EDGE('',*,*,#12715,.T.);
#16596=ORIENTED_EDGE('',*,*,#12714,.F.);
#16597=ORIENTED_EDGE('',*,*,#12715,.F.);
#16598=ORIENTED_EDGE('',*,*,#12716,.T.);
#16599=ORIENTED_EDGE('',*,*,#12717,.T.);
#16600=ORIENTED_EDGE('',*,*,#12716,.F.);
#16601=ORIENTED_EDGE('',*,*,#12717,.F.);
#16602=ORIENTED_EDGE('',*,*,#12718,.T.);
#16603=ORIENTED_EDGE('',*,*,#12719,.T.);
#16604=ORIENTED_EDGE('',*,*,#12718,.F.);
#16605=ORIENTED_EDGE('',*,*,#12720,.T.);
#16606=ORIENTED_EDGE('',*,*,#12719,.F.);
#16607=ORIENTED_EDGE('',*,*,#12720,.F.);
#16608=ORIENTED_EDGE('',*,*,#12721,.T.);
#16609=ORIENTED_EDGE('',*,*,#12722,.F.);
#16610=ORIENTED_EDGE('',*,*,#12721,.F.);
#16611=ORIENTED_EDGE('',*,*,#12723,.F.);
#16612=ORIENTED_EDGE('',*,*,#12724,.T.);
#16613=ORIENTED_EDGE('',*,*,#12725,.T.);
#16614=ORIENTED_EDGE('',*,*,#12724,.F.);
#16615=ORIENTED_EDGE('',*,*,#12725,.F.);
#16616=ORIENTED_EDGE('',*,*,#12726,.T.);
#16617=ORIENTED_EDGE('',*,*,#12727,.T.);
#16618=ORIENTED_EDGE('',*,*,#12726,.F.);
#16619=ORIENTED_EDGE('',*,*,#12727,.F.);
#16620=ORIENTED_EDGE('',*,*,#12728,.T.);
#16621=ORIENTED_EDGE('',*,*,#12729,.T.);
#16622=ORIENTED_EDGE('',*,*,#12728,.F.);
#16623=ORIENTED_EDGE('',*,*,#12730,.T.);
#16624=ORIENTED_EDGE('',*,*,#12729,.F.);
#16625=ORIENTED_EDGE('',*,*,#12730,.F.);
#16626=ORIENTED_EDGE('',*,*,#12731,.T.);
#16627=ORIENTED_EDGE('',*,*,#12732,.F.);
#16628=ORIENTED_EDGE('',*,*,#12731,.F.);
#16629=ORIENTED_EDGE('',*,*,#12733,.F.);
#16630=ORIENTED_EDGE('',*,*,#12734,.T.);
#16631=ORIENTED_EDGE('',*,*,#12735,.T.);
#16632=ORIENTED_EDGE('',*,*,#12734,.F.);
#16633=ORIENTED_EDGE('',*,*,#12735,.F.);
#16634=ORIENTED_EDGE('',*,*,#12736,.T.);
#16635=ORIENTED_EDGE('',*,*,#12737,.T.);
#16636=ORIENTED_EDGE('',*,*,#12736,.F.);
#16637=ORIENTED_EDGE('',*,*,#12737,.F.);
#16638=ORIENTED_EDGE('',*,*,#12738,.T.);
#16639=ORIENTED_EDGE('',*,*,#12739,.T.);
#16640=ORIENTED_EDGE('',*,*,#12738,.F.);
#16641=ORIENTED_EDGE('',*,*,#12740,.T.);
#16642=ORIENTED_EDGE('',*,*,#12739,.F.);
#16643=ORIENTED_EDGE('',*,*,#12740,.F.);
#16644=ORIENTED_EDGE('',*,*,#12741,.T.);
#16645=ORIENTED_EDGE('',*,*,#12742,.F.);
#16646=ORIENTED_EDGE('',*,*,#12741,.F.);
#16647=ORIENTED_EDGE('',*,*,#12743,.F.);
#16648=ORIENTED_EDGE('',*,*,#12744,.T.);
#16649=ORIENTED_EDGE('',*,*,#12745,.T.);
#16650=ORIENTED_EDGE('',*,*,#12744,.F.);
#16651=ORIENTED_EDGE('',*,*,#12745,.F.);
#16652=ORIENTED_EDGE('',*,*,#12746,.T.);
#16653=ORIENTED_EDGE('',*,*,#12747,.T.);
#16654=ORIENTED_EDGE('',*,*,#12746,.F.);
#16655=ORIENTED_EDGE('',*,*,#12747,.F.);
#16656=ORIENTED_EDGE('',*,*,#12748,.T.);
#16657=ORIENTED_EDGE('',*,*,#12749,.T.);
#16658=ORIENTED_EDGE('',*,*,#12748,.F.);
#16659=ORIENTED_EDGE('',*,*,#12750,.T.);
#16660=ORIENTED_EDGE('',*,*,#12749,.F.);
#16661=ORIENTED_EDGE('',*,*,#12750,.F.);
#16662=ORIENTED_EDGE('',*,*,#12751,.T.);
#16663=ORIENTED_EDGE('',*,*,#12752,.F.);
#16664=ORIENTED_EDGE('',*,*,#12751,.F.);
#16665=ORIENTED_EDGE('',*,*,#12753,.F.);
#16666=ORIENTED_EDGE('',*,*,#12754,.T.);
#16667=ORIENTED_EDGE('',*,*,#12755,.T.);
#16668=ORIENTED_EDGE('',*,*,#12754,.F.);
#16669=ORIENTED_EDGE('',*,*,#12755,.F.);
#16670=ORIENTED_EDGE('',*,*,#12756,.T.);
#16671=ORIENTED_EDGE('',*,*,#12757,.T.);
#16672=ORIENTED_EDGE('',*,*,#12756,.F.);
#16673=ORIENTED_EDGE('',*,*,#12757,.F.);
#16674=ORIENTED_EDGE('',*,*,#12758,.T.);
#16675=ORIENTED_EDGE('',*,*,#12759,.T.);
#16676=ORIENTED_EDGE('',*,*,#12758,.F.);
#16677=ORIENTED_EDGE('',*,*,#12760,.T.);
#16678=ORIENTED_EDGE('',*,*,#12759,.F.);
#16679=ORIENTED_EDGE('',*,*,#12760,.F.);
#16680=ORIENTED_EDGE('',*,*,#12761,.T.);
#16681=ORIENTED_EDGE('',*,*,#12762,.F.);
#16682=ORIENTED_EDGE('',*,*,#12761,.F.);
#16683=ORIENTED_EDGE('',*,*,#12763,.F.);
#16684=ORIENTED_EDGE('',*,*,#12764,.T.);
#16685=ORIENTED_EDGE('',*,*,#12765,.T.);
#16686=ORIENTED_EDGE('',*,*,#12764,.F.);
#16687=ORIENTED_EDGE('',*,*,#12765,.F.);
#16688=ORIENTED_EDGE('',*,*,#12766,.T.);
#16689=ORIENTED_EDGE('',*,*,#12767,.T.);
#16690=ORIENTED_EDGE('',*,*,#12766,.F.);
#16691=ORIENTED_EDGE('',*,*,#12767,.F.);
#16692=ORIENTED_EDGE('',*,*,#12768,.T.);
#16693=ORIENTED_EDGE('',*,*,#12769,.T.);
#16694=ORIENTED_EDGE('',*,*,#12768,.F.);
#16695=ORIENTED_EDGE('',*,*,#12770,.T.);
#16696=ORIENTED_EDGE('',*,*,#12769,.F.);
#16697=ORIENTED_EDGE('',*,*,#12770,.F.);
#16698=ORIENTED_EDGE('',*,*,#12771,.T.);
#16699=ORIENTED_EDGE('',*,*,#12772,.F.);
#16700=ORIENTED_EDGE('',*,*,#12771,.F.);
#16701=ORIENTED_EDGE('',*,*,#12773,.T.);
#16702=ORIENTED_EDGE('',*,*,#12774,.T.);
#16703=ORIENTED_EDGE('',*,*,#12775,.T.);
#16704=ORIENTED_EDGE('',*,*,#12776,.T.);
#16705=ORIENTED_EDGE('',*,*,#12774,.F.);
#16706=ORIENTED_EDGE('',*,*,#12777,.F.);
#16707=ORIENTED_EDGE('',*,*,#12778,.F.);
#16708=ORIENTED_EDGE('',*,*,#12779,.T.);
#16709=ORIENTED_EDGE('',*,*,#12775,.F.);
#16710=ORIENTED_EDGE('',*,*,#12776,.F.);
#16711=ORIENTED_EDGE('',*,*,#12779,.F.);
#16712=ORIENTED_EDGE('',*,*,#12780,.F.);
#16713=ORIENTED_EDGE('',*,*,#12640,.T.);
#16714=ORIENTED_EDGE('',*,*,#12646,.T.);
#16715=ORIENTED_EDGE('',*,*,#12652,.T.);
#16716=ORIENTED_EDGE('',*,*,#12773,.F.);
#16717=ORIENTED_EDGE('',*,*,#12777,.T.);
#16718=ORIENTED_EDGE('',*,*,#12778,.T.);
#16719=ORIENTED_EDGE('',*,*,#12781,.T.);
#16720=ORIENTED_EDGE('',*,*,#12782,.T.);
#16721=ORIENTED_EDGE('',*,*,#12781,.F.);
#16722=ORIENTED_EDGE('',*,*,#12783,.T.);
#16723=ORIENTED_EDGE('',*,*,#12782,.F.);
#16724=ORIENTED_EDGE('',*,*,#12784,.T.);
#16725=ORIENTED_EDGE('',*,*,#12785,.T.);
#16726=ORIENTED_EDGE('',*,*,#12786,.T.);
#16727=ORIENTED_EDGE('',*,*,#12787,.T.);
#16728=ORIENTED_EDGE('',*,*,#12786,.F.);
#16729=ORIENTED_EDGE('',*,*,#12788,.F.);
#16730=ORIENTED_EDGE('',*,*,#12789,.F.);
#16731=ORIENTED_EDGE('',*,*,#12790,.T.);
#16732=ORIENTED_EDGE('',*,*,#12784,.F.);
#16733=ORIENTED_EDGE('',*,*,#12785,.F.);
#16734=ORIENTED_EDGE('',*,*,#12790,.F.);
#16735=ORIENTED_EDGE('',*,*,#12787,.F.);
#16736=ORIENTED_EDGE('',*,*,#12663,.T.);
#16737=ORIENTED_EDGE('',*,*,#12683,.T.);
#16738=ORIENTED_EDGE('',*,*,#12703,.T.);
#16739=ORIENTED_EDGE('',*,*,#12713,.T.);
#16740=ORIENTED_EDGE('',*,*,#12723,.T.);
#16741=ORIENTED_EDGE('',*,*,#12733,.T.);
#16742=ORIENTED_EDGE('',*,*,#12743,.T.);
#16743=ORIENTED_EDGE('',*,*,#12753,.T.);
#16744=ORIENTED_EDGE('',*,*,#12763,.T.);
#16745=ORIENTED_EDGE('',*,*,#12791,.T.);
#16746=ORIENTED_EDGE('',*,*,#12693,.T.);
#16747=ORIENTED_EDGE('',*,*,#12673,.T.);
#16748=ORIENTED_EDGE('',*,*,#12653,.T.);
#16749=ORIENTED_EDGE('',*,*,#12792,.T.);
#16750=ORIENTED_EDGE('',*,*,#12793,.T.);
#16751=ORIENTED_EDGE('',*,*,#12788,.T.);
#16752=ORIENTED_EDGE('',*,*,#12789,.T.);
#16753=ORIENTED_EDGE('',*,*,#12793,.F.);
#16754=ORIENTED_EDGE('',*,*,#12792,.F.);
#16755=ORIENTED_EDGE('',*,*,#12634,.T.);
#16756=ORIENTED_EDGE('',*,*,#12672,.T.);
#16757=ORIENTED_EDGE('',*,*,#12692,.T.);
#16758=ORIENTED_EDGE('',*,*,#12712,.T.);
#16759=ORIENTED_EDGE('',*,*,#12732,.T.);
#16760=ORIENTED_EDGE('',*,*,#12752,.T.);
#16761=ORIENTED_EDGE('',*,*,#12772,.T.);
#16762=ORIENTED_EDGE('',*,*,#12794,.T.);
#16763=ORIENTED_EDGE('',*,*,#12795,.F.);
#16764=ORIENTED_EDGE('',*,*,#12796,.T.);
#16765=ORIENTED_EDGE('',*,*,#12797,.F.);
#16766=ORIENTED_EDGE('',*,*,#12798,.T.);
#16767=ORIENTED_EDGE('',*,*,#12799,.F.);
#16768=ORIENTED_EDGE('',*,*,#12800,.T.);
#16769=ORIENTED_EDGE('',*,*,#12801,.F.);
#16770=ORIENTED_EDGE('',*,*,#12802,.T.);
#16771=ORIENTED_EDGE('',*,*,#12803,.T.);
#16772=ORIENTED_EDGE('',*,*,#12804,.T.);
#16773=ORIENTED_EDGE('',*,*,#12805,.F.);
#16774=ORIENTED_EDGE('',*,*,#12806,.T.);
#16775=ORIENTED_EDGE('',*,*,#12807,.T.);
#16776=ORIENTED_EDGE('',*,*,#12808,.F.);
#16777=ORIENTED_EDGE('',*,*,#12809,.F.);
#16778=ORIENTED_EDGE('',*,*,#12810,.T.);
#16779=ORIENTED_EDGE('',*,*,#12811,.T.);
#16780=ORIENTED_EDGE('',*,*,#12812,.F.);
#16781=ORIENTED_EDGE('',*,*,#12813,.T.);
#16782=ORIENTED_EDGE('',*,*,#12814,.T.);
#16783=ORIENTED_EDGE('',*,*,#12815,.F.);
#16784=ORIENTED_EDGE('',*,*,#12816,.T.);
#16785=ORIENTED_EDGE('',*,*,#12817,.F.);
#16786=ORIENTED_EDGE('',*,*,#12818,.T.);
#16787=ORIENTED_EDGE('',*,*,#12819,.F.);
#16788=ORIENTED_EDGE('',*,*,#12820,.T.);
#16789=ORIENTED_EDGE('',*,*,#12821,.F.);
#16790=ORIENTED_EDGE('',*,*,#12822,.T.);
#16791=ORIENTED_EDGE('',*,*,#12823,.T.);
#16792=ORIENTED_EDGE('',*,*,#12824,.T.);
#16793=ORIENTED_EDGE('',*,*,#12825,.F.);
#16794=ORIENTED_EDGE('',*,*,#12826,.T.);
#16795=ORIENTED_EDGE('',*,*,#12827,.T.);
#16796=ORIENTED_EDGE('',*,*,#12828,.F.);
#16797=ORIENTED_EDGE('',*,*,#12829,.F.);
#16798=ORIENTED_EDGE('',*,*,#12830,.T.);
#16799=ORIENTED_EDGE('',*,*,#12831,.T.);
#16800=ORIENTED_EDGE('',*,*,#12832,.F.);
#16801=ORIENTED_EDGE('',*,*,#12833,.T.);
#16802=ORIENTED_EDGE('',*,*,#12834,.T.);
#16803=ORIENTED_EDGE('',*,*,#12835,.F.);
#16804=ORIENTED_EDGE('',*,*,#12836,.T.);
#16805=ORIENTED_EDGE('',*,*,#12837,.F.);
#16806=ORIENTED_EDGE('',*,*,#12838,.T.);
#16807=ORIENTED_EDGE('',*,*,#12839,.F.);
#16808=ORIENTED_EDGE('',*,*,#12840,.T.);
#16809=ORIENTED_EDGE('',*,*,#12841,.F.);
#16810=ORIENTED_EDGE('',*,*,#12842,.T.);
#16811=ORIENTED_EDGE('',*,*,#12843,.T.);
#16812=ORIENTED_EDGE('',*,*,#12844,.T.);
#16813=ORIENTED_EDGE('',*,*,#12845,.F.);
#16814=ORIENTED_EDGE('',*,*,#12846,.T.);
#16815=ORIENTED_EDGE('',*,*,#12847,.T.);
#16816=ORIENTED_EDGE('',*,*,#12848,.F.);
#16817=ORIENTED_EDGE('',*,*,#12849,.F.);
#16818=ORIENTED_EDGE('',*,*,#12850,.T.);
#16819=ORIENTED_EDGE('',*,*,#12851,.T.);
#16820=ORIENTED_EDGE('',*,*,#12852,.F.);
#16821=ORIENTED_EDGE('',*,*,#12853,.T.);
#16822=ORIENTED_EDGE('',*,*,#12854,.T.);
#16823=ORIENTED_EDGE('',*,*,#12855,.F.);
#16824=ORIENTED_EDGE('',*,*,#12856,.T.);
#16825=ORIENTED_EDGE('',*,*,#12857,.F.);
#16826=ORIENTED_EDGE('',*,*,#12858,.T.);
#16827=ORIENTED_EDGE('',*,*,#12859,.F.);
#16828=ORIENTED_EDGE('',*,*,#12860,.T.);
#16829=ORIENTED_EDGE('',*,*,#12861,.F.);
#16830=ORIENTED_EDGE('',*,*,#12862,.T.);
#16831=ORIENTED_EDGE('',*,*,#12863,.F.);
#16832=ORIENTED_EDGE('',*,*,#12864,.T.);
#16833=ORIENTED_EDGE('',*,*,#12865,.F.);
#16834=ORIENTED_EDGE('',*,*,#12866,.T.);
#16835=ORIENTED_EDGE('',*,*,#12867,.F.);
#16836=ORIENTED_EDGE('',*,*,#12868,.T.);
#16837=ORIENTED_EDGE('',*,*,#12869,.F.);
#16838=ORIENTED_EDGE('',*,*,#12870,.T.);
#16839=ORIENTED_EDGE('',*,*,#12871,.F.);
#16840=ORIENTED_EDGE('',*,*,#12872,.T.);
#16841=ORIENTED_EDGE('',*,*,#12873,.F.);
#16842=ORIENTED_EDGE('',*,*,#12874,.T.);
#16843=ORIENTED_EDGE('',*,*,#12875,.F.);
#16844=ORIENTED_EDGE('',*,*,#12876,.T.);
#16845=ORIENTED_EDGE('',*,*,#12877,.F.);
#16846=ORIENTED_EDGE('',*,*,#12878,.T.);
#16847=ORIENTED_EDGE('',*,*,#12879,.F.);
#16848=ORIENTED_EDGE('',*,*,#12880,.T.);
#16849=ORIENTED_EDGE('',*,*,#12881,.F.);
#16850=ORIENTED_EDGE('',*,*,#12882,.T.);
#16851=ORIENTED_EDGE('',*,*,#12883,.F.);
#16852=ORIENTED_EDGE('',*,*,#12884,.T.);
#16853=ORIENTED_EDGE('',*,*,#12885,.F.);
#16854=ORIENTED_EDGE('',*,*,#12886,.T.);
#16855=ORIENTED_EDGE('',*,*,#12887,.F.);
#16856=ORIENTED_EDGE('',*,*,#12888,.T.);
#16857=ORIENTED_EDGE('',*,*,#12889,.F.);
#16858=ORIENTED_EDGE('',*,*,#12890,.T.);
#16859=ORIENTED_EDGE('',*,*,#12891,.F.);
#16860=ORIENTED_EDGE('',*,*,#12892,.T.);
#16861=ORIENTED_EDGE('',*,*,#12893,.F.);
#16862=ORIENTED_EDGE('',*,*,#12894,.T.);
#16863=ORIENTED_EDGE('',*,*,#12895,.F.);
#16864=ORIENTED_EDGE('',*,*,#12896,.T.);
#16865=ORIENTED_EDGE('',*,*,#12897,.F.);
#16866=ORIENTED_EDGE('',*,*,#12898,.T.);
#16867=ORIENTED_EDGE('',*,*,#12899,.F.);
#16868=ORIENTED_EDGE('',*,*,#12900,.T.);
#16869=ORIENTED_EDGE('',*,*,#12901,.F.);
#16870=ORIENTED_EDGE('',*,*,#12902,.T.);
#16871=ORIENTED_EDGE('',*,*,#12903,.F.);
#16872=ORIENTED_EDGE('',*,*,#12904,.T.);
#16873=ORIENTED_EDGE('',*,*,#12905,.F.);
#16874=ORIENTED_EDGE('',*,*,#12906,.T.);
#16875=ORIENTED_EDGE('',*,*,#12907,.F.);
#16876=ORIENTED_EDGE('',*,*,#12908,.T.);
#16877=ORIENTED_EDGE('',*,*,#12909,.F.);
#16878=ORIENTED_EDGE('',*,*,#12910,.T.);
#16879=ORIENTED_EDGE('',*,*,#12911,.F.);
#16880=ORIENTED_EDGE('',*,*,#12912,.T.);
#16881=ORIENTED_EDGE('',*,*,#12913,.F.);
#16882=ORIENTED_EDGE('',*,*,#12914,.T.);
#16883=ORIENTED_EDGE('',*,*,#12915,.F.);
#16884=ORIENTED_EDGE('',*,*,#12916,.T.);
#16885=ORIENTED_EDGE('',*,*,#12917,.F.);
#16886=ORIENTED_EDGE('',*,*,#12918,.T.);
#16887=ORIENTED_EDGE('',*,*,#12919,.F.);
#16888=ORIENTED_EDGE('',*,*,#12920,.T.);
#16889=ORIENTED_EDGE('',*,*,#12921,.F.);
#16890=ORIENTED_EDGE('',*,*,#12922,.T.);
#16891=ORIENTED_EDGE('',*,*,#12923,.F.);
#16892=ORIENTED_EDGE('',*,*,#12924,.T.);
#16893=ORIENTED_EDGE('',*,*,#12925,.F.);
#16894=ORIENTED_EDGE('',*,*,#12926,.T.);
#16895=ORIENTED_EDGE('',*,*,#12927,.F.);
#16896=ORIENTED_EDGE('',*,*,#12928,.T.);
#16897=ORIENTED_EDGE('',*,*,#12929,.F.);
#16898=ORIENTED_EDGE('',*,*,#12930,.T.);
#16899=ORIENTED_EDGE('',*,*,#12931,.F.);
#16900=ORIENTED_EDGE('',*,*,#12932,.T.);
#16901=ORIENTED_EDGE('',*,*,#12933,.F.);
#16902=ORIENTED_EDGE('',*,*,#12934,.T.);
#16903=ORIENTED_EDGE('',*,*,#12935,.F.);
#16904=ORIENTED_EDGE('',*,*,#12936,.T.);
#16905=ORIENTED_EDGE('',*,*,#12937,.F.);
#16906=ORIENTED_EDGE('',*,*,#12938,.T.);
#16907=ORIENTED_EDGE('',*,*,#12939,.F.);
#16908=ORIENTED_EDGE('',*,*,#12940,.T.);
#16909=ORIENTED_EDGE('',*,*,#12941,.F.);
#16910=ORIENTED_EDGE('',*,*,#12942,.T.);
#16911=ORIENTED_EDGE('',*,*,#12943,.F.);
#16912=ORIENTED_EDGE('',*,*,#12944,.T.);
#16913=ORIENTED_EDGE('',*,*,#12945,.F.);
#16914=ORIENTED_EDGE('',*,*,#12946,.T.);
#16915=ORIENTED_EDGE('',*,*,#12947,.F.);
#16916=ORIENTED_EDGE('',*,*,#12948,.T.);
#16917=ORIENTED_EDGE('',*,*,#12949,.F.);
#16918=ORIENTED_EDGE('',*,*,#12950,.T.);
#16919=ORIENTED_EDGE('',*,*,#12951,.F.);
#16920=ORIENTED_EDGE('',*,*,#12952,.T.);
#16921=ORIENTED_EDGE('',*,*,#12953,.F.);
#16922=ORIENTED_EDGE('',*,*,#12954,.T.);
#16923=ORIENTED_EDGE('',*,*,#12955,.F.);
#16924=ORIENTED_EDGE('',*,*,#12956,.T.);
#16925=ORIENTED_EDGE('',*,*,#12957,.F.);
#16926=ORIENTED_EDGE('',*,*,#12958,.T.);
#16927=ORIENTED_EDGE('',*,*,#12959,.F.);
#16928=ORIENTED_EDGE('',*,*,#12960,.T.);
#16929=ORIENTED_EDGE('',*,*,#12961,.F.);
#16930=ORIENTED_EDGE('',*,*,#12962,.F.);
#16931=ORIENTED_EDGE('',*,*,#12762,.T.);
#16932=ORIENTED_EDGE('',*,*,#12742,.T.);
#16933=ORIENTED_EDGE('',*,*,#12722,.T.);
#16934=ORIENTED_EDGE('',*,*,#12702,.T.);
#16935=ORIENTED_EDGE('',*,*,#12682,.T.);
#16936=ORIENTED_EDGE('',*,*,#12662,.T.);
#16937=ORIENTED_EDGE('',*,*,#12628,.T.);
#16938=ORIENTED_EDGE('',*,*,#12847,.F.);
#16939=ORIENTED_EDGE('',*,*,#12963,.T.);
#16940=ORIENTED_EDGE('',*,*,#12964,.F.);
#16941=ORIENTED_EDGE('',*,*,#12965,.T.);
#16942=ORIENTED_EDGE('',*,*,#12966,.F.);
#16943=ORIENTED_EDGE('',*,*,#12967,.T.);
#16944=ORIENTED_EDGE('',*,*,#12852,.T.);
#16945=ORIENTED_EDGE('',*,*,#12968,.T.);
#16946=ORIENTED_EDGE('',*,*,#12967,.F.);
#16947=ORIENTED_EDGE('',*,*,#12969,.T.);
#16948=ORIENTED_EDGE('',*,*,#12970,.T.);
#16949=ORIENTED_EDGE('',*,*,#12853,.F.);
#16950=ORIENTED_EDGE('',*,*,#12971,.F.);
#16951=ORIENTED_EDGE('',*,*,#12972,.T.);
#16952=ORIENTED_EDGE('',*,*,#12850,.F.);
#16953=ORIENTED_EDGE('',*,*,#12973,.T.);
#16954=ORIENTED_EDGE('',*,*,#12966,.T.);
#16955=ORIENTED_EDGE('',*,*,#12974,.F.);
#16956=ORIENTED_EDGE('',*,*,#12971,.T.);
#16957=ORIENTED_EDGE('',*,*,#12975,.T.);
#16958=ORIENTED_EDGE('',*,*,#12969,.F.);
#16959=ORIENTED_EDGE('',*,*,#12976,.F.);
#16960=ORIENTED_EDGE('',*,*,#12977,.T.);
#16961=ORIENTED_EDGE('',*,*,#12959,.T.);
#16962=ORIENTED_EDGE('',*,*,#12978,.T.);
#16963=ORIENTED_EDGE('',*,*,#12977,.F.);
#16964=ORIENTED_EDGE('',*,*,#12979,.T.);
#16965=ORIENTED_EDGE('',*,*,#12980,.F.);
#16966=ORIENTED_EDGE('',*,*,#12960,.F.);
#16967=ORIENTED_EDGE('',*,*,#12981,.F.);
#16968=ORIENTED_EDGE('',*,*,#12982,.T.);
#16969=ORIENTED_EDGE('',*,*,#12957,.T.);
#16970=ORIENTED_EDGE('',*,*,#12983,.T.);
#16971=ORIENTED_EDGE('',*,*,#12976,.T.);
#16972=ORIENTED_EDGE('',*,*,#12984,.F.);
#16973=ORIENTED_EDGE('',*,*,#12981,.T.);
#16974=ORIENTED_EDGE('',*,*,#12985,.F.);
#16975=ORIENTED_EDGE('',*,*,#12986,.T.);
#16976=ORIENTED_EDGE('',*,*,#12979,.F.);
#16977=ORIENTED_EDGE('',*,*,#12983,.F.);
#16978=ORIENTED_EDGE('',*,*,#12956,.F.);
#16979=ORIENTED_EDGE('',*,*,#12987,.F.);
#16980=ORIENTED_EDGE('',*,*,#12985,.T.);
#16981=ORIENTED_EDGE('',*,*,#12986,.F.);
#16982=ORIENTED_EDGE('',*,*,#12987,.T.);
#16983=ORIENTED_EDGE('',*,*,#12961,.T.);
#16984=ORIENTED_EDGE('',*,*,#12980,.T.);
#16985=ORIENTED_EDGE('',*,*,#12988,.F.);
#16986=ORIENTED_EDGE('',*,*,#12989,.T.);
#16987=ORIENTED_EDGE('',*,*,#12953,.T.);
#16988=ORIENTED_EDGE('',*,*,#12990,.T.);
#16989=ORIENTED_EDGE('',*,*,#12989,.F.);
#16990=ORIENTED_EDGE('',*,*,#12991,.T.);
#16991=ORIENTED_EDGE('',*,*,#12992,.F.);
#16992=ORIENTED_EDGE('',*,*,#12954,.F.);
#16993=ORIENTED_EDGE('',*,*,#12993,.F.);
#16994=ORIENTED_EDGE('',*,*,#12994,.T.);
#16995=ORIENTED_EDGE('',*,*,#12951,.T.);
#16996=ORIENTED_EDGE('',*,*,#12995,.T.);
#16997=ORIENTED_EDGE('',*,*,#12988,.T.);
#16998=ORIENTED_EDGE('',*,*,#12996,.F.);
#16999=ORIENTED_EDGE('',*,*,#12993,.T.);
#17000=ORIENTED_EDGE('',*,*,#12997,.F.);
#17001=ORIENTED_EDGE('',*,*,#12998,.T.);
#17002=ORIENTED_EDGE('',*,*,#12991,.F.);
#17003=ORIENTED_EDGE('',*,*,#12995,.F.);
#17004=ORIENTED_EDGE('',*,*,#12950,.F.);
#17005=ORIENTED_EDGE('',*,*,#12999,.F.);
#17006=ORIENTED_EDGE('',*,*,#12997,.T.);
#17007=ORIENTED_EDGE('',*,*,#12998,.F.);
#17008=ORIENTED_EDGE('',*,*,#12999,.T.);
#17009=ORIENTED_EDGE('',*,*,#12955,.T.);
#17010=ORIENTED_EDGE('',*,*,#12992,.T.);
#17011=ORIENTED_EDGE('',*,*,#12827,.F.);
#17012=ORIENTED_EDGE('',*,*,#13000,.T.);
#17013=ORIENTED_EDGE('',*,*,#13001,.F.);
#17014=ORIENTED_EDGE('',*,*,#13002,.T.);
#17015=ORIENTED_EDGE('',*,*,#13003,.F.);
#17016=ORIENTED_EDGE('',*,*,#13004,.T.);
#17017=ORIENTED_EDGE('',*,*,#12947,.T.);
#17018=ORIENTED_EDGE('',*,*,#13005,.T.);
#17019=ORIENTED_EDGE('',*,*,#13004,.F.);
#17020=ORIENTED_EDGE('',*,*,#13006,.T.);
#17021=ORIENTED_EDGE('',*,*,#13007,.F.);
#17022=ORIENTED_EDGE('',*,*,#12948,.F.);
#17023=ORIENTED_EDGE('',*,*,#13008,.F.);
#17024=ORIENTED_EDGE('',*,*,#13009,.T.);
#17025=ORIENTED_EDGE('',*,*,#12945,.T.);
#17026=ORIENTED_EDGE('',*,*,#13010,.T.);
#17027=ORIENTED_EDGE('',*,*,#13003,.T.);
#17028=ORIENTED_EDGE('',*,*,#13011,.F.);
#17029=ORIENTED_EDGE('',*,*,#13008,.T.);
#17030=ORIENTED_EDGE('',*,*,#13012,.F.);
#17031=ORIENTED_EDGE('',*,*,#13013,.T.);
#17032=ORIENTED_EDGE('',*,*,#13006,.F.);
#17033=ORIENTED_EDGE('',*,*,#13010,.F.);
#17034=ORIENTED_EDGE('',*,*,#12944,.F.);
#17035=ORIENTED_EDGE('',*,*,#13014,.F.);
#17036=ORIENTED_EDGE('',*,*,#13012,.T.);
#17037=ORIENTED_EDGE('',*,*,#13013,.F.);
#17038=ORIENTED_EDGE('',*,*,#13014,.T.);
#17039=ORIENTED_EDGE('',*,*,#12949,.T.);
#17040=ORIENTED_EDGE('',*,*,#13007,.T.);
#17041=ORIENTED_EDGE('',*,*,#13015,.F.);
#17042=ORIENTED_EDGE('',*,*,#13016,.T.);
#17043=ORIENTED_EDGE('',*,*,#12941,.T.);
#17044=ORIENTED_EDGE('',*,*,#13017,.T.);
#17045=ORIENTED_EDGE('',*,*,#13016,.F.);
#17046=ORIENTED_EDGE('',*,*,#13018,.T.);
#17047=ORIENTED_EDGE('',*,*,#13019,.F.);
#17048=ORIENTED_EDGE('',*,*,#12942,.F.);
#17049=ORIENTED_EDGE('',*,*,#13020,.F.);
#17050=ORIENTED_EDGE('',*,*,#13021,.T.);
#17051=ORIENTED_EDGE('',*,*,#12939,.T.);
#17052=ORIENTED_EDGE('',*,*,#13022,.T.);
#17053=ORIENTED_EDGE('',*,*,#13015,.T.);
#17054=ORIENTED_EDGE('',*,*,#13023,.F.);
#17055=ORIENTED_EDGE('',*,*,#13020,.T.);
#17056=ORIENTED_EDGE('',*,*,#13024,.F.);
#17057=ORIENTED_EDGE('',*,*,#13025,.T.);
#17058=ORIENTED_EDGE('',*,*,#13018,.F.);
#17059=ORIENTED_EDGE('',*,*,#13022,.F.);
#17060=ORIENTED_EDGE('',*,*,#12938,.F.);
#17061=ORIENTED_EDGE('',*,*,#13026,.F.);
#17062=ORIENTED_EDGE('',*,*,#13024,.T.);
#17063=ORIENTED_EDGE('',*,*,#13025,.F.);
#17064=ORIENTED_EDGE('',*,*,#13026,.T.);
#17065=ORIENTED_EDGE('',*,*,#12943,.T.);
#17066=ORIENTED_EDGE('',*,*,#13019,.T.);
#17067=ORIENTED_EDGE('',*,*,#13027,.F.);
#17068=ORIENTED_EDGE('',*,*,#13028,.T.);
#17069=ORIENTED_EDGE('',*,*,#12815,.T.);
#17070=ORIENTED_EDGE('',*,*,#13029,.T.);
#17071=ORIENTED_EDGE('',*,*,#13028,.F.);
#17072=ORIENTED_EDGE('',*,*,#13030,.T.);
#17073=ORIENTED_EDGE('',*,*,#13031,.T.);
#17074=ORIENTED_EDGE('',*,*,#12816,.F.);
#17075=ORIENTED_EDGE('',*,*,#13032,.F.);
#17076=ORIENTED_EDGE('',*,*,#13033,.T.);
#17077=ORIENTED_EDGE('',*,*,#12832,.T.);
#17078=ORIENTED_EDGE('',*,*,#13034,.T.);
#17079=ORIENTED_EDGE('',*,*,#13032,.T.);
#17080=ORIENTED_EDGE('',*,*,#13035,.F.);
#17081=ORIENTED_EDGE('',*,*,#13036,.T.);
#17082=ORIENTED_EDGE('',*,*,#13037,.T.);
#17083=ORIENTED_EDGE('',*,*,#13038,.F.);
#17084=ORIENTED_EDGE('',*,*,#13034,.F.);
#17085=ORIENTED_EDGE('',*,*,#12831,.F.);
#17086=ORIENTED_EDGE('',*,*,#13039,.F.);
#17087=ORIENTED_EDGE('',*,*,#13035,.T.);
#17088=ORIENTED_EDGE('',*,*,#13036,.F.);
#17089=ORIENTED_EDGE('',*,*,#13039,.T.);
#17090=ORIENTED_EDGE('',*,*,#12830,.F.);
#17091=ORIENTED_EDGE('',*,*,#13040,.T.);
#17092=ORIENTED_EDGE('',*,*,#13041,.F.);
#17093=ORIENTED_EDGE('',*,*,#13042,.T.);
#17094=ORIENTED_EDGE('',*,*,#12935,.T.);
#17095=ORIENTED_EDGE('',*,*,#13043,.T.);
#17096=ORIENTED_EDGE('',*,*,#13042,.F.);
#17097=ORIENTED_EDGE('',*,*,#13044,.T.);
#17098=ORIENTED_EDGE('',*,*,#13045,.F.);
#17099=ORIENTED_EDGE('',*,*,#12936,.F.);
#17100=ORIENTED_EDGE('',*,*,#13046,.F.);
#17101=ORIENTED_EDGE('',*,*,#13047,.T.);
#17102=ORIENTED_EDGE('',*,*,#12933,.T.);
#17103=ORIENTED_EDGE('',*,*,#13048,.T.);
#17104=ORIENTED_EDGE('',*,*,#13041,.T.);
#17105=ORIENTED_EDGE('',*,*,#13049,.F.);
#17106=ORIENTED_EDGE('',*,*,#13046,.T.);
#17107=ORIENTED_EDGE('',*,*,#13050,.F.);
#17108=ORIENTED_EDGE('',*,*,#13051,.T.);
#17109=ORIENTED_EDGE('',*,*,#13044,.F.);
#17110=ORIENTED_EDGE('',*,*,#13048,.F.);
#17111=ORIENTED_EDGE('',*,*,#12932,.F.);
#17112=ORIENTED_EDGE('',*,*,#13052,.F.);
#17113=ORIENTED_EDGE('',*,*,#13050,.T.);
#17114=ORIENTED_EDGE('',*,*,#13051,.F.);
#17115=ORIENTED_EDGE('',*,*,#13052,.T.);
#17116=ORIENTED_EDGE('',*,*,#12937,.T.);
#17117=ORIENTED_EDGE('',*,*,#13045,.T.);
#17118=ORIENTED_EDGE('',*,*,#13053,.F.);
#17119=ORIENTED_EDGE('',*,*,#13054,.T.);
#17120=ORIENTED_EDGE('',*,*,#12929,.T.);
#17121=ORIENTED_EDGE('',*,*,#13055,.T.);
#17122=ORIENTED_EDGE('',*,*,#13054,.F.);
#17123=ORIENTED_EDGE('',*,*,#13056,.T.);
#17124=ORIENTED_EDGE('',*,*,#13057,.F.);
#17125=ORIENTED_EDGE('',*,*,#12930,.F.);
#17126=ORIENTED_EDGE('',*,*,#13058,.F.);
#17127=ORIENTED_EDGE('',*,*,#13059,.T.);
#17128=ORIENTED_EDGE('',*,*,#12927,.T.);
#17129=ORIENTED_EDGE('',*,*,#13060,.T.);
#17130=ORIENTED_EDGE('',*,*,#13053,.T.);
#17131=ORIENTED_EDGE('',*,*,#13061,.F.);
#17132=ORIENTED_EDGE('',*,*,#13058,.T.);
#17133=ORIENTED_EDGE('',*,*,#13062,.F.);
#17134=ORIENTED_EDGE('',*,*,#13063,.T.);
#17135=ORIENTED_EDGE('',*,*,#13056,.F.);
#17136=ORIENTED_EDGE('',*,*,#13060,.F.);
#17137=ORIENTED_EDGE('',*,*,#12926,.F.);
#17138=ORIENTED_EDGE('',*,*,#13064,.F.);
#17139=ORIENTED_EDGE('',*,*,#13062,.T.);
#17140=ORIENTED_EDGE('',*,*,#13063,.F.);
#17141=ORIENTED_EDGE('',*,*,#13064,.T.);
#17142=ORIENTED_EDGE('',*,*,#12931,.T.);
#17143=ORIENTED_EDGE('',*,*,#13057,.T.);
#17144=ORIENTED_EDGE('',*,*,#12823,.F.);
#17145=ORIENTED_EDGE('',*,*,#13065,.T.);
#17146=ORIENTED_EDGE('',*,*,#13066,.F.);
#17147=ORIENTED_EDGE('',*,*,#13067,.T.);
#17148=ORIENTED_EDGE('',*,*,#13066,.T.);
#17149=ORIENTED_EDGE('',*,*,#13068,.F.);
#17150=ORIENTED_EDGE('',*,*,#13069,.T.);
#17151=ORIENTED_EDGE('',*,*,#13070,.F.);
#17152=ORIENTED_EDGE('',*,*,#13071,.T.);
#17153=ORIENTED_EDGE('',*,*,#13065,.F.);
#17154=ORIENTED_EDGE('',*,*,#12822,.F.);
#17155=ORIENTED_EDGE('',*,*,#13072,.F.);
#17156=ORIENTED_EDGE('',*,*,#13068,.T.);
#17157=ORIENTED_EDGE('',*,*,#13069,.F.);
#17158=ORIENTED_EDGE('',*,*,#13072,.T.);
#17159=ORIENTED_EDGE('',*,*,#12821,.T.);
#17160=ORIENTED_EDGE('',*,*,#13073,.T.);
#17161=ORIENTED_EDGE('',*,*,#13073,.F.);
#17162=ORIENTED_EDGE('',*,*,#12820,.F.);
#17163=ORIENTED_EDGE('',*,*,#13074,.T.);
#17164=ORIENTED_EDGE('',*,*,#13070,.T.);
#17165=ORIENTED_EDGE('',*,*,#13075,.F.);
#17166=ORIENTED_EDGE('',*,*,#13076,.T.);
#17167=ORIENTED_EDGE('',*,*,#12923,.T.);
#17168=ORIENTED_EDGE('',*,*,#13077,.T.);
#17169=ORIENTED_EDGE('',*,*,#13076,.F.);
#17170=ORIENTED_EDGE('',*,*,#13078,.T.);
#17171=ORIENTED_EDGE('',*,*,#13079,.F.);
#17172=ORIENTED_EDGE('',*,*,#12924,.F.);
#17173=ORIENTED_EDGE('',*,*,#13080,.F.);
#17174=ORIENTED_EDGE('',*,*,#13081,.T.);
#17175=ORIENTED_EDGE('',*,*,#12921,.T.);
#17176=ORIENTED_EDGE('',*,*,#13082,.T.);
#17177=ORIENTED_EDGE('',*,*,#13075,.T.);
#17178=ORIENTED_EDGE('',*,*,#13083,.F.);
#17179=ORIENTED_EDGE('',*,*,#13080,.T.);
#17180=ORIENTED_EDGE('',*,*,#13084,.F.);
#17181=ORIENTED_EDGE('',*,*,#13085,.T.);
#17182=ORIENTED_EDGE('',*,*,#13078,.F.);
#17183=ORIENTED_EDGE('',*,*,#13082,.F.);
#17184=ORIENTED_EDGE('',*,*,#12920,.F.);
#17185=ORIENTED_EDGE('',*,*,#13086,.F.);
#17186=ORIENTED_EDGE('',*,*,#13084,.T.);
#17187=ORIENTED_EDGE('',*,*,#13085,.F.);
#17188=ORIENTED_EDGE('',*,*,#13086,.T.);
#17189=ORIENTED_EDGE('',*,*,#12925,.T.);
#17190=ORIENTED_EDGE('',*,*,#13079,.T.);
#17191=ORIENTED_EDGE('',*,*,#13087,.F.);
#17192=ORIENTED_EDGE('',*,*,#13088,.T.);
#17193=ORIENTED_EDGE('',*,*,#12917,.T.);
#17194=ORIENTED_EDGE('',*,*,#13089,.T.);
#17195=ORIENTED_EDGE('',*,*,#13088,.F.);
#17196=ORIENTED_EDGE('',*,*,#13090,.T.);
#17197=ORIENTED_EDGE('',*,*,#13091,.F.);
#17198=ORIENTED_EDGE('',*,*,#12918,.F.);
#17199=ORIENTED_EDGE('',*,*,#13092,.F.);
#17200=ORIENTED_EDGE('',*,*,#13093,.T.);
#17201=ORIENTED_EDGE('',*,*,#12915,.T.);
#17202=ORIENTED_EDGE('',*,*,#13094,.T.);
#17203=ORIENTED_EDGE('',*,*,#13087,.T.);
#17204=ORIENTED_EDGE('',*,*,#13095,.F.);
#17205=ORIENTED_EDGE('',*,*,#13092,.T.);
#17206=ORIENTED_EDGE('',*,*,#13096,.F.);
#17207=ORIENTED_EDGE('',*,*,#13097,.T.);
#17208=ORIENTED_EDGE('',*,*,#13090,.F.);
#17209=ORIENTED_EDGE('',*,*,#13094,.F.);
#17210=ORIENTED_EDGE('',*,*,#12914,.F.);
#17211=ORIENTED_EDGE('',*,*,#13098,.F.);
#17212=ORIENTED_EDGE('',*,*,#13096,.T.);
#17213=ORIENTED_EDGE('',*,*,#13097,.F.);
#17214=ORIENTED_EDGE('',*,*,#13098,.T.);
#17215=ORIENTED_EDGE('',*,*,#12919,.T.);
#17216=ORIENTED_EDGE('',*,*,#13091,.T.);
#17217=ORIENTED_EDGE('',*,*,#13099,.F.);
#17218=ORIENTED_EDGE('',*,*,#13100,.T.);
#17219=ORIENTED_EDGE('',*,*,#12795,.T.);
#17220=ORIENTED_EDGE('',*,*,#13101,.T.);
#17221=ORIENTED_EDGE('',*,*,#13100,.F.);
#17222=ORIENTED_EDGE('',*,*,#13102,.T.);
#17223=ORIENTED_EDGE('',*,*,#13103,.T.);
#17224=ORIENTED_EDGE('',*,*,#12796,.F.);
#17225=ORIENTED_EDGE('',*,*,#13104,.F.);
#17226=ORIENTED_EDGE('',*,*,#13105,.T.);
#17227=ORIENTED_EDGE('',*,*,#12812,.T.);
#17228=ORIENTED_EDGE('',*,*,#13106,.T.);
#17229=ORIENTED_EDGE('',*,*,#13104,.T.);
#17230=ORIENTED_EDGE('',*,*,#13107,.F.);
#17231=ORIENTED_EDGE('',*,*,#13108,.T.);
#17232=ORIENTED_EDGE('',*,*,#13109,.T.);
#17233=ORIENTED_EDGE('',*,*,#13110,.F.);
#17234=ORIENTED_EDGE('',*,*,#13106,.F.);
#17235=ORIENTED_EDGE('',*,*,#12811,.F.);
#17236=ORIENTED_EDGE('',*,*,#13111,.F.);
#17237=ORIENTED_EDGE('',*,*,#13107,.T.);
#17238=ORIENTED_EDGE('',*,*,#13108,.F.);
#17239=ORIENTED_EDGE('',*,*,#13111,.T.);
#17240=ORIENTED_EDGE('',*,*,#12810,.F.);
#17241=ORIENTED_EDGE('',*,*,#13112,.T.);
#17242=ORIENTED_EDGE('',*,*,#13113,.F.);
#17243=ORIENTED_EDGE('',*,*,#13114,.T.);
#17244=ORIENTED_EDGE('',*,*,#12911,.T.);
#17245=ORIENTED_EDGE('',*,*,#13115,.T.);
#17246=ORIENTED_EDGE('',*,*,#13114,.F.);
#17247=ORIENTED_EDGE('',*,*,#13116,.T.);
#17248=ORIENTED_EDGE('',*,*,#13117,.F.);
#17249=ORIENTED_EDGE('',*,*,#12912,.F.);
#17250=ORIENTED_EDGE('',*,*,#13118,.F.);
#17251=ORIENTED_EDGE('',*,*,#13119,.T.);
#17252=ORIENTED_EDGE('',*,*,#12909,.T.);
#17253=ORIENTED_EDGE('',*,*,#13120,.T.);
#17254=ORIENTED_EDGE('',*,*,#13113,.T.);
#17255=ORIENTED_EDGE('',*,*,#13121,.F.);
#17256=ORIENTED_EDGE('',*,*,#13118,.T.);
#17257=ORIENTED_EDGE('',*,*,#13122,.F.);
#17258=ORIENTED_EDGE('',*,*,#13123,.T.);
#17259=ORIENTED_EDGE('',*,*,#13116,.F.);
#17260=ORIENTED_EDGE('',*,*,#13120,.F.);
#17261=ORIENTED_EDGE('',*,*,#12908,.F.);
#17262=ORIENTED_EDGE('',*,*,#13124,.F.);
#17263=ORIENTED_EDGE('',*,*,#13122,.T.);
#17264=ORIENTED_EDGE('',*,*,#13123,.F.);
#17265=ORIENTED_EDGE('',*,*,#13124,.T.);
#17266=ORIENTED_EDGE('',*,*,#12913,.T.);
#17267=ORIENTED_EDGE('',*,*,#13117,.T.);
#17268=ORIENTED_EDGE('',*,*,#13125,.F.);
#17269=ORIENTED_EDGE('',*,*,#13126,.T.);
#17270=ORIENTED_EDGE('',*,*,#12905,.T.);
#17271=ORIENTED_EDGE('',*,*,#13127,.T.);
#17272=ORIENTED_EDGE('',*,*,#13126,.F.);
#17273=ORIENTED_EDGE('',*,*,#13128,.T.);
#17274=ORIENTED_EDGE('',*,*,#13129,.F.);
#17275=ORIENTED_EDGE('',*,*,#12906,.F.);
#17276=ORIENTED_EDGE('',*,*,#13130,.F.);
#17277=ORIENTED_EDGE('',*,*,#13131,.T.);
#17278=ORIENTED_EDGE('',*,*,#12903,.T.);
#17279=ORIENTED_EDGE('',*,*,#13132,.T.);
#17280=ORIENTED_EDGE('',*,*,#13125,.T.);
#17281=ORIENTED_EDGE('',*,*,#13133,.F.);
#17282=ORIENTED_EDGE('',*,*,#13130,.T.);
#17283=ORIENTED_EDGE('',*,*,#13134,.F.);
#17284=ORIENTED_EDGE('',*,*,#13135,.T.);
#17285=ORIENTED_EDGE('',*,*,#13128,.F.);
#17286=ORIENTED_EDGE('',*,*,#13132,.F.);
#17287=ORIENTED_EDGE('',*,*,#12902,.F.);
#17288=ORIENTED_EDGE('',*,*,#13136,.F.);
#17289=ORIENTED_EDGE('',*,*,#13134,.T.);
#17290=ORIENTED_EDGE('',*,*,#13135,.F.);
#17291=ORIENTED_EDGE('',*,*,#13136,.T.);
#17292=ORIENTED_EDGE('',*,*,#12907,.T.);
#17293=ORIENTED_EDGE('',*,*,#13129,.T.);
#17294=ORIENTED_EDGE('',*,*,#13137,.F.);
#17295=ORIENTED_EDGE('',*,*,#13138,.T.);
#17296=ORIENTED_EDGE('',*,*,#12899,.T.);
#17297=ORIENTED_EDGE('',*,*,#13139,.T.);
#17298=ORIENTED_EDGE('',*,*,#13138,.F.);
#17299=ORIENTED_EDGE('',*,*,#13140,.T.);
#17300=ORIENTED_EDGE('',*,*,#13141,.F.);
#17301=ORIENTED_EDGE('',*,*,#12900,.F.);
#17302=ORIENTED_EDGE('',*,*,#13142,.F.);
#17303=ORIENTED_EDGE('',*,*,#13143,.T.);
#17304=ORIENTED_EDGE('',*,*,#12897,.T.);
#17305=ORIENTED_EDGE('',*,*,#13144,.T.);
#17306=ORIENTED_EDGE('',*,*,#13137,.T.);
#17307=ORIENTED_EDGE('',*,*,#13145,.F.);
#17308=ORIENTED_EDGE('',*,*,#13142,.T.);
#17309=ORIENTED_EDGE('',*,*,#13146,.F.);
#17310=ORIENTED_EDGE('',*,*,#13147,.T.);
#17311=ORIENTED_EDGE('',*,*,#13140,.F.);
#17312=ORIENTED_EDGE('',*,*,#13144,.F.);
#17313=ORIENTED_EDGE('',*,*,#12896,.F.);
#17314=ORIENTED_EDGE('',*,*,#13148,.F.);
#17315=ORIENTED_EDGE('',*,*,#13146,.T.);
#17316=ORIENTED_EDGE('',*,*,#13147,.F.);
#17317=ORIENTED_EDGE('',*,*,#13148,.T.);
#17318=ORIENTED_EDGE('',*,*,#12901,.T.);
#17319=ORIENTED_EDGE('',*,*,#13141,.T.);
#17320=ORIENTED_EDGE('',*,*,#12807,.F.);
#17321=ORIENTED_EDGE('',*,*,#13149,.T.);
#17322=ORIENTED_EDGE('',*,*,#13150,.F.);
#17323=ORIENTED_EDGE('',*,*,#13151,.T.);
#17324=ORIENTED_EDGE('',*,*,#13152,.F.);
#17325=ORIENTED_EDGE('',*,*,#13153,.T.);
#17326=ORIENTED_EDGE('',*,*,#12893,.T.);
#17327=ORIENTED_EDGE('',*,*,#13154,.T.);
#17328=ORIENTED_EDGE('',*,*,#13153,.F.);
#17329=ORIENTED_EDGE('',*,*,#13155,.T.);
#17330=ORIENTED_EDGE('',*,*,#13156,.F.);
#17331=ORIENTED_EDGE('',*,*,#12894,.F.);
#17332=ORIENTED_EDGE('',*,*,#13157,.F.);
#17333=ORIENTED_EDGE('',*,*,#13158,.T.);
#17334=ORIENTED_EDGE('',*,*,#12891,.T.);
#17335=ORIENTED_EDGE('',*,*,#13159,.T.);
#17336=ORIENTED_EDGE('',*,*,#13152,.T.);
#17337=ORIENTED_EDGE('',*,*,#13160,.F.);
#17338=ORIENTED_EDGE('',*,*,#13157,.T.);
#17339=ORIENTED_EDGE('',*,*,#13161,.F.);
#17340=ORIENTED_EDGE('',*,*,#13162,.T.);
#17341=ORIENTED_EDGE('',*,*,#13155,.F.);
#17342=ORIENTED_EDGE('',*,*,#13159,.F.);
#17343=ORIENTED_EDGE('',*,*,#12890,.F.);
#17344=ORIENTED_EDGE('',*,*,#13163,.F.);
#17345=ORIENTED_EDGE('',*,*,#13161,.T.);
#17346=ORIENTED_EDGE('',*,*,#13162,.F.);
#17347=ORIENTED_EDGE('',*,*,#13163,.T.);
#17348=ORIENTED_EDGE('',*,*,#12895,.T.);
#17349=ORIENTED_EDGE('',*,*,#13156,.T.);
#17350=ORIENTED_EDGE('',*,*,#13164,.F.);
#17351=ORIENTED_EDGE('',*,*,#13165,.T.);
#17352=ORIENTED_EDGE('',*,*,#12887,.T.);
#17353=ORIENTED_EDGE('',*,*,#13166,.T.);
#17354=ORIENTED_EDGE('',*,*,#13165,.F.);
#17355=ORIENTED_EDGE('',*,*,#13167,.T.);
#17356=ORIENTED_EDGE('',*,*,#13168,.F.);
#17357=ORIENTED_EDGE('',*,*,#12888,.F.);
#17358=ORIENTED_EDGE('',*,*,#13169,.F.);
#17359=ORIENTED_EDGE('',*,*,#13170,.T.);
#17360=ORIENTED_EDGE('',*,*,#12885,.T.);
#17361=ORIENTED_EDGE('',*,*,#13171,.T.);
#17362=ORIENTED_EDGE('',*,*,#13164,.T.);
#17363=ORIENTED_EDGE('',*,*,#13172,.F.);
#17364=ORIENTED_EDGE('',*,*,#13169,.T.);
#17365=ORIENTED_EDGE('',*,*,#13173,.F.);
#17366=ORIENTED_EDGE('',*,*,#13174,.T.);
#17367=ORIENTED_EDGE('',*,*,#13167,.F.);
#17368=ORIENTED_EDGE('',*,*,#13171,.F.);
#17369=ORIENTED_EDGE('',*,*,#12884,.F.);
#17370=ORIENTED_EDGE('',*,*,#13175,.F.);
#17371=ORIENTED_EDGE('',*,*,#13173,.T.);
#17372=ORIENTED_EDGE('',*,*,#13174,.F.);
#17373=ORIENTED_EDGE('',*,*,#13175,.T.);
#17374=ORIENTED_EDGE('',*,*,#12889,.T.);
#17375=ORIENTED_EDGE('',*,*,#13168,.T.);
#17376=ORIENTED_EDGE('',*,*,#12803,.F.);
#17377=ORIENTED_EDGE('',*,*,#13176,.T.);
#17378=ORIENTED_EDGE('',*,*,#13177,.F.);
#17379=ORIENTED_EDGE('',*,*,#13178,.T.);
#17380=ORIENTED_EDGE('',*,*,#13177,.T.);
#17381=ORIENTED_EDGE('',*,*,#13179,.F.);
#17382=ORIENTED_EDGE('',*,*,#13180,.T.);
#17383=ORIENTED_EDGE('',*,*,#13181,.F.);
#17384=ORIENTED_EDGE('',*,*,#13182,.T.);
#17385=ORIENTED_EDGE('',*,*,#13176,.F.);
#17386=ORIENTED_EDGE('',*,*,#12802,.F.);
#17387=ORIENTED_EDGE('',*,*,#13183,.F.);
#17388=ORIENTED_EDGE('',*,*,#13179,.T.);
#17389=ORIENTED_EDGE('',*,*,#13180,.F.);
#17390=ORIENTED_EDGE('',*,*,#13183,.T.);
#17391=ORIENTED_EDGE('',*,*,#12801,.T.);
#17392=ORIENTED_EDGE('',*,*,#13184,.T.);
#17393=ORIENTED_EDGE('',*,*,#13184,.F.);
#17394=ORIENTED_EDGE('',*,*,#12800,.F.);
#17395=ORIENTED_EDGE('',*,*,#13185,.T.);
#17396=ORIENTED_EDGE('',*,*,#13181,.T.);
#17397=ORIENTED_EDGE('',*,*,#13186,.F.);
#17398=ORIENTED_EDGE('',*,*,#13187,.T.);
#17399=ORIENTED_EDGE('',*,*,#12881,.T.);
#17400=ORIENTED_EDGE('',*,*,#13188,.T.);
#17401=ORIENTED_EDGE('',*,*,#13187,.F.);
#17402=ORIENTED_EDGE('',*,*,#13189,.T.);
#17403=ORIENTED_EDGE('',*,*,#13190,.F.);
#17404=ORIENTED_EDGE('',*,*,#12882,.F.);
#17405=ORIENTED_EDGE('',*,*,#13191,.F.);
#17406=ORIENTED_EDGE('',*,*,#13192,.T.);
#17407=ORIENTED_EDGE('',*,*,#12879,.T.);
#17408=ORIENTED_EDGE('',*,*,#13193,.T.);
#17409=ORIENTED_EDGE('',*,*,#13186,.T.);
#17410=ORIENTED_EDGE('',*,*,#13194,.F.);
#17411=ORIENTED_EDGE('',*,*,#13191,.T.);
#17412=ORIENTED_EDGE('',*,*,#13195,.F.);
#17413=ORIENTED_EDGE('',*,*,#13196,.T.);
#17414=ORIENTED_EDGE('',*,*,#13189,.F.);
#17415=ORIENTED_EDGE('',*,*,#13193,.F.);
#17416=ORIENTED_EDGE('',*,*,#12878,.F.);
#17417=ORIENTED_EDGE('',*,*,#13197,.F.);
#17418=ORIENTED_EDGE('',*,*,#13195,.T.);
#17419=ORIENTED_EDGE('',*,*,#13196,.F.);
#17420=ORIENTED_EDGE('',*,*,#13197,.T.);
#17421=ORIENTED_EDGE('',*,*,#12883,.T.);
#17422=ORIENTED_EDGE('',*,*,#13190,.T.);
#17423=ORIENTED_EDGE('',*,*,#13198,.F.);
#17424=ORIENTED_EDGE('',*,*,#13199,.T.);
#17425=ORIENTED_EDGE('',*,*,#12875,.T.);
#17426=ORIENTED_EDGE('',*,*,#13200,.T.);
#17427=ORIENTED_EDGE('',*,*,#13199,.F.);
#17428=ORIENTED_EDGE('',*,*,#13201,.T.);
#17429=ORIENTED_EDGE('',*,*,#13202,.F.);
#17430=ORIENTED_EDGE('',*,*,#12876,.F.);
#17431=ORIENTED_EDGE('',*,*,#13203,.F.);
#17432=ORIENTED_EDGE('',*,*,#13204,.T.);
#17433=ORIENTED_EDGE('',*,*,#12873,.T.);
#17434=ORIENTED_EDGE('',*,*,#13205,.T.);
#17435=ORIENTED_EDGE('',*,*,#13198,.T.);
#17436=ORIENTED_EDGE('',*,*,#13206,.F.);
#17437=ORIENTED_EDGE('',*,*,#13203,.T.);
#17438=ORIENTED_EDGE('',*,*,#13207,.F.);
#17439=ORIENTED_EDGE('',*,*,#13208,.T.);
#17440=ORIENTED_EDGE('',*,*,#13201,.F.);
#17441=ORIENTED_EDGE('',*,*,#13205,.F.);
#17442=ORIENTED_EDGE('',*,*,#12872,.F.);
#17443=ORIENTED_EDGE('',*,*,#13209,.F.);
#17444=ORIENTED_EDGE('',*,*,#13207,.T.);
#17445=ORIENTED_EDGE('',*,*,#13208,.F.);
#17446=ORIENTED_EDGE('',*,*,#13209,.T.);
#17447=ORIENTED_EDGE('',*,*,#12877,.T.);
#17448=ORIENTED_EDGE('',*,*,#13202,.T.);
#17449=ORIENTED_EDGE('',*,*,#12843,.F.);
#17450=ORIENTED_EDGE('',*,*,#13210,.T.);
#17451=ORIENTED_EDGE('',*,*,#13211,.F.);
#17452=ORIENTED_EDGE('',*,*,#13212,.T.);
#17453=ORIENTED_EDGE('',*,*,#13213,.F.);
#17454=ORIENTED_EDGE('',*,*,#13214,.T.);
#17455=ORIENTED_EDGE('',*,*,#12841,.T.);
#17456=ORIENTED_EDGE('',*,*,#13215,.T.);
#17457=ORIENTED_EDGE('',*,*,#13211,.T.);
#17458=ORIENTED_EDGE('',*,*,#13216,.F.);
#17459=ORIENTED_EDGE('',*,*,#13213,.T.);
#17460=ORIENTED_EDGE('',*,*,#13217,.F.);
#17461=ORIENTED_EDGE('',*,*,#13218,.T.);
#17462=ORIENTED_EDGE('',*,*,#13215,.F.);
#17463=ORIENTED_EDGE('',*,*,#12840,.F.);
#17464=ORIENTED_EDGE('',*,*,#13219,.T.);
#17465=ORIENTED_EDGE('',*,*,#13217,.T.);
#17466=ORIENTED_EDGE('',*,*,#13220,.F.);
#17467=ORIENTED_EDGE('',*,*,#13221,.T.);
#17468=ORIENTED_EDGE('',*,*,#12869,.T.);
#17469=ORIENTED_EDGE('',*,*,#13222,.T.);
#17470=ORIENTED_EDGE('',*,*,#13221,.F.);
#17471=ORIENTED_EDGE('',*,*,#13223,.T.);
#17472=ORIENTED_EDGE('',*,*,#13224,.F.);
#17473=ORIENTED_EDGE('',*,*,#12870,.F.);
#17474=ORIENTED_EDGE('',*,*,#13225,.F.);
#17475=ORIENTED_EDGE('',*,*,#13226,.T.);
#17476=ORIENTED_EDGE('',*,*,#12867,.T.);
#17477=ORIENTED_EDGE('',*,*,#13227,.T.);
#17478=ORIENTED_EDGE('',*,*,#13220,.T.);
#17479=ORIENTED_EDGE('',*,*,#13228,.F.);
#17480=ORIENTED_EDGE('',*,*,#13225,.T.);
#17481=ORIENTED_EDGE('',*,*,#13229,.F.);
#17482=ORIENTED_EDGE('',*,*,#13230,.T.);
#17483=ORIENTED_EDGE('',*,*,#13223,.F.);
#17484=ORIENTED_EDGE('',*,*,#13227,.F.);
#17485=ORIENTED_EDGE('',*,*,#12866,.F.);
#17486=ORIENTED_EDGE('',*,*,#13231,.F.);
#17487=ORIENTED_EDGE('',*,*,#13229,.T.);
#17488=ORIENTED_EDGE('',*,*,#13230,.F.);
#17489=ORIENTED_EDGE('',*,*,#13231,.T.);
#17490=ORIENTED_EDGE('',*,*,#12871,.T.);
#17491=ORIENTED_EDGE('',*,*,#13224,.T.);
#17492=ORIENTED_EDGE('',*,*,#13232,.F.);
#17493=ORIENTED_EDGE('',*,*,#13233,.T.);
#17494=ORIENTED_EDGE('',*,*,#12863,.T.);
#17495=ORIENTED_EDGE('',*,*,#13234,.T.);
#17496=ORIENTED_EDGE('',*,*,#13233,.F.);
#17497=ORIENTED_EDGE('',*,*,#13235,.T.);
#17498=ORIENTED_EDGE('',*,*,#13236,.F.);
#17499=ORIENTED_EDGE('',*,*,#12864,.F.);
#17500=ORIENTED_EDGE('',*,*,#13237,.F.);
#17501=ORIENTED_EDGE('',*,*,#13238,.T.);
#17502=ORIENTED_EDGE('',*,*,#12861,.T.);
#17503=ORIENTED_EDGE('',*,*,#13239,.T.);
#17504=ORIENTED_EDGE('',*,*,#13232,.T.);
#17505=ORIENTED_EDGE('',*,*,#13240,.F.);
#17506=ORIENTED_EDGE('',*,*,#13237,.T.);
#17507=ORIENTED_EDGE('',*,*,#13241,.F.);
#17508=ORIENTED_EDGE('',*,*,#13242,.T.);
#17509=ORIENTED_EDGE('',*,*,#13235,.F.);
#17510=ORIENTED_EDGE('',*,*,#13239,.F.);
#17511=ORIENTED_EDGE('',*,*,#12860,.F.);
#17512=ORIENTED_EDGE('',*,*,#13243,.F.);
#17513=ORIENTED_EDGE('',*,*,#13241,.T.);
#17514=ORIENTED_EDGE('',*,*,#13242,.F.);
#17515=ORIENTED_EDGE('',*,*,#13243,.T.);
#17516=ORIENTED_EDGE('',*,*,#12865,.T.);
#17517=ORIENTED_EDGE('',*,*,#13236,.T.);
#17518=ORIENTED_EDGE('',*,*,#13244,.F.);
#17519=ORIENTED_EDGE('',*,*,#13245,.T.);
#17520=ORIENTED_EDGE('',*,*,#12857,.T.);
#17521=ORIENTED_EDGE('',*,*,#13246,.T.);
#17522=ORIENTED_EDGE('',*,*,#13245,.F.);
#17523=ORIENTED_EDGE('',*,*,#13247,.T.);
#17524=ORIENTED_EDGE('',*,*,#13248,.F.);
#17525=ORIENTED_EDGE('',*,*,#12858,.F.);
#17526=ORIENTED_EDGE('',*,*,#13249,.F.);
#17527=ORIENTED_EDGE('',*,*,#13250,.T.);
#17528=ORIENTED_EDGE('',*,*,#12855,.T.);
#17529=ORIENTED_EDGE('',*,*,#13251,.T.);
#17530=ORIENTED_EDGE('',*,*,#13244,.T.);
#17531=ORIENTED_EDGE('',*,*,#13252,.F.);
#17532=ORIENTED_EDGE('',*,*,#13249,.T.);
#17533=ORIENTED_EDGE('',*,*,#13253,.F.);
#17534=ORIENTED_EDGE('',*,*,#13254,.T.);
#17535=ORIENTED_EDGE('',*,*,#13247,.F.);
#17536=ORIENTED_EDGE('',*,*,#13251,.F.);
#17537=ORIENTED_EDGE('',*,*,#12854,.F.);
#17538=ORIENTED_EDGE('',*,*,#13255,.F.);
#17539=ORIENTED_EDGE('',*,*,#13253,.T.);
#17540=ORIENTED_EDGE('',*,*,#13254,.F.);
#17541=ORIENTED_EDGE('',*,*,#13255,.T.);
#17542=ORIENTED_EDGE('',*,*,#12859,.T.);
#17543=ORIENTED_EDGE('',*,*,#13248,.T.);
#17544=ORIENTED_EDGE('',*,*,#13256,.F.);
#17545=ORIENTED_EDGE('',*,*,#13257,.T.);
#17546=ORIENTED_EDGE('',*,*,#12845,.T.);
#17547=ORIENTED_EDGE('',*,*,#13258,.T.);
#17548=ORIENTED_EDGE('',*,*,#12964,.T.);
#17549=ORIENTED_EDGE('',*,*,#13259,.F.);
#17550=ORIENTED_EDGE('',*,*,#13256,.T.);
#17551=ORIENTED_EDGE('',*,*,#13260,.F.);
#17552=ORIENTED_EDGE('',*,*,#13261,.T.);
#17553=ORIENTED_EDGE('',*,*,#13258,.F.);
#17554=ORIENTED_EDGE('',*,*,#12844,.F.);
#17555=ORIENTED_EDGE('',*,*,#13262,.T.);
#17556=ORIENTED_EDGE('',*,*,#13260,.T.);
#17557=ORIENTED_EDGE('',*,*,#13263,.F.);
#17558=ORIENTED_EDGE('',*,*,#13264,.T.);
#17559=ORIENTED_EDGE('',*,*,#12835,.T.);
#17560=ORIENTED_EDGE('',*,*,#13265,.T.);
#17561=ORIENTED_EDGE('',*,*,#13264,.F.);
#17562=ORIENTED_EDGE('',*,*,#13266,.T.);
#17563=ORIENTED_EDGE('',*,*,#13267,.T.);
#17564=ORIENTED_EDGE('',*,*,#12836,.F.);
#17565=ORIENTED_EDGE('',*,*,#13268,.F.);
#17566=ORIENTED_EDGE('',*,*,#13269,.T.);
#17567=ORIENTED_EDGE('',*,*,#12838,.F.);
#17568=ORIENTED_EDGE('',*,*,#13270,.T.);
#17569=ORIENTED_EDGE('',*,*,#13263,.T.);
#17570=ORIENTED_EDGE('',*,*,#13271,.F.);
#17571=ORIENTED_EDGE('',*,*,#13268,.T.);
#17572=ORIENTED_EDGE('',*,*,#13272,.T.);
#17573=ORIENTED_EDGE('',*,*,#13266,.F.);
#17574=ORIENTED_EDGE('',*,*,#13273,.F.);
#17575=ORIENTED_EDGE('',*,*,#13274,.T.);
#17576=ORIENTED_EDGE('',*,*,#12825,.T.);
#17577=ORIENTED_EDGE('',*,*,#13275,.T.);
#17578=ORIENTED_EDGE('',*,*,#13001,.T.);
#17579=ORIENTED_EDGE('',*,*,#13276,.F.);
#17580=ORIENTED_EDGE('',*,*,#13273,.T.);
#17581=ORIENTED_EDGE('',*,*,#13277,.F.);
#17582=ORIENTED_EDGE('',*,*,#13278,.T.);
#17583=ORIENTED_EDGE('',*,*,#13275,.F.);
#17584=ORIENTED_EDGE('',*,*,#12824,.F.);
#17585=ORIENTED_EDGE('',*,*,#13279,.T.);
#17586=ORIENTED_EDGE('',*,*,#13277,.T.);
#17587=ORIENTED_EDGE('',*,*,#13280,.F.);
#17588=ORIENTED_EDGE('',*,*,#13281,.T.);
#17589=ORIENTED_EDGE('',*,*,#12818,.F.);
#17590=ORIENTED_EDGE('',*,*,#13282,.T.);
#17591=ORIENTED_EDGE('',*,*,#13027,.T.);
#17592=ORIENTED_EDGE('',*,*,#13283,.F.);
#17593=ORIENTED_EDGE('',*,*,#13280,.T.);
#17594=ORIENTED_EDGE('',*,*,#13284,.T.);
#17595=ORIENTED_EDGE('',*,*,#13030,.F.);
#17596=ORIENTED_EDGE('',*,*,#13285,.F.);
#17597=ORIENTED_EDGE('',*,*,#13286,.T.);
#17598=ORIENTED_EDGE('',*,*,#12805,.T.);
#17599=ORIENTED_EDGE('',*,*,#13287,.T.);
#17600=ORIENTED_EDGE('',*,*,#13150,.T.);
#17601=ORIENTED_EDGE('',*,*,#13288,.F.);
#17602=ORIENTED_EDGE('',*,*,#13285,.T.);
#17603=ORIENTED_EDGE('',*,*,#13289,.F.);
#17604=ORIENTED_EDGE('',*,*,#13290,.T.);
#17605=ORIENTED_EDGE('',*,*,#13287,.F.);
#17606=ORIENTED_EDGE('',*,*,#12804,.F.);
#17607=ORIENTED_EDGE('',*,*,#13291,.T.);
#17608=ORIENTED_EDGE('',*,*,#13289,.T.);
#17609=ORIENTED_EDGE('',*,*,#13292,.F.);
#17610=ORIENTED_EDGE('',*,*,#13293,.T.);
#17611=ORIENTED_EDGE('',*,*,#12798,.F.);
#17612=ORIENTED_EDGE('',*,*,#13294,.T.);
#17613=ORIENTED_EDGE('',*,*,#13099,.T.);
#17614=ORIENTED_EDGE('',*,*,#13295,.F.);
#17615=ORIENTED_EDGE('',*,*,#13292,.T.);
#17616=ORIENTED_EDGE('',*,*,#13296,.T.);
#17617=ORIENTED_EDGE('',*,*,#13102,.F.);
#17618=ORIENTED_EDGE('',*,*,#13262,.F.);
#17619=ORIENTED_EDGE('',*,*,#12848,.T.);
#17620=ORIENTED_EDGE('',*,*,#12965,.F.);
#17621=ORIENTED_EDGE('',*,*,#13261,.F.);
#17622=ORIENTED_EDGE('',*,*,#12970,.F.);
#17623=ORIENTED_EDGE('',*,*,#12975,.F.);
#17624=ORIENTED_EDGE('',*,*,#12973,.F.);
#17625=ORIENTED_EDGE('',*,*,#12849,.T.);
#17626=ORIENTED_EDGE('',*,*,#13270,.F.);
#17627=ORIENTED_EDGE('',*,*,#12837,.T.);
#17628=ORIENTED_EDGE('',*,*,#13267,.F.);
#17629=ORIENTED_EDGE('',*,*,#13272,.F.);
#17630=ORIENTED_EDGE('',*,*,#13212,.F.);
#17631=ORIENTED_EDGE('',*,*,#13218,.F.);
#17632=ORIENTED_EDGE('',*,*,#13219,.F.);
#17633=ORIENTED_EDGE('',*,*,#12839,.T.);
#17634=ORIENTED_EDGE('',*,*,#13279,.F.);
#17635=ORIENTED_EDGE('',*,*,#12828,.T.);
#17636=ORIENTED_EDGE('',*,*,#13002,.F.);
#17637=ORIENTED_EDGE('',*,*,#13278,.F.);
#17638=ORIENTED_EDGE('',*,*,#13297,.F.);
#17639=ORIENTED_EDGE('',*,*,#13037,.F.);
#17640=ORIENTED_EDGE('',*,*,#13040,.F.);
#17641=ORIENTED_EDGE('',*,*,#12829,.T.);
#17642=ORIENTED_EDGE('',*,*,#13282,.F.);
#17643=ORIENTED_EDGE('',*,*,#12817,.T.);
#17644=ORIENTED_EDGE('',*,*,#13031,.F.);
#17645=ORIENTED_EDGE('',*,*,#13284,.F.);
#17646=ORIENTED_EDGE('',*,*,#13067,.F.);
#17647=ORIENTED_EDGE('',*,*,#13071,.F.);
#17648=ORIENTED_EDGE('',*,*,#13074,.F.);
#17649=ORIENTED_EDGE('',*,*,#12819,.T.);
#17650=ORIENTED_EDGE('',*,*,#13291,.F.);
#17651=ORIENTED_EDGE('',*,*,#12808,.T.);
#17652=ORIENTED_EDGE('',*,*,#13151,.F.);
#17653=ORIENTED_EDGE('',*,*,#13290,.F.);
#17654=ORIENTED_EDGE('',*,*,#13298,.F.);
#17655=ORIENTED_EDGE('',*,*,#13109,.F.);
#17656=ORIENTED_EDGE('',*,*,#13112,.F.);
#17657=ORIENTED_EDGE('',*,*,#12809,.T.);
#17658=ORIENTED_EDGE('',*,*,#13294,.F.);
#17659=ORIENTED_EDGE('',*,*,#12797,.T.);
#17660=ORIENTED_EDGE('',*,*,#13103,.F.);
#17661=ORIENTED_EDGE('',*,*,#13296,.F.);
#17662=ORIENTED_EDGE('',*,*,#13178,.F.);
#17663=ORIENTED_EDGE('',*,*,#13182,.F.);
#17664=ORIENTED_EDGE('',*,*,#13185,.F.);
#17665=ORIENTED_EDGE('',*,*,#12799,.T.);
#17666=ORIENTED_EDGE('',*,*,#13265,.F.);
#17667=ORIENTED_EDGE('',*,*,#12834,.F.);
#17668=ORIENTED_EDGE('',*,*,#13269,.F.);
#17669=ORIENTED_EDGE('',*,*,#13271,.T.);
#17670=ORIENTED_EDGE('',*,*,#13246,.F.);
#17671=ORIENTED_EDGE('',*,*,#12856,.F.);
#17672=ORIENTED_EDGE('',*,*,#13250,.F.);
#17673=ORIENTED_EDGE('',*,*,#13252,.T.);
#17674=ORIENTED_EDGE('',*,*,#13234,.F.);
#17675=ORIENTED_EDGE('',*,*,#12862,.F.);
#17676=ORIENTED_EDGE('',*,*,#13238,.F.);
#17677=ORIENTED_EDGE('',*,*,#13240,.T.);
#17678=ORIENTED_EDGE('',*,*,#13222,.F.);
#17679=ORIENTED_EDGE('',*,*,#12868,.F.);
#17680=ORIENTED_EDGE('',*,*,#13226,.F.);
#17681=ORIENTED_EDGE('',*,*,#13228,.T.);
#17682=ORIENTED_EDGE('',*,*,#13210,.F.);
#17683=ORIENTED_EDGE('',*,*,#12842,.F.);
#17684=ORIENTED_EDGE('',*,*,#13214,.F.);
#17685=ORIENTED_EDGE('',*,*,#13216,.T.);
#17686=ORIENTED_EDGE('',*,*,#13200,.F.);
#17687=ORIENTED_EDGE('',*,*,#12874,.F.);
#17688=ORIENTED_EDGE('',*,*,#13204,.F.);
#17689=ORIENTED_EDGE('',*,*,#13206,.T.);
#17690=ORIENTED_EDGE('',*,*,#13188,.F.);
#17691=ORIENTED_EDGE('',*,*,#12880,.F.);
#17692=ORIENTED_EDGE('',*,*,#13192,.F.);
#17693=ORIENTED_EDGE('',*,*,#13194,.T.);
#17694=ORIENTED_EDGE('',*,*,#13166,.F.);
#17695=ORIENTED_EDGE('',*,*,#12886,.F.);
#17696=ORIENTED_EDGE('',*,*,#13170,.F.);
#17697=ORIENTED_EDGE('',*,*,#13172,.T.);
#17698=ORIENTED_EDGE('',*,*,#13154,.F.);
#17699=ORIENTED_EDGE('',*,*,#12892,.F.);
#17700=ORIENTED_EDGE('',*,*,#13158,.F.);
#17701=ORIENTED_EDGE('',*,*,#13160,.T.);
#17702=ORIENTED_EDGE('',*,*,#13149,.F.);
#17703=ORIENTED_EDGE('',*,*,#12806,.F.);
#17704=ORIENTED_EDGE('',*,*,#13286,.F.);
#17705=ORIENTED_EDGE('',*,*,#13288,.T.);
#17706=ORIENTED_EDGE('',*,*,#13139,.F.);
#17707=ORIENTED_EDGE('',*,*,#12898,.F.);
#17708=ORIENTED_EDGE('',*,*,#13143,.F.);
#17709=ORIENTED_EDGE('',*,*,#13145,.T.);
#17710=ORIENTED_EDGE('',*,*,#13127,.F.);
#17711=ORIENTED_EDGE('',*,*,#12904,.F.);
#17712=ORIENTED_EDGE('',*,*,#13131,.F.);
#17713=ORIENTED_EDGE('',*,*,#13133,.T.);
#17714=ORIENTED_EDGE('',*,*,#13115,.F.);
#17715=ORIENTED_EDGE('',*,*,#12910,.F.);
#17716=ORIENTED_EDGE('',*,*,#13119,.F.);
#17717=ORIENTED_EDGE('',*,*,#13121,.T.);
#17718=ORIENTED_EDGE('',*,*,#13105,.F.);
#17719=ORIENTED_EDGE('',*,*,#13110,.T.);
#17720=ORIENTED_EDGE('',*,*,#13298,.T.);
#17721=ORIENTED_EDGE('',*,*,#12813,.F.);
#17722=ORIENTED_EDGE('',*,*,#13101,.F.);
#17723=ORIENTED_EDGE('',*,*,#12794,.F.);
#17724=ORIENTED_EDGE('',*,*,#13293,.F.);
#17725=ORIENTED_EDGE('',*,*,#13295,.T.);
#17726=ORIENTED_EDGE('',*,*,#13089,.F.);
#17727=ORIENTED_EDGE('',*,*,#12916,.F.);
#17728=ORIENTED_EDGE('',*,*,#13093,.F.);
#17729=ORIENTED_EDGE('',*,*,#13095,.T.);
#17730=ORIENTED_EDGE('',*,*,#13077,.F.);
#17731=ORIENTED_EDGE('',*,*,#12922,.F.);
#17732=ORIENTED_EDGE('',*,*,#13081,.F.);
#17733=ORIENTED_EDGE('',*,*,#13083,.T.);
#17734=ORIENTED_EDGE('',*,*,#13055,.F.);
#17735=ORIENTED_EDGE('',*,*,#12928,.F.);
#17736=ORIENTED_EDGE('',*,*,#13059,.F.);
#17737=ORIENTED_EDGE('',*,*,#13061,.T.);
#17738=ORIENTED_EDGE('',*,*,#13043,.F.);
#17739=ORIENTED_EDGE('',*,*,#12934,.F.);
#17740=ORIENTED_EDGE('',*,*,#13047,.F.);
#17741=ORIENTED_EDGE('',*,*,#13049,.T.);
#17742=ORIENTED_EDGE('',*,*,#13033,.F.);
#17743=ORIENTED_EDGE('',*,*,#13038,.T.);
#17744=ORIENTED_EDGE('',*,*,#13297,.T.);
#17745=ORIENTED_EDGE('',*,*,#12833,.F.);
#17746=ORIENTED_EDGE('',*,*,#13029,.F.);
#17747=ORIENTED_EDGE('',*,*,#12814,.F.);
#17748=ORIENTED_EDGE('',*,*,#13281,.F.);
#17749=ORIENTED_EDGE('',*,*,#13283,.T.);
#17750=ORIENTED_EDGE('',*,*,#13017,.F.);
#17751=ORIENTED_EDGE('',*,*,#12940,.F.);
#17752=ORIENTED_EDGE('',*,*,#13021,.F.);
#17753=ORIENTED_EDGE('',*,*,#13023,.T.);
#17754=ORIENTED_EDGE('',*,*,#13005,.F.);
#17755=ORIENTED_EDGE('',*,*,#12946,.F.);
#17756=ORIENTED_EDGE('',*,*,#13009,.F.);
#17757=ORIENTED_EDGE('',*,*,#13011,.T.);
#17758=ORIENTED_EDGE('',*,*,#13000,.F.);
#17759=ORIENTED_EDGE('',*,*,#12826,.F.);
#17760=ORIENTED_EDGE('',*,*,#13274,.F.);
#17761=ORIENTED_EDGE('',*,*,#13276,.T.);
#17762=ORIENTED_EDGE('',*,*,#12990,.F.);
#17763=ORIENTED_EDGE('',*,*,#12952,.F.);
#17764=ORIENTED_EDGE('',*,*,#12994,.F.);
#17765=ORIENTED_EDGE('',*,*,#12996,.T.);
#17766=ORIENTED_EDGE('',*,*,#12978,.F.);
#17767=ORIENTED_EDGE('',*,*,#12958,.F.);
#17768=ORIENTED_EDGE('',*,*,#12982,.F.);
#17769=ORIENTED_EDGE('',*,*,#12984,.T.);
#17770=ORIENTED_EDGE('',*,*,#12968,.F.);
#17771=ORIENTED_EDGE('',*,*,#12851,.F.);
#17772=ORIENTED_EDGE('',*,*,#12972,.F.);
#17773=ORIENTED_EDGE('',*,*,#12974,.T.);
#17774=ORIENTED_EDGE('',*,*,#12963,.F.);
#17775=ORIENTED_EDGE('',*,*,#12846,.F.);
#17776=ORIENTED_EDGE('',*,*,#13257,.F.);
#17777=ORIENTED_EDGE('',*,*,#13259,.T.);
#17778=ORIENTED_EDGE('',*,*,#12780,.T.);
#17779=ORIENTED_EDGE('',*,*,#13299,.T.);
#17780=ORIENTED_EDGE('',*,*,#13300,.F.);
#17781=ORIENTED_EDGE('',*,*,#13299,.F.);
#17782=ORIENTED_EDGE('',*,*,#13301,.F.);
#17783=ORIENTED_EDGE('',*,*,#13300,.T.);
#17784=ORIENTED_EDGE('',*,*,#12791,.F.);
#17785=ORIENTED_EDGE('',*,*,#13302,.T.);
#17786=ORIENTED_EDGE('',*,*,#13301,.T.);
#17787=ORIENTED_EDGE('',*,*,#13302,.F.);
#17788=ORIENTED_EDGE('',*,*,#12962,.T.);
#17789=ORIENTED_EDGE('',*,*,#13303,.T.);
#17790=ORIENTED_EDGE('',*,*,#12783,.F.);
#17791=ORIENTED_EDGE('',*,*,#13303,.F.);
#23035=CONICAL_SURFACE('',#25059,0.0525,1.02974425867667);
#23036=CONICAL_SURFACE('',#25063,0.155,0.78539816339745);
#23037=CONICAL_SURFACE('',#25065,0.0525,1.02974425867667);
#23038=CONICAL_SURFACE('',#25069,0.155,0.78539816339745);
#23039=CONICAL_SURFACE('',#25071,0.0650000000000004,1.02974425867666);
#23040=CONICAL_SURFACE('',#25075,0.180000000000001,0.785398163397451);
#23041=CONICAL_SURFACE('',#25077,0.0649999999999999,1.02974425867666);
#23042=CONICAL_SURFACE('',#25081,0.18,0.785398163397451);
#23043=CONICAL_SURFACE('',#25083,0.065,1.02974425867666);
#23044=CONICAL_SURFACE('',#25087,0.18,0.78539816339745);
#23045=CONICAL_SURFACE('',#25089,0.1325,0.321750554396632);
#23046=CONICAL_SURFACE('',#25094,0.1325,0.785398163397466);
#23047=CONICAL_SURFACE('',#25100,0.1325,0.321750554396642);
#23048=CONICAL_SURFACE('',#25105,0.1325,0.785398163397484);
#23049=CONICAL_SURFACE('',#25111,0.1325,0.32175055439664);
#23050=CONICAL_SURFACE('',#25116,0.1325,0.785398163397479);
#23051=CONICAL_SURFACE('',#25122,0.1325,0.321750554396637);
#23052=CONICAL_SURFACE('',#25127,0.1325,0.785398163397475);
#23053=CONICAL_SURFACE('',#25133,0.1325,0.321750554396637);
#23054=CONICAL_SURFACE('',#25138,0.1325,0.785398163397475);
#23055=CONICAL_SURFACE('',#25144,0.1325,0.321750554396632);
#23056=CONICAL_SURFACE('',#25149,0.1325,0.785398163397466);
#23057=CONICAL_SURFACE('',#25155,0.1325,0.321750554396642);
#23058=CONICAL_SURFACE('',#25160,0.1325,0.785398163397484);
#23059=CONICAL_SURFACE('',#25166,0.132499999999999,0.321750554396637);
#23060=CONICAL_SURFACE('',#25171,0.132499999999999,0.785398163397475);
#23061=CONICAL_SURFACE('',#25177,0.1325,0.321750554396637);
#23062=CONICAL_SURFACE('',#25182,0.1325,0.785398163397475);
#23063=CONICAL_SURFACE('',#25188,0.1325,0.32175055439664);
#23064=CONICAL_SURFACE('',#25193,0.1325,0.785398163397479);
#23065=CONICAL_SURFACE('',#25199,0.1325,0.321750554396637);
#23066=CONICAL_SURFACE('',#25204,0.1325,0.785398163397475);
#23067=CONICAL_SURFACE('',#25210,0.1325,0.321750554396632);
#23068=CONICAL_SURFACE('',#25215,0.1325,0.785398163397466);
#23069=CONICAL_SURFACE('',#25221,0.72,0.785398163397459);
#23070=CONICAL_SURFACE('',#25230,0.72,0.785398163397459);
#23071=CONICAL_SURFACE('',#25234,4.585,0.785398163397463);
#23072=CONICAL_SURFACE('',#25243,4.585,0.785398163397463);
#23297=ADVANCED_FACE('',(#2544),#23035,.F.);
#23298=ADVANCED_FACE('',(#2545),#1992,.F.);
#23299=ADVANCED_FACE('',(#2546),#23036,.F.);
#23300=ADVANCED_FACE('',(#2547),#23037,.F.);
#23301=ADVANCED_FACE('',(#2548),#1993,.F.);
#23302=ADVANCED_FACE('',(#2549),#23038,.F.);
#23303=ADVANCED_FACE('',(#2550),#23039,.F.);
#23304=ADVANCED_FACE('',(#2551),#1994,.F.);
#23305=ADVANCED_FACE('',(#2552),#23040,.F.);
#23306=ADVANCED_FACE('',(#2553),#23041,.F.);
#23307=ADVANCED_FACE('',(#2554),#1995,.F.);
#23308=ADVANCED_FACE('',(#2555),#23042,.F.);
#23309=ADVANCED_FACE('',(#2556),#23043,.F.);
#23310=ADVANCED_FACE('',(#2557),#1996,.F.);
#23311=ADVANCED_FACE('',(#2558),#23044,.F.);
#23312=ADVANCED_FACE('',(#2559),#23045,.F.);
#23313=ADVANCED_FACE('',(#2560),#1997,.F.);
#23314=ADVANCED_FACE('',(#2561),#23046,.F.);
#23315=ADVANCED_FACE('',(#2562,#1082),#1289,.F.);
#23316=ADVANCED_FACE('',(#2563),#1998,.F.);
#23317=ADVANCED_FACE('',(#2564),#23047,.F.);
#23318=ADVANCED_FACE('',(#2565),#1999,.F.);
#23319=ADVANCED_FACE('',(#2566),#23048,.F.);
#23320=ADVANCED_FACE('',(#2567,#1083),#1290,.F.);
#23321=ADVANCED_FACE('',(#2568),#2000,.F.);
#23322=ADVANCED_FACE('',(#2569),#23049,.F.);
#23323=ADVANCED_FACE('',(#2570),#2001,.F.);
#23324=ADVANCED_FACE('',(#2571),#23050,.F.);
#23325=ADVANCED_FACE('',(#2572,#1084),#1291,.F.);
#23326=ADVANCED_FACE('',(#2573),#2002,.F.);
#23327=ADVANCED_FACE('',(#2574),#23051,.F.);
#23328=ADVANCED_FACE('',(#2575),#2003,.F.);
#23329=ADVANCED_FACE('',(#2576),#23052,.F.);
#23330=ADVANCED_FACE('',(#2577,#1085),#1292,.F.);
#23331=ADVANCED_FACE('',(#2578),#2004,.F.);
#23332=ADVANCED_FACE('',(#2579),#23053,.F.);
#23333=ADVANCED_FACE('',(#2580),#2005,.F.);
#23334=ADVANCED_FACE('',(#2581),#23054,.F.);
#23335=ADVANCED_FACE('',(#2582,#1086),#1293,.F.);
#23336=ADVANCED_FACE('',(#2583),#2006,.F.);
#23337=ADVANCED_FACE('',(#2584),#23055,.F.);
#23338=ADVANCED_FACE('',(#2585),#2007,.F.);
#23339=ADVANCED_FACE('',(#2586),#23056,.F.);
#23340=ADVANCED_FACE('',(#2587,#1087),#1294,.F.);
#23341=ADVANCED_FACE('',(#2588),#2008,.F.);
#23342=ADVANCED_FACE('',(#2589),#23057,.F.);
#23343=ADVANCED_FACE('',(#2590),#2009,.F.);
#23344=ADVANCED_FACE('',(#2591),#23058,.F.);
#23345=ADVANCED_FACE('',(#2592,#1088),#1295,.F.);
#23346=ADVANCED_FACE('',(#2593),#2010,.F.);
#23347=ADVANCED_FACE('',(#2594),#23059,.F.);
#23348=ADVANCED_FACE('',(#2595),#2011,.F.);
#23349=ADVANCED_FACE('',(#2596),#23060,.F.);
#23350=ADVANCED_FACE('',(#2597,#1089),#1296,.F.);
#23351=ADVANCED_FACE('',(#2598),#2012,.F.);
#23352=ADVANCED_FACE('',(#2599),#23061,.F.);
#23353=ADVANCED_FACE('',(#2600),#2013,.F.);
#23354=ADVANCED_FACE('',(#2601),#23062,.F.);
#23355=ADVANCED_FACE('',(#2602,#1090),#1297,.F.);
#23356=ADVANCED_FACE('',(#2603),#2014,.F.);
#23357=ADVANCED_FACE('',(#2604),#23063,.F.);
#23358=ADVANCED_FACE('',(#2605),#2015,.F.);
#23359=ADVANCED_FACE('',(#2606),#23064,.F.);
#23360=ADVANCED_FACE('',(#2607,#1091),#1298,.F.);
#23361=ADVANCED_FACE('',(#2608),#2016,.F.);
#23362=ADVANCED_FACE('',(#2609),#23065,.F.);
#23363=ADVANCED_FACE('',(#2610),#2017,.F.);
#23364=ADVANCED_FACE('',(#2611),#23066,.F.);
#23365=ADVANCED_FACE('',(#2612,#1092),#1299,.F.);
#23366=ADVANCED_FACE('',(#2613),#2018,.F.);
#23367=ADVANCED_FACE('',(#2614),#23067,.F.);
#23368=ADVANCED_FACE('',(#2615),#2019,.F.);
#23369=ADVANCED_FACE('',(#2616),#23068,.F.);
#23370=ADVANCED_FACE('',(#2617,#1093),#1300,.F.);
#23371=ADVANCED_FACE('',(#2618),#2020,.F.);
#23372=ADVANCED_FACE('',(#2619),#23069,.F.);
#23373=ADVANCED_FACE('',(#2620),#2021,.F.);
#23374=ADVANCED_FACE('',(#2621,#1094,#1095,#1096,#1097),#1301,.T.);
#23375=ADVANCED_FACE('',(#2622),#23070,.F.);
#23376=ADVANCED_FACE('',(#2623,#1098),#1302,.T.);
#23377=ADVANCED_FACE('',(#2624),#23071,.T.);
#23378=ADVANCED_FACE('',(#2625),#2022,.T.);
#23379=ADVANCED_FACE('',(#2626,#1099,#1100,#1101,#1102,#1103,#1104,#1105,
#1106,#1107,#1108,#1109,#1110,#1111),#1303,.T.);
#23380=ADVANCED_FACE('',(#2627),#23072,.T.);
#23381=ADVANCED_FACE('',(#2628,#1112,#1113,#1114,#1115,#1116,#1117,#1118,
#1119,#1120,#1121,#1122,#1123,#1124,#1125,#1126,#1127,#1128,#1129,#1130,
#1131,#1132,#1133,#1134,#1135,#1136,#1137,#1138,#1139,#1140,#1141,#1142,
#1143,#1144,#1145,#1146,#1147,#1148,#1149,#1150,#1151,#1152,#1153,#1154,
#1155,#1156),#1304,.T.);
#23382=ADVANCED_FACE('',(#2629),#2023,.F.);
#23383=ADVANCED_FACE('',(#2630),#2024,.F.);
#23384=ADVANCED_FACE('',(#2631),#1305,.F.);
#23385=ADVANCED_FACE('',(#2632),#2025,.F.);
#23386=ADVANCED_FACE('',(#2633),#1306,.F.);
#23387=ADVANCED_FACE('',(#2634),#2026,.F.);
#23388=ADVANCED_FACE('',(#2635),#1307,.F.);
#23389=ADVANCED_FACE('',(#2636),#2027,.F.);
#23390=ADVANCED_FACE('',(#2637),#1308,.F.);
#23391=ADVANCED_FACE('',(#2638),#1309,.F.);
#23392=ADVANCED_FACE('',(#2639),#2028,.F.);
#23393=ADVANCED_FACE('',(#2640),#2029,.F.);
#23394=ADVANCED_FACE('',(#2641),#1310,.F.);
#23395=ADVANCED_FACE('',(#2642),#2030,.F.);
#23396=ADVANCED_FACE('',(#2643),#1311,.F.);
#23397=ADVANCED_FACE('',(#2644),#1312,.F.);
#23398=ADVANCED_FACE('',(#2645),#2031,.F.);
#23399=ADVANCED_FACE('',(#2646),#2032,.F.);
#23400=ADVANCED_FACE('',(#2647),#2033,.F.);
#23401=ADVANCED_FACE('',(#2648),#1313,.F.);
#23402=ADVANCED_FACE('',(#2649),#2034,.F.);
#23403=ADVANCED_FACE('',(#2650),#1314,.F.);
#23404=ADVANCED_FACE('',(#2651),#1315,.F.);
#23405=ADVANCED_FACE('',(#2652),#2035,.F.);
#23406=ADVANCED_FACE('',(#2653),#2036,.F.);
#23407=ADVANCED_FACE('',(#2654),#1316,.F.);
#23408=ADVANCED_FACE('',(#2655),#2037,.F.);
#23409=ADVANCED_FACE('',(#2656),#1317,.F.);
#23410=ADVANCED_FACE('',(#2657),#1318,.F.);
#23411=ADVANCED_FACE('',(#2658),#2038,.F.);
#23412=ADVANCED_FACE('',(#2659),#2039,.F.);
#23413=ADVANCED_FACE('',(#2660),#1319,.F.);
#23414=ADVANCED_FACE('',(#2661),#2040,.F.);
#23415=ADVANCED_FACE('',(#2662),#1320,.F.);
#23416=ADVANCED_FACE('',(#2663),#1321,.F.);
#23417=ADVANCED_FACE('',(#2664),#2041,.F.);
#23418=ADVANCED_FACE('',(#2665),#2042,.F.);
#23419=ADVANCED_FACE('',(#2666),#1322,.F.);
#23420=ADVANCED_FACE('',(#2667),#2043,.F.);
#23421=ADVANCED_FACE('',(#2668),#1323,.F.);
#23422=ADVANCED_FACE('',(#2669),#1324,.F.);
#23423=ADVANCED_FACE('',(#2670),#2044,.F.);
#23424=ADVANCED_FACE('',(#2671),#2045,.F.);
#23425=ADVANCED_FACE('',(#2672),#1325,.F.);
#23426=ADVANCED_FACE('',(#2673),#2046,.F.);
#23427=ADVANCED_FACE('',(#2674),#1326,.F.);
#23428=ADVANCED_FACE('',(#2675),#1327,.F.);
#23429=ADVANCED_FACE('',(#2676),#2047,.F.);
#23430=ADVANCED_FACE('',(#2677),#2048,.F.);
#23431=ADVANCED_FACE('',(#2678),#1328,.F.);
#23432=ADVANCED_FACE('',(#2679),#1329,.F.);
#23433=ADVANCED_FACE('',(#2680),#2049,.F.);
#23434=ADVANCED_FACE('',(#2681),#1330,.F.);
#23435=ADVANCED_FACE('',(#2682),#2050,.F.);
#23436=ADVANCED_FACE('',(#2683),#1331,.F.);
#23437=ADVANCED_FACE('',(#2684),#2051,.F.);
#23438=ADVANCED_FACE('',(#2685),#1332,.F.);
#23439=ADVANCED_FACE('',(#2686),#1333,.F.);
#23440=ADVANCED_FACE('',(#2687),#2052,.F.);
#23441=ADVANCED_FACE('',(#2688),#2053,.F.);
#23442=ADVANCED_FACE('',(#2689),#1334,.F.);
#23443=ADVANCED_FACE('',(#2690),#2054,.F.);
#23444=ADVANCED_FACE('',(#2691),#1335,.F.);
#23445=ADVANCED_FACE('',(#2692),#1336,.F.);
#23446=ADVANCED_FACE('',(#2693),#2055,.F.);
#23447=ADVANCED_FACE('',(#2694),#2056,.F.);
#23448=ADVANCED_FACE('',(#2695),#1337,.F.);
#23449=ADVANCED_FACE('',(#2696),#2057,.F.);
#23450=ADVANCED_FACE('',(#2697),#1338,.F.);
#23451=ADVANCED_FACE('',(#2698),#1339,.F.);
#23452=ADVANCED_FACE('',(#2699),#2058,.F.);
#23453=ADVANCED_FACE('',(#2700),#2059,.F.);
#23454=ADVANCED_FACE('',(#2701),#1340,.F.);
#23455=ADVANCED_FACE('',(#2702),#2060,.F.);
#23456=ADVANCED_FACE('',(#2703),#1341,.F.);
#23457=ADVANCED_FACE('',(#2704),#1342,.F.);
#23458=ADVANCED_FACE('',(#2705),#2061,.F.);
#23459=ADVANCED_FACE('',(#2706),#2062,.F.);
#23460=ADVANCED_FACE('',(#2707),#1343,.F.);
#23461=ADVANCED_FACE('',(#2708),#2063,.F.);
#23462=ADVANCED_FACE('',(#2709),#1344,.F.);
#23463=ADVANCED_FACE('',(#2710),#1345,.F.);
#23464=ADVANCED_FACE('',(#2711),#2064,.F.);
#23465=ADVANCED_FACE('',(#2712),#2065,.F.);
#23466=ADVANCED_FACE('',(#2713),#1346,.F.);
#23467=ADVANCED_FACE('',(#2714),#2066,.F.);
#23468=ADVANCED_FACE('',(#2715),#1347,.F.);
#23469=ADVANCED_FACE('',(#2716),#1348,.F.);
#23470=ADVANCED_FACE('',(#2717),#2067,.F.);
#23471=ADVANCED_FACE('',(#2718),#2068,.F.);
#23472=ADVANCED_FACE('',(#2719),#2069,.F.);
#23473=ADVANCED_FACE('',(#2720),#1349,.F.);
#23474=ADVANCED_FACE('',(#2721),#2070,.F.);
#23475=ADVANCED_FACE('',(#2722),#1350,.F.);
#23476=ADVANCED_FACE('',(#2723),#1351,.F.);
#23477=ADVANCED_FACE('',(#2724),#2071,.F.);
#23478=ADVANCED_FACE('',(#2725),#2072,.F.);
#23479=ADVANCED_FACE('',(#2726),#1352,.F.);
#23480=ADVANCED_FACE('',(#2727),#2073,.F.);
#23481=ADVANCED_FACE('',(#2728),#1353,.F.);
#23482=ADVANCED_FACE('',(#2729),#1354,.F.);
#23483=ADVANCED_FACE('',(#2730),#2074,.F.);
#23484=ADVANCED_FACE('',(#2731),#2075,.F.);
#23485=ADVANCED_FACE('',(#2732),#1355,.F.);
#23486=ADVANCED_FACE('',(#2733),#1356,.F.);
#23487=ADVANCED_FACE('',(#2734),#2076,.F.);
#23488=ADVANCED_FACE('',(#2735),#1357,.F.);
#23489=ADVANCED_FACE('',(#2736),#2077,.F.);
#23490=ADVANCED_FACE('',(#2737),#1358,.F.);
#23491=ADVANCED_FACE('',(#2738),#2078,.F.);
#23492=ADVANCED_FACE('',(#2739),#1359,.F.);
#23493=ADVANCED_FACE('',(#2740),#1360,.F.);
#23494=ADVANCED_FACE('',(#2741),#2079,.F.);
#23495=ADVANCED_FACE('',(#2742),#2080,.F.);
#23496=ADVANCED_FACE('',(#2743),#1361,.F.);
#23497=ADVANCED_FACE('',(#2744),#2081,.F.);
#23498=ADVANCED_FACE('',(#2745),#1362,.F.);
#23499=ADVANCED_FACE('',(#2746),#1363,.F.);
#23500=ADVANCED_FACE('',(#2747),#2082,.F.);
#23501=ADVANCED_FACE('',(#2748),#2083,.F.);
#23502=ADVANCED_FACE('',(#2749),#2084,.F.);
#23503=ADVANCED_FACE('',(#2750),#1364,.F.);
#23504=ADVANCED_FACE('',(#2751),#1365,.F.);
#23505=ADVANCED_FACE('',(#2752),#2085,.F.);
#23506=ADVANCED_FACE('',(#2753),#1366,.F.);
#23507=ADVANCED_FACE('',(#2754),#2086,.F.);
#23508=ADVANCED_FACE('',(#2755),#1367,.F.);
#23509=ADVANCED_FACE('',(#2756),#1368,.F.);
#23510=ADVANCED_FACE('',(#2757),#2087,.F.);
#23511=ADVANCED_FACE('',(#2758),#2088,.F.);
#23512=ADVANCED_FACE('',(#2759),#1369,.F.);
#23513=ADVANCED_FACE('',(#2760),#2089,.F.);
#23514=ADVANCED_FACE('',(#2761),#1370,.F.);
#23515=ADVANCED_FACE('',(#2762),#1371,.F.);
#23516=ADVANCED_FACE('',(#2763),#2090,.F.);
#23517=ADVANCED_FACE('',(#2764),#2091,.F.);
#23518=ADVANCED_FACE('',(#2765),#1372,.F.);
#23519=ADVANCED_FACE('',(#2766),#2092,.F.);
#23520=ADVANCED_FACE('',(#2767),#1373,.F.);
#23521=ADVANCED_FACE('',(#2768),#1374,.F.);
#23522=ADVANCED_FACE('',(#2769),#2093,.F.);
#23523=ADVANCED_FACE('',(#2770),#2094,.F.);
#23524=ADVANCED_FACE('',(#2771),#1375,.F.);
#23525=ADVANCED_FACE('',(#2772),#1376,.F.);
#23526=ADVANCED_FACE('',(#2773),#2095,.F.);
#23527=ADVANCED_FACE('',(#2774),#1377,.F.);
#23528=ADVANCED_FACE('',(#2775),#2096,.F.);
#23529=ADVANCED_FACE('',(#2776),#1378,.F.);
#23530=ADVANCED_FACE('',(#2777),#2097,.F.);
#23531=ADVANCED_FACE('',(#2778),#1379,.F.);
#23532=ADVANCED_FACE('',(#2779),#1380,.F.);
#23533=ADVANCED_FACE('',(#2780),#2098,.F.);
#23534=ADVANCED_FACE('',(#2781),#1381,.F.);
#23535=ADVANCED_FACE('',(#2782),#2099,.F.);
#23536=ADVANCED_FACE('',(#2783),#1382,.F.);
#23537=ADVANCED_FACE('',(#2784),#1383,.F.);
#23538=ADVANCED_FACE('',(#2785),#2100,.F.);
#23539=ADVANCED_FACE('',(#2786),#1384,.F.);
#23540=ADVANCED_FACE('',(#2787),#2101,.F.);
#23541=ADVANCED_FACE('',(#2788),#2102,.F.);
#23542=ADVANCED_FACE('',(#2789),#2103,.F.);
#23543=ADVANCED_FACE('',(#2790),#2104,.F.);
#23544=ADVANCED_FACE('',(#2791),#2105,.F.);
#23545=ADVANCED_FACE('',(#2792),#2106,.F.);
#23546=ADVANCED_FACE('',(#2793),#2107,.F.);
#23547=ADVANCED_FACE('',(#2794),#2108,.F.);
#23548=ADVANCED_FACE('',(#2795),#2109,.F.);
#23549=ADVANCED_FACE('',(#2796),#2110,.F.);
#23550=ADVANCED_FACE('',(#2797),#2111,.F.);
#23551=ADVANCED_FACE('',(#2798),#2112,.F.);
#23552=ADVANCED_FACE('',(#2799),#1385,.F.);
#23553=ADVANCED_FACE('',(#2800),#1386,.F.);
#23554=ADVANCED_FACE('',(#2801),#1387,.F.);
#23555=ADVANCED_FACE('',(#2802),#1388,.F.);
#23556=ADVANCED_FACE('',(#2803),#1389,.F.);
#23557=ADVANCED_FACE('',(#2804),#1390,.F.);
#23558=ADVANCED_FACE('',(#2805),#1391,.F.);
#23559=ADVANCED_FACE('',(#2806),#1392,.F.);
#23560=ADVANCED_FACE('',(#2807),#1393,.F.);
#23561=ADVANCED_FACE('',(#2808),#1394,.F.);
#23562=ADVANCED_FACE('',(#2809),#1395,.F.);
#23563=ADVANCED_FACE('',(#2810),#1396,.F.);
#23564=ADVANCED_FACE('',(#2811),#1397,.F.);
#23565=ADVANCED_FACE('',(#2812),#1398,.F.);
#23566=ADVANCED_FACE('',(#2813),#1399,.F.);
#23567=ADVANCED_FACE('',(#2814),#1400,.F.);
#23568=ADVANCED_FACE('',(#2815),#1401,.F.);
#23569=ADVANCED_FACE('',(#2816),#1402,.F.);
#23570=ADVANCED_FACE('',(#2817),#1403,.F.);
#23571=ADVANCED_FACE('',(#2818),#1404,.F.);
#23572=ADVANCED_FACE('',(#2819),#1405,.F.);
#23573=ADVANCED_FACE('',(#2820),#1406,.F.);
#23574=ADVANCED_FACE('',(#2821),#1407,.F.);
#23575=ADVANCED_FACE('',(#2822),#1408,.F.);
#23576=ADVANCED_FACE('',(#2823),#1409,.F.);
#23577=ADVANCED_FACE('',(#2824),#1410,.F.);
#23578=ADVANCED_FACE('',(#2825),#1411,.F.);
#23579=ADVANCED_FACE('',(#2826),#1412,.F.);
#23580=ADVANCED_FACE('',(#2827),#2113,.F.);
#23581=ADVANCED_FACE('',(#2828,#1157),#1413,.T.);
#23582=ADVANCED_FACE('',(#2829),#2114,.T.);
#23583=ADVANCED_FACE('',(#2830),#2115,.F.);
#24531=CLOSED_SHELL('',(#23297,#23298,#23299,#23300,#23301,#23302,#23303,
#23304,#23305,#23306,#23307,#23308,#23309,#23310,#23311,#23312,#23313,#23314,
#23315,#23316,#23317,#23318,#23319,#23320,#23321,#23322,#23323,#23324,#23325,
#23326,#23327,#23328,#23329,#23330,#23331,#23332,#23333,#23334,#23335,#23336,
#23337,#23338,#23339,#23340,#23341,#23342,#23343,#23344,#23345,#23346,#23347,
#23348,#23349,#23350,#23351,#23352,#23353,#23354,#23355,#23356,#23357,#23358,
#23359,#23360,#23361,#23362,#23363,#23364,#23365,#23366,#23367,#23368,#23369,
#23370,#23371,#23372,#23373,#23374,#23375,#23376,#23377,#23378,#23379,#23380,
#23381,#23382,#23383,#23384,#23385,#23386,#23387,#23388,#23389,#23390,#23391,
#23392,#23393,#23394,#23395,#23396,#23397,#23398,#23399,#23400,#23401,#23402,
#23403,#23404,#23405,#23406,#23407,#23408,#23409,#23410,#23411,#23412,#23413,
#23414,#23415,#23416,#23417,#23418,#23419,#23420,#23421,#23422,#23423,#23424,
#23425,#23426,#23427,#23428,#23429,#23430,#23431,#23432,#23433,#23434,#23435,
#23436,#23437,#23438,#23439,#23440,#23441,#23442,#23443,#23444,#23445,#23446,
#23447,#23448,#23449,#23450,#23451,#23452,#23453,#23454,#23455,#23456,#23457,
#23458,#23459,#23460,#23461,#23462,#23463,#23464,#23465,#23466,#23467,#23468,
#23469,#23470,#23471,#23472,#23473,#23474,#23475,#23476,#23477,#23478,#23479,
#23480,#23481,#23482,#23483,#23484,#23485,#23486,#23487,#23488,#23489,#23490,
#23491,#23492,#23493,#23494,#23495,#23496,#23497,#23498,#23499,#23500,#23501,
#23502,#23503,#23504,#23505,#23506,#23507,#23508,#23509,#23510,#23511,#23512,
#23513,#23514,#23515,#23516,#23517,#23518,#23519,#23520,#23521,#23522,#23523,
#23524,#23525,#23526,#23527,#23528,#23529,#23530,#23531,#23532,#23533,#23534,
#23535,#23536,#23537,#23538,#23539,#23540,#23541,#23542,#23543,#23544,#23545,
#23546,#23547,#23548,#23549,#23550,#23551,#23552,#23553,#23554,#23555,#23556,
#23557,#23558,#23559,#23560,#23561,#23562,#23563,#23564,#23565,#23566,#23567,
#23568,#23569,#23570,#23571,#23572,#23573,#23574,#23575,#23576,#23577,#23578,
#23579,#23580,#23581,#23582,#23583));
#25058=AXIS2_PLACEMENT_3D('',#34450,#27891,#27892);
#25059=AXIS2_PLACEMENT_3D('',#34451,#27893,#27894);
#25060=AXIS2_PLACEMENT_3D('',#34455,#27896,#27897);
#25061=AXIS2_PLACEMENT_3D('',#34456,#27898,#27899);
#25062=AXIS2_PLACEMENT_3D('',#34459,#27901,#27902);
#25063=AXIS2_PLACEMENT_3D('',#34460,#27903,#27904);
#25064=AXIS2_PLACEMENT_3D('',#34463,#27906,#27907);
#25065=AXIS2_PLACEMENT_3D('',#34464,#27908,#27909);
#25066=AXIS2_PLACEMENT_3D('',#34468,#27911,#27912);
#25067=AXIS2_PLACEMENT_3D('',#34469,#27913,#27914);
#25068=AXIS2_PLACEMENT_3D('',#34472,#27916,#27917);
#25069=AXIS2_PLACEMENT_3D('',#34473,#27918,#27919);
#25070=AXIS2_PLACEMENT_3D('',#34476,#27921,#27922);
#25071=AXIS2_PLACEMENT_3D('',#34477,#27923,#27924);
#25072=AXIS2_PLACEMENT_3D('',#34481,#27926,#27927);
#25073=AXIS2_PLACEMENT_3D('',#34482,#27928,#27929);
#25074=AXIS2_PLACEMENT_3D('',#34485,#27931,#27932);
#25075=AXIS2_PLACEMENT_3D('',#34486,#27933,#27934);
#25076=AXIS2_PLACEMENT_3D('',#34489,#27936,#27937);
#25077=AXIS2_PLACEMENT_3D('',#34490,#27938,#27939);
#25078=AXIS2_PLACEMENT_3D('',#34494,#27941,#27942);
#25079=AXIS2_PLACEMENT_3D('',#34495,#27943,#27944);
#25080=AXIS2_PLACEMENT_3D('',#34498,#27946,#27947);
#25081=AXIS2_PLACEMENT_3D('',#34499,#27948,#27949);
#25082=AXIS2_PLACEMENT_3D('',#34502,#27951,#27952);
#25083=AXIS2_PLACEMENT_3D('',#34503,#27953,#27954);
#25084=AXIS2_PLACEMENT_3D('',#34507,#27956,#27957);
#25085=AXIS2_PLACEMENT_3D('',#34508,#27958,#27959);
#25086=AXIS2_PLACEMENT_3D('',#34511,#27961,#27962);
#25087=AXIS2_PLACEMENT_3D('',#34512,#27963,#27964);
#25088=AXIS2_PLACEMENT_3D('',#34515,#27966,#27967);
#25089=AXIS2_PLACEMENT_3D('',#34516,#27968,#27969);
#25090=AXIS2_PLACEMENT_3D('',#34518,#27970,#27971);
#25091=AXIS2_PLACEMENT_3D('',#34521,#27973,#27974);
#25092=AXIS2_PLACEMENT_3D('',#34522,#27975,#27976);
#25093=AXIS2_PLACEMENT_3D('',#34525,#27978,#27979);
#25094=AXIS2_PLACEMENT_3D('',#34526,#27980,#27981);
#25095=AXIS2_PLACEMENT_3D('',#34529,#27983,#27984);
#25096=AXIS2_PLACEMENT_3D('',#34530,#27985,#27986);
#25097=AXIS2_PLACEMENT_3D('',#34532,#27987,#27988);
#25098=AXIS2_PLACEMENT_3D('',#34533,#27989,#27990);
#25099=AXIS2_PLACEMENT_3D('',#34536,#27992,#27993);
#25100=AXIS2_PLACEMENT_3D('',#34537,#27994,#27995);
#25101=AXIS2_PLACEMENT_3D('',#34539,#27996,#27997);
#25102=AXIS2_PLACEMENT_3D('',#34542,#27999,#28000);
#25103=AXIS2_PLACEMENT_3D('',#34543,#28001,#28002);
#25104=AXIS2_PLACEMENT_3D('',#34546,#28004,#28005);
#25105=AXIS2_PLACEMENT_3D('',#34547,#28006,#28007);
#25106=AXIS2_PLACEMENT_3D('',#34550,#28009,#28010);
#25107=AXIS2_PLACEMENT_3D('',#34551,#28011,#28012);
#25108=AXIS2_PLACEMENT_3D('',#34553,#28013,#28014);
#25109=AXIS2_PLACEMENT_3D('',#34554,#28015,#28016);
#25110=AXIS2_PLACEMENT_3D('',#34557,#28018,#28019);
#25111=AXIS2_PLACEMENT_3D('',#34558,#28020,#28021);
#25112=AXIS2_PLACEMENT_3D('',#34560,#28022,#28023);
#25113=AXIS2_PLACEMENT_3D('',#34563,#28025,#28026);
#25114=AXIS2_PLACEMENT_3D('',#34564,#28027,#28028);
#25115=AXIS2_PLACEMENT_3D('',#34567,#28030,#28031);
#25116=AXIS2_PLACEMENT_3D('',#34568,#28032,#28033);
#25117=AXIS2_PLACEMENT_3D('',#34571,#28035,#28036);
#25118=AXIS2_PLACEMENT_3D('',#34572,#28037,#28038);
#25119=AXIS2_PLACEMENT_3D('',#34574,#28039,#28040);
#25120=AXIS2_PLACEMENT_3D('',#34575,#28041,#28042);
#25121=AXIS2_PLACEMENT_3D('',#34578,#28044,#28045);
#25122=AXIS2_PLACEMENT_3D('',#34579,#28046,#28047);
#25123=AXIS2_PLACEMENT_3D('',#34581,#28048,#28049);
#25124=AXIS2_PLACEMENT_3D('',#34584,#28051,#28052);
#25125=AXIS2_PLACEMENT_3D('',#34585,#28053,#28054);
#25126=AXIS2_PLACEMENT_3D('',#34588,#28056,#28057);
#25127=AXIS2_PLACEMENT_3D('',#34589,#28058,#28059);
#25128=AXIS2_PLACEMENT_3D('',#34592,#28061,#28062);
#25129=AXIS2_PLACEMENT_3D('',#34593,#28063,#28064);
#25130=AXIS2_PLACEMENT_3D('',#34595,#28065,#28066);
#25131=AXIS2_PLACEMENT_3D('',#34596,#28067,#28068);
#25132=AXIS2_PLACEMENT_3D('',#34599,#28070,#28071);
#25133=AXIS2_PLACEMENT_3D('',#34600,#28072,#28073);
#25134=AXIS2_PLACEMENT_3D('',#34602,#28074,#28075);
#25135=AXIS2_PLACEMENT_3D('',#34605,#28077,#28078);
#25136=AXIS2_PLACEMENT_3D('',#34606,#28079,#28080);
#25137=AXIS2_PLACEMENT_3D('',#34609,#28082,#28083);
#25138=AXIS2_PLACEMENT_3D('',#34610,#28084,#28085);
#25139=AXIS2_PLACEMENT_3D('',#34613,#28087,#28088);
#25140=AXIS2_PLACEMENT_3D('',#34614,#28089,#28090);
#25141=AXIS2_PLACEMENT_3D('',#34616,#28091,#28092);
#25142=AXIS2_PLACEMENT_3D('',#34617,#28093,#28094);
#25143=AXIS2_PLACEMENT_3D('',#34620,#28096,#28097);
#25144=AXIS2_PLACEMENT_3D('',#34621,#28098,#28099);
#25145=AXIS2_PLACEMENT_3D('',#34623,#28100,#28101);
#25146=AXIS2_PLACEMENT_3D('',#34626,#28103,#28104);
#25147=AXIS2_PLACEMENT_3D('',#34627,#28105,#28106);
#25148=AXIS2_PLACEMENT_3D('',#34630,#28108,#28109);
#25149=AXIS2_PLACEMENT_3D('',#34631,#28110,#28111);
#25150=AXIS2_PLACEMENT_3D('',#34634,#28113,#28114);
#25151=AXIS2_PLACEMENT_3D('',#34635,#28115,#28116);
#25152=AXIS2_PLACEMENT_3D('',#34637,#28117,#28118);
#25153=AXIS2_PLACEMENT_3D('',#34638,#28119,#28120);
#25154=AXIS2_PLACEMENT_3D('',#34641,#28122,#28123);
#25155=AXIS2_PLACEMENT_3D('',#34642,#28124,#28125);
#25156=AXIS2_PLACEMENT_3D('',#34644,#28126,#28127);
#25157=AXIS2_PLACEMENT_3D('',#34647,#28129,#28130);
#25158=AXIS2_PLACEMENT_3D('',#34648,#28131,#28132);
#25159=AXIS2_PLACEMENT_3D('',#34651,#28134,#28135);
#25160=AXIS2_PLACEMENT_3D('',#34652,#28136,#28137);
#25161=AXIS2_PLACEMENT_3D('',#34655,#28139,#28140);
#25162=AXIS2_PLACEMENT_3D('',#34656,#28141,#28142);
#25163=AXIS2_PLACEMENT_3D('',#34658,#28143,#28144);
#25164=AXIS2_PLACEMENT_3D('',#34659,#28145,#28146);
#25165=AXIS2_PLACEMENT_3D('',#34662,#28148,#28149);
#25166=AXIS2_PLACEMENT_3D('',#34663,#28150,#28151);
#25167=AXIS2_PLACEMENT_3D('',#34665,#28152,#28153);
#25168=AXIS2_PLACEMENT_3D('',#34668,#28155,#28156);
#25169=AXIS2_PLACEMENT_3D('',#34669,#28157,#28158);
#25170=AXIS2_PLACEMENT_3D('',#34672,#28160,#28161);
#25171=AXIS2_PLACEMENT_3D('',#34673,#28162,#28163);
#25172=AXIS2_PLACEMENT_3D('',#34676,#28165,#28166);
#25173=AXIS2_PLACEMENT_3D('',#34677,#28167,#28168);
#25174=AXIS2_PLACEMENT_3D('',#34679,#28169,#28170);
#25175=AXIS2_PLACEMENT_3D('',#34680,#28171,#28172);
#25176=AXIS2_PLACEMENT_3D('',#34683,#28174,#28175);
#25177=AXIS2_PLACEMENT_3D('',#34684,#28176,#28177);
#25178=AXIS2_PLACEMENT_3D('',#34686,#28178,#28179);
#25179=AXIS2_PLACEMENT_3D('',#34689,#28181,#28182);
#25180=AXIS2_PLACEMENT_3D('',#34690,#28183,#28184);
#25181=AXIS2_PLACEMENT_3D('',#34693,#28186,#28187);
#25182=AXIS2_PLACEMENT_3D('',#34694,#28188,#28189);
#25183=AXIS2_PLACEMENT_3D('',#34697,#28191,#28192);
#25184=AXIS2_PLACEMENT_3D('',#34698,#28193,#28194);
#25185=AXIS2_PLACEMENT_3D('',#34700,#28195,#28196);
#25186=AXIS2_PLACEMENT_3D('',#34701,#28197,#28198);
#25187=AXIS2_PLACEMENT_3D('',#34704,#28200,#28201);
#25188=AXIS2_PLACEMENT_3D('',#34705,#28202,#28203);
#25189=AXIS2_PLACEMENT_3D('',#34707,#28204,#28205);
#25190=AXIS2_PLACEMENT_3D('',#34710,#28207,#28208);
#25191=AXIS2_PLACEMENT_3D('',#34711,#28209,#28210);
#25192=AXIS2_PLACEMENT_3D('',#34714,#28212,#28213);
#25193=AXIS2_PLACEMENT_3D('',#34715,#28214,#28215);
#25194=AXIS2_PLACEMENT_3D('',#34718,#28217,#28218);
#25195=AXIS2_PLACEMENT_3D('',#34719,#28219,#28220);
#25196=AXIS2_PLACEMENT_3D('',#34721,#28221,#28222);
#25197=AXIS2_PLACEMENT_3D('',#34722,#28223,#28224);
#25198=AXIS2_PLACEMENT_3D('',#34725,#28226,#28227);
#25199=AXIS2_PLACEMENT_3D('',#34726,#28228,#28229);
#25200=AXIS2_PLACEMENT_3D('',#34728,#28230,#28231);
#25201=AXIS2_PLACEMENT_3D('',#34731,#28233,#28234);
#25202=AXIS2_PLACEMENT_3D('',#34732,#28235,#28236);
#25203=AXIS2_PLACEMENT_3D('',#34735,#28238,#28239);
#25204=AXIS2_PLACEMENT_3D('',#34736,#28240,#28241);
#25205=AXIS2_PLACEMENT_3D('',#34739,#28243,#28244);
#25206=AXIS2_PLACEMENT_3D('',#34740,#28245,#28246);
#25207=AXIS2_PLACEMENT_3D('',#34742,#28247,#28248);
#25208=AXIS2_PLACEMENT_3D('',#34743,#28249,#28250);
#25209=AXIS2_PLACEMENT_3D('',#34746,#28252,#28253);
#25210=AXIS2_PLACEMENT_3D('',#34747,#28254,#28255);
#25211=AXIS2_PLACEMENT_3D('',#34749,#28256,#28257);
#25212=AXIS2_PLACEMENT_3D('',#34752,#28259,#28260);
#25213=AXIS2_PLACEMENT_3D('',#34753,#28261,#28262);
#25214=AXIS2_PLACEMENT_3D('',#34756,#28264,#28265);
#25215=AXIS2_PLACEMENT_3D('',#34757,#28266,#28267);
#25216=AXIS2_PLACEMENT_3D('',#34760,#28269,#28270);
#25217=AXIS2_PLACEMENT_3D('',#34761,#28271,#28272);
#25218=AXIS2_PLACEMENT_3D('',#34763,#28273,#28274);
#25219=AXIS2_PLACEMENT_3D('',#34764,#28275,#28276);
#25220=AXIS2_PLACEMENT_3D('',#34767,#28278,#28279);
#25221=AXIS2_PLACEMENT_3D('',#34768,#28280,#28281);
#25222=AXIS2_PLACEMENT_3D('',#34770,#28282,#28283);
#25223=AXIS2_PLACEMENT_3D('',#34774,#28285,#28286);
#25224=AXIS2_PLACEMENT_3D('',#34775,#28287,#28288);
#25225=AXIS2_PLACEMENT_3D('',#34776,#28289,#28290);
#25226=AXIS2_PLACEMENT_3D('',#34779,#28291,#28292);
#25227=AXIS2_PLACEMENT_3D('',#34780,#28293,#28294);
#25228=AXIS2_PLACEMENT_3D('',#34782,#28296,#28297);
#25229=AXIS2_PLACEMENT_3D('',#34784,#28298,#28299);
#25230=AXIS2_PLACEMENT_3D('',#34785,#28300,#28301);
#25231=AXIS2_PLACEMENT_3D('',#34788,#28303,#28304);
#25232=AXIS2_PLACEMENT_3D('',#34789,#28305,#28306);
#25233=AXIS2_PLACEMENT_3D('',#34791,#28307,#28308);
#25234=AXIS2_PLACEMENT_3D('',#34792,#28309,#28310);
#25235=AXIS2_PLACEMENT_3D('',#34795,#28311,#28312);
#25236=AXIS2_PLACEMENT_3D('',#34796,#28313,#28314);
#25237=AXIS2_PLACEMENT_3D('',#34799,#28316,#28317);
#25238=AXIS2_PLACEMENT_3D('',#34800,#28318,#28319);
#25239=AXIS2_PLACEMENT_3D('',#34803,#28320,#28321);
#25240=AXIS2_PLACEMENT_3D('',#34804,#28322,#28323);
#25241=AXIS2_PLACEMENT_3D('',#34806,#28325,#28326);
#25242=AXIS2_PLACEMENT_3D('',#34808,#28327,#28328);
#25243=AXIS2_PLACEMENT_3D('',#34809,#28329,#28330);
#25244=AXIS2_PLACEMENT_3D('',#34811,#28331,#28332);
#25245=AXIS2_PLACEMENT_3D('',#34813,#28334,#28335);
#25246=AXIS2_PLACEMENT_3D('',#34818,#28337,#28338);
#25247=AXIS2_PLACEMENT_3D('',#34822,#28340,#28341);
#25248=AXIS2_PLACEMENT_3D('',#34823,#28342,#28343);
#25249=AXIS2_PLACEMENT_3D('',#34826,#28344,#28345);
#25250=AXIS2_PLACEMENT_3D('',#34830,#28347,#28348);
#25251=AXIS2_PLACEMENT_3D('',#34833,#28350,#28351);
#25252=AXIS2_PLACEMENT_3D('',#34838,#28353,#28354);
#25253=AXIS2_PLACEMENT_3D('',#34842,#28356,#28357);
#25254=AXIS2_PLACEMENT_3D('',#34843,#28358,#28359);
#25255=AXIS2_PLACEMENT_3D('',#34846,#28360,#28361);
#25256=AXIS2_PLACEMENT_3D('',#34848,#28362,#28363);
#25257=AXIS2_PLACEMENT_3D('',#34852,#28365,#28366);
#25258=AXIS2_PLACEMENT_3D('',#34858,#28369,#28370);
#25259=AXIS2_PLACEMENT_3D('',#34862,#28372,#28373);
#25260=AXIS2_PLACEMENT_3D('',#34863,#28374,#28375);
#25261=AXIS2_PLACEMENT_3D('',#34866,#28376,#28377);
#25262=AXIS2_PLACEMENT_3D('',#34870,#28379,#28380);
#25263=AXIS2_PLACEMENT_3D('',#34873,#28382,#28383);
#25264=AXIS2_PLACEMENT_3D('',#34878,#28385,#28386);
#25265=AXIS2_PLACEMENT_3D('',#34882,#28388,#28389);
#25266=AXIS2_PLACEMENT_3D('',#34883,#28390,#28391);
#25267=AXIS2_PLACEMENT_3D('',#34886,#28392,#28393);
#25268=AXIS2_PLACEMENT_3D('',#34888,#28394,#28395);
#25269=AXIS2_PLACEMENT_3D('',#34892,#28397,#28398);
#25270=AXIS2_PLACEMENT_3D('',#34898,#28401,#28402);
#25271=AXIS2_PLACEMENT_3D('',#34902,#28404,#28405);
#25272=AXIS2_PLACEMENT_3D('',#34903,#28406,#28407);
#25273=AXIS2_PLACEMENT_3D('',#34906,#28408,#28409);
#25274=AXIS2_PLACEMENT_3D('',#34910,#28411,#28412);
#25275=AXIS2_PLACEMENT_3D('',#34913,#28414,#28415);
#25276=AXIS2_PLACEMENT_3D('',#34918,#28417,#28418);
#25277=AXIS2_PLACEMENT_3D('',#34922,#28420,#28421);
#25278=AXIS2_PLACEMENT_3D('',#34923,#28422,#28423);
#25279=AXIS2_PLACEMENT_3D('',#34926,#28424,#28425);
#25280=AXIS2_PLACEMENT_3D('',#34928,#28426,#28427);
#25281=AXIS2_PLACEMENT_3D('',#34932,#28429,#28430);
#25282=AXIS2_PLACEMENT_3D('',#34938,#28433,#28434);
#25283=AXIS2_PLACEMENT_3D('',#34942,#28436,#28437);
#25284=AXIS2_PLACEMENT_3D('',#34945,#28439,#28440);
#25285=AXIS2_PLACEMENT_3D('',#34950,#28442,#28443);
#25286=AXIS2_PLACEMENT_3D('',#34954,#28445,#28446);
#25287=AXIS2_PLACEMENT_3D('',#34957,#28448,#28449);
#25288=AXIS2_PLACEMENT_3D('',#34962,#28451,#28452);
#25289=AXIS2_PLACEMENT_3D('',#34966,#28454,#28455);
#25290=AXIS2_PLACEMENT_3D('',#34969,#28457,#28458);
#25291=AXIS2_PLACEMENT_3D('',#34974,#28460,#28461);
#25292=AXIS2_PLACEMENT_3D('',#34978,#28463,#28464);
#25293=AXIS2_PLACEMENT_3D('',#34981,#28466,#28467);
#25294=AXIS2_PLACEMENT_3D('',#34986,#28469,#28470);
#25295=AXIS2_PLACEMENT_3D('',#34990,#28472,#28473);
#25296=AXIS2_PLACEMENT_3D('',#34993,#28475,#28476);
#25297=AXIS2_PLACEMENT_3D('',#34998,#28478,#28479);
#25298=AXIS2_PLACEMENT_3D('',#35002,#28481,#28482);
#25299=AXIS2_PLACEMENT_3D('',#35005,#28484,#28485);
#25300=AXIS2_PLACEMENT_3D('',#35010,#28487,#28488);
#25301=AXIS2_PLACEMENT_3D('',#35014,#28490,#28491);
#25302=AXIS2_PLACEMENT_3D('',#35017,#28493,#28494);
#25303=AXIS2_PLACEMENT_3D('',#35022,#28496,#28497);
#25304=AXIS2_PLACEMENT_3D('',#35026,#28499,#28500);
#25305=AXIS2_PLACEMENT_3D('',#35029,#28502,#28503);
#25306=AXIS2_PLACEMENT_3D('',#35034,#28505,#28506);
#25307=AXIS2_PLACEMENT_3D('',#35038,#28508,#28509);
#25308=AXIS2_PLACEMENT_3D('',#35041,#28511,#28512);
#25309=AXIS2_PLACEMENT_3D('',#35046,#28514,#28515);
#25310=AXIS2_PLACEMENT_3D('',#35050,#28517,#28518);
#25311=AXIS2_PLACEMENT_3D('',#35053,#28520,#28521);
#25312=AXIS2_PLACEMENT_3D('',#35058,#28523,#28524);
#25313=AXIS2_PLACEMENT_3D('',#35062,#28526,#28527);
#25314=AXIS2_PLACEMENT_3D('',#35065,#28529,#28530);
#25315=AXIS2_PLACEMENT_3D('',#35070,#28532,#28533);
#25316=AXIS2_PLACEMENT_3D('',#35074,#28535,#28536);
#25317=AXIS2_PLACEMENT_3D('',#35077,#28538,#28539);
#25318=AXIS2_PLACEMENT_3D('',#35082,#28541,#28542);
#25319=AXIS2_PLACEMENT_3D('',#35086,#28544,#28545);
#25320=AXIS2_PLACEMENT_3D('',#35089,#28547,#28548);
#25321=AXIS2_PLACEMENT_3D('',#35094,#28550,#28551);
#25322=AXIS2_PLACEMENT_3D('',#35098,#28553,#28554);
#25323=AXIS2_PLACEMENT_3D('',#35101,#28556,#28557);
#25324=AXIS2_PLACEMENT_3D('',#35106,#28559,#28560);
#25325=AXIS2_PLACEMENT_3D('',#35110,#28562,#28563);
#25326=AXIS2_PLACEMENT_3D('',#35113,#28565,#28566);
#25327=AXIS2_PLACEMENT_3D('',#35118,#28568,#28569);
#25328=AXIS2_PLACEMENT_3D('',#35122,#28571,#28572);
#25329=AXIS2_PLACEMENT_3D('',#35125,#28574,#28575);
#25330=AXIS2_PLACEMENT_3D('',#35130,#28577,#28578);
#25331=AXIS2_PLACEMENT_3D('',#35134,#28580,#28581);
#25332=AXIS2_PLACEMENT_3D('',#35137,#28583,#28584);
#25333=AXIS2_PLACEMENT_3D('',#35142,#28586,#28587);
#25334=AXIS2_PLACEMENT_3D('',#35146,#28589,#28590);
#25335=AXIS2_PLACEMENT_3D('',#35149,#28592,#28593);
#25336=AXIS2_PLACEMENT_3D('',#35151,#28594,#28595);
#25337=AXIS2_PLACEMENT_3D('',#35152,#28596,#28597);
#25338=AXIS2_PLACEMENT_3D('',#35156,#28599,#28600);
#25339=AXIS2_PLACEMENT_3D('',#35158,#28602,#28603);
#25340=AXIS2_PLACEMENT_3D('',#35161,#28604,#28605);
#25341=AXIS2_PLACEMENT_3D('',#35164,#28608,#28609);
#25342=AXIS2_PLACEMENT_3D('',#35168,#28612,#28613);
#25343=AXIS2_PLACEMENT_3D('',#35171,#28614,#28615);
#25344=AXIS2_PLACEMENT_3D('',#35174,#28618,#28619);
#25345=AXIS2_PLACEMENT_3D('',#35176,#28621,#28622);
#25346=AXIS2_PLACEMENT_3D('',#35177,#28623,#28624);
#25347=AXIS2_PLACEMENT_3D('',#35180,#28625,#28626);
#25348=AXIS2_PLACEMENT_3D('',#35183,#28629,#28630);
#25349=AXIS2_PLACEMENT_3D('',#35187,#28633,#28634);
#25350=AXIS2_PLACEMENT_3D('',#35190,#28635,#28636);
#25351=AXIS2_PLACEMENT_3D('',#35193,#28639,#28640);
#25352=AXIS2_PLACEMENT_3D('',#35197,#28643,#28644);
#25353=AXIS2_PLACEMENT_3D('',#35198,#28645,#28646);
#25354=AXIS2_PLACEMENT_3D('',#35200,#28648,#28649);
#25355=AXIS2_PLACEMENT_3D('',#35201,#28650,#28651);
#25356=AXIS2_PLACEMENT_3D('',#35204,#28652,#28653);
#25357=AXIS2_PLACEMENT_3D('',#35207,#28656,#28657);
#25358=AXIS2_PLACEMENT_3D('',#35211,#28660,#28661);
#25359=AXIS2_PLACEMENT_3D('',#35214,#28662,#28663);
#25360=AXIS2_PLACEMENT_3D('',#35217,#28666,#28667);
#25361=AXIS2_PLACEMENT_3D('',#35221,#28670,#28671);
#25362=AXIS2_PLACEMENT_3D('',#35222,#28672,#28673);
#25363=AXIS2_PLACEMENT_3D('',#35224,#28675,#28676);
#25364=AXIS2_PLACEMENT_3D('',#35225,#28677,#28678);
#25365=AXIS2_PLACEMENT_3D('',#35229,#28680,#28681);
#25366=AXIS2_PLACEMENT_3D('',#35231,#28683,#28684);
#25367=AXIS2_PLACEMENT_3D('',#35234,#28685,#28686);
#25368=AXIS2_PLACEMENT_3D('',#35237,#28689,#28690);
#25369=AXIS2_PLACEMENT_3D('',#35241,#28693,#28694);
#25370=AXIS2_PLACEMENT_3D('',#35244,#28695,#28696);
#25371=AXIS2_PLACEMENT_3D('',#35247,#28699,#28700);
#25372=AXIS2_PLACEMENT_3D('',#35251,#28703,#28704);
#25373=AXIS2_PLACEMENT_3D('',#35252,#28705,#28706);
#25374=AXIS2_PLACEMENT_3D('',#35254,#28708,#28709);
#25375=AXIS2_PLACEMENT_3D('',#35255,#28710,#28711);
#25376=AXIS2_PLACEMENT_3D('',#35258,#28712,#28713);
#25377=AXIS2_PLACEMENT_3D('',#35261,#28716,#28717);
#25378=AXIS2_PLACEMENT_3D('',#35265,#28720,#28721);
#25379=AXIS2_PLACEMENT_3D('',#35268,#28722,#28723);
#25380=AXIS2_PLACEMENT_3D('',#35271,#28726,#28727);
#25381=AXIS2_PLACEMENT_3D('',#35275,#28730,#28731);
#25382=AXIS2_PLACEMENT_3D('',#35276,#28732,#28733);
#25383=AXIS2_PLACEMENT_3D('',#35278,#28735,#28736);
#25384=AXIS2_PLACEMENT_3D('',#35279,#28737,#28738);
#25385=AXIS2_PLACEMENT_3D('',#35282,#28739,#28740);
#25386=AXIS2_PLACEMENT_3D('',#35285,#28743,#28744);
#25387=AXIS2_PLACEMENT_3D('',#35289,#28747,#28748);
#25388=AXIS2_PLACEMENT_3D('',#35292,#28749,#28750);
#25389=AXIS2_PLACEMENT_3D('',#35295,#28753,#28754);
#25390=AXIS2_PLACEMENT_3D('',#35299,#28756,#28757);
#25391=AXIS2_PLACEMENT_3D('',#35301,#28758,#28759);
#25392=AXIS2_PLACEMENT_3D('',#35303,#28761,#28762);
#25393=AXIS2_PLACEMENT_3D('',#35305,#28764,#28765);
#25394=AXIS2_PLACEMENT_3D('',#35307,#28767,#28768);
#25395=AXIS2_PLACEMENT_3D('',#35310,#28769,#28770);
#25396=AXIS2_PLACEMENT_3D('',#35313,#28773,#28774);
#25397=AXIS2_PLACEMENT_3D('',#35317,#28777,#28778);
#25398=AXIS2_PLACEMENT_3D('',#35320,#28779,#28780);
#25399=AXIS2_PLACEMENT_3D('',#35323,#28783,#28784);
#25400=AXIS2_PLACEMENT_3D('',#35327,#28787,#28788);
#25401=AXIS2_PLACEMENT_3D('',#35328,#28789,#28790);
#25402=AXIS2_PLACEMENT_3D('',#35330,#28792,#28793);
#25403=AXIS2_PLACEMENT_3D('',#35331,#28794,#28795);
#25404=AXIS2_PLACEMENT_3D('',#35334,#28796,#28797);
#25405=AXIS2_PLACEMENT_3D('',#35337,#28800,#28801);
#25406=AXIS2_PLACEMENT_3D('',#35341,#28804,#28805);
#25407=AXIS2_PLACEMENT_3D('',#35344,#28806,#28807);
#25408=AXIS2_PLACEMENT_3D('',#35347,#28810,#28811);
#25409=AXIS2_PLACEMENT_3D('',#35351,#28814,#28815);
#25410=AXIS2_PLACEMENT_3D('',#35352,#28816,#28817);
#25411=AXIS2_PLACEMENT_3D('',#35354,#28819,#28820);
#25412=AXIS2_PLACEMENT_3D('',#35355,#28821,#28822);
#25413=AXIS2_PLACEMENT_3D('',#35359,#28824,#28825);
#25414=AXIS2_PLACEMENT_3D('',#35361,#28827,#28828);
#25415=AXIS2_PLACEMENT_3D('',#35365,#28830,#28831);
#25416=AXIS2_PLACEMENT_3D('',#35368,#28833,#28834);
#25417=AXIS2_PLACEMENT_3D('',#35369,#28835,#28836);
#25418=AXIS2_PLACEMENT_3D('',#35371,#28838,#28839);
#25419=AXIS2_PLACEMENT_3D('',#35373,#28841,#28842);
#25420=AXIS2_PLACEMENT_3D('',#35375,#28844,#28845);
#25421=AXIS2_PLACEMENT_3D('',#35378,#28846,#28847);
#25422=AXIS2_PLACEMENT_3D('',#35381,#28850,#28851);
#25423=AXIS2_PLACEMENT_3D('',#35385,#28854,#28855);
#25424=AXIS2_PLACEMENT_3D('',#35388,#28856,#28857);
#25425=AXIS2_PLACEMENT_3D('',#35391,#28860,#28861);
#25426=AXIS2_PLACEMENT_3D('',#35395,#28864,#28865);
#25427=AXIS2_PLACEMENT_3D('',#35396,#28866,#28867);
#25428=AXIS2_PLACEMENT_3D('',#35398,#28869,#28870);
#25429=AXIS2_PLACEMENT_3D('',#35399,#28871,#28872);
#25430=AXIS2_PLACEMENT_3D('',#35402,#28873,#28874);
#25431=AXIS2_PLACEMENT_3D('',#35405,#28877,#28878);
#25432=AXIS2_PLACEMENT_3D('',#35409,#28881,#28882);
#25433=AXIS2_PLACEMENT_3D('',#35412,#28883,#28884);
#25434=AXIS2_PLACEMENT_3D('',#35415,#28887,#28888);
#25435=AXIS2_PLACEMENT_3D('',#35419,#28891,#28892);
#25436=AXIS2_PLACEMENT_3D('',#35420,#28893,#28894);
#25437=AXIS2_PLACEMENT_3D('',#35422,#28896,#28897);
#25438=AXIS2_PLACEMENT_3D('',#35423,#28898,#28899);
#25439=AXIS2_PLACEMENT_3D('',#35426,#28900,#28901);
#25440=AXIS2_PLACEMENT_3D('',#35429,#28904,#28905);
#25441=AXIS2_PLACEMENT_3D('',#35433,#28908,#28909);
#25442=AXIS2_PLACEMENT_3D('',#35436,#28910,#28911);
#25443=AXIS2_PLACEMENT_3D('',#35439,#28914,#28915);
#25444=AXIS2_PLACEMENT_3D('',#35443,#28917,#28918);
#25445=AXIS2_PLACEMENT_3D('',#35445,#28919,#28920);
#25446=AXIS2_PLACEMENT_3D('',#35447,#28922,#28923);
#25447=AXIS2_PLACEMENT_3D('',#35449,#28925,#28926);
#25448=AXIS2_PLACEMENT_3D('',#35451,#28928,#28929);
#25449=AXIS2_PLACEMENT_3D('',#35454,#28930,#28931);
#25450=AXIS2_PLACEMENT_3D('',#35457,#28934,#28935);
#25451=AXIS2_PLACEMENT_3D('',#35461,#28938,#28939);
#25452=AXIS2_PLACEMENT_3D('',#35464,#28940,#28941);
#25453=AXIS2_PLACEMENT_3D('',#35467,#28944,#28945);
#25454=AXIS2_PLACEMENT_3D('',#35471,#28948,#28949);
#25455=AXIS2_PLACEMENT_3D('',#35472,#28950,#28951);
#25456=AXIS2_PLACEMENT_3D('',#35474,#28953,#28954);
#25457=AXIS2_PLACEMENT_3D('',#35475,#28955,#28956);
#25458=AXIS2_PLACEMENT_3D('',#35478,#28957,#28958);
#25459=AXIS2_PLACEMENT_3D('',#35481,#28961,#28962);
#25460=AXIS2_PLACEMENT_3D('',#35485,#28965,#28966);
#25461=AXIS2_PLACEMENT_3D('',#35488,#28967,#28968);
#25462=AXIS2_PLACEMENT_3D('',#35491,#28971,#28972);
#25463=AXIS2_PLACEMENT_3D('',#35495,#28975,#28976);
#25464=AXIS2_PLACEMENT_3D('',#35496,#28977,#28978);
#25465=AXIS2_PLACEMENT_3D('',#35498,#28980,#28981);
#25466=AXIS2_PLACEMENT_3D('',#35499,#28982,#28983);
#25467=AXIS2_PLACEMENT_3D('',#35502,#28984,#28985);
#25468=AXIS2_PLACEMENT_3D('',#35505,#28988,#28989);
#25469=AXIS2_PLACEMENT_3D('',#35509,#28992,#28993);
#25470=AXIS2_PLACEMENT_3D('',#35512,#28994,#28995);
#25471=AXIS2_PLACEMENT_3D('',#35515,#28998,#28999);
#25472=AXIS2_PLACEMENT_3D('',#35519,#29002,#29003);
#25473=AXIS2_PLACEMENT_3D('',#35520,#29004,#29005);
#25474=AXIS2_PLACEMENT_3D('',#35522,#29007,#29008);
#25475=AXIS2_PLACEMENT_3D('',#35523,#29009,#29010);
#25476=AXIS2_PLACEMENT_3D('',#35527,#29012,#29013);
#25477=AXIS2_PLACEMENT_3D('',#35529,#29015,#29016);
#25478=AXIS2_PLACEMENT_3D('',#35532,#29017,#29018);
#25479=AXIS2_PLACEMENT_3D('',#35535,#29021,#29022);
#25480=AXIS2_PLACEMENT_3D('',#35539,#29025,#29026);
#25481=AXIS2_PLACEMENT_3D('',#35542,#29027,#29028);
#25482=AXIS2_PLACEMENT_3D('',#35545,#29031,#29032);
#25483=AXIS2_PLACEMENT_3D('',#35549,#29035,#29036);
#25484=AXIS2_PLACEMENT_3D('',#35550,#29037,#29038);
#25485=AXIS2_PLACEMENT_3D('',#35552,#29040,#29041);
#25486=AXIS2_PLACEMENT_3D('',#35553,#29042,#29043);
#25487=AXIS2_PLACEMENT_3D('',#35556,#29044,#29045);
#25488=AXIS2_PLACEMENT_3D('',#35559,#29048,#29049);
#25489=AXIS2_PLACEMENT_3D('',#35563,#29052,#29053);
#25490=AXIS2_PLACEMENT_3D('',#35566,#29054,#29055);
#25491=AXIS2_PLACEMENT_3D('',#35569,#29058,#29059);
#25492=AXIS2_PLACEMENT_3D('',#35573,#29062,#29063);
#25493=AXIS2_PLACEMENT_3D('',#35574,#29064,#29065);
#25494=AXIS2_PLACEMENT_3D('',#35576,#29067,#29068);
#25495=AXIS2_PLACEMENT_3D('',#35577,#29069,#29070);
#25496=AXIS2_PLACEMENT_3D('',#35581,#29072,#29073);
#25497=AXIS2_PLACEMENT_3D('',#35583,#29075,#29076);
#25498=AXIS2_PLACEMENT_3D('',#35587,#29078,#29079);
#25499=AXIS2_PLACEMENT_3D('',#35590,#29081,#29082);
#25500=AXIS2_PLACEMENT_3D('',#35591,#29083,#29084);
#25501=AXIS2_PLACEMENT_3D('',#35593,#29086,#29087);
#25502=AXIS2_PLACEMENT_3D('',#35595,#29089,#29090);
#25503=AXIS2_PLACEMENT_3D('',#35597,#29092,#29093);
#25504=AXIS2_PLACEMENT_3D('',#35600,#29094,#29095);
#25505=AXIS2_PLACEMENT_3D('',#35603,#29098,#29099);
#25506=AXIS2_PLACEMENT_3D('',#35607,#29102,#29103);
#25507=AXIS2_PLACEMENT_3D('',#35610,#29104,#29105);
#25508=AXIS2_PLACEMENT_3D('',#35613,#29108,#29109);
#25509=AXIS2_PLACEMENT_3D('',#35617,#29112,#29113);
#25510=AXIS2_PLACEMENT_3D('',#35618,#29114,#29115);
#25511=AXIS2_PLACEMENT_3D('',#35620,#29117,#29118);
#25512=AXIS2_PLACEMENT_3D('',#35621,#29119,#29120);
#25513=AXIS2_PLACEMENT_3D('',#35624,#29121,#29122);
#25514=AXIS2_PLACEMENT_3D('',#35627,#29125,#29126);
#25515=AXIS2_PLACEMENT_3D('',#35631,#29129,#29130);
#25516=AXIS2_PLACEMENT_3D('',#35634,#29131,#29132);
#25517=AXIS2_PLACEMENT_3D('',#35637,#29135,#29136);
#25518=AXIS2_PLACEMENT_3D('',#35641,#29139,#29140);
#25519=AXIS2_PLACEMENT_3D('',#35642,#29141,#29142);
#25520=AXIS2_PLACEMENT_3D('',#35644,#29144,#29145);
#25521=AXIS2_PLACEMENT_3D('',#35645,#29146,#29147);
#25522=AXIS2_PLACEMENT_3D('',#35649,#29149,#29150);
#25523=AXIS2_PLACEMENT_3D('',#35651,#29152,#29153);
#25524=AXIS2_PLACEMENT_3D('',#35654,#29154,#29155);
#25525=AXIS2_PLACEMENT_3D('',#35657,#29158,#29159);
#25526=AXIS2_PLACEMENT_3D('',#35661,#29162,#29163);
#25527=AXIS2_PLACEMENT_3D('',#35662,#29164,#29165);
#25528=AXIS2_PLACEMENT_3D('',#35664,#29167,#29168);
#25529=AXIS2_PLACEMENT_3D('',#35667,#29169,#29170);
#25530=AXIS2_PLACEMENT_3D('',#35670,#29173,#29174);
#25531=AXIS2_PLACEMENT_3D('',#35674,#29177,#29178);
#25532=AXIS2_PLACEMENT_3D('',#35677,#29179,#29180);
#25533=AXIS2_PLACEMENT_3D('',#35680,#29183,#29184);
#25534=AXIS2_PLACEMENT_3D('',#35684,#29187,#29188);
#25535=AXIS2_PLACEMENT_3D('',#35685,#29189,#29190);
#25536=AXIS2_PLACEMENT_3D('',#35687,#29192,#29193);
#25537=AXIS2_PLACEMENT_3D('',#35688,#29194,#29195);
#25538=AXIS2_PLACEMENT_3D('',#35691,#29196,#29197);
#25539=AXIS2_PLACEMENT_3D('',#35694,#29200,#29201);
#25540=AXIS2_PLACEMENT_3D('',#35698,#29204,#29205);
#25541=AXIS2_PLACEMENT_3D('',#35701,#29206,#29207);
#25542=AXIS2_PLACEMENT_3D('',#35704,#29210,#29211);
#25543=AXIS2_PLACEMENT_3D('',#35708,#29214,#29215);
#25544=AXIS2_PLACEMENT_3D('',#35709,#29216,#29217);
#25545=AXIS2_PLACEMENT_3D('',#35711,#29219,#29220);
#25546=AXIS2_PLACEMENT_3D('',#35712,#29221,#29222);
#25547=AXIS2_PLACEMENT_3D('',#35715,#29223,#29224);
#25548=AXIS2_PLACEMENT_3D('',#35718,#29227,#29228);
#25549=AXIS2_PLACEMENT_3D('',#35722,#29231,#29232);
#25550=AXIS2_PLACEMENT_3D('',#35725,#29233,#29234);
#25551=AXIS2_PLACEMENT_3D('',#35728,#29237,#29238);
#25552=AXIS2_PLACEMENT_3D('',#35732,#29241,#29242);
#25553=AXIS2_PLACEMENT_3D('',#35733,#29243,#29244);
#25554=AXIS2_PLACEMENT_3D('',#35735,#29246,#29247);
#25555=AXIS2_PLACEMENT_3D('',#35736,#29248,#29249);
#25556=AXIS2_PLACEMENT_3D('',#35739,#29250,#29251);
#25557=AXIS2_PLACEMENT_3D('',#35742,#29254,#29255);
#25558=AXIS2_PLACEMENT_3D('',#35746,#29258,#29259);
#25559=AXIS2_PLACEMENT_3D('',#35747,#29260,#29261);
#25560=AXIS2_PLACEMENT_3D('',#35749,#29263,#29264);
#25561=AXIS2_PLACEMENT_3D('',#35752,#29265,#29266);
#25562=AXIS2_PLACEMENT_3D('',#35755,#29269,#29270);
#25563=AXIS2_PLACEMENT_3D('',#35759,#29273,#29274);
#25564=AXIS2_PLACEMENT_3D('',#35762,#29275,#29276);
#25565=AXIS2_PLACEMENT_3D('',#35765,#29279,#29280);
#25566=AXIS2_PLACEMENT_3D('',#35767,#29282,#29283);
#25567=AXIS2_PLACEMENT_3D('',#35768,#29284,#29285);
#25568=AXIS2_PLACEMENT_3D('',#35771,#29286,#29287);
#25569=AXIS2_PLACEMENT_3D('',#35774,#29290,#29291);
#25570=AXIS2_PLACEMENT_3D('',#35778,#29294,#29295);
#25571=AXIS2_PLACEMENT_3D('',#35779,#29296,#29297);
#25572=AXIS2_PLACEMENT_3D('',#35781,#29299,#29300);
#25573=AXIS2_PLACEMENT_3D('',#35784,#29301,#29302);
#25574=AXIS2_PLACEMENT_3D('',#35787,#29305,#29306);
#25575=AXIS2_PLACEMENT_3D('',#35789,#29308,#29309);
#25576=AXIS2_PLACEMENT_3D('',#35790,#29310,#29311);
#25577=AXIS2_PLACEMENT_3D('',#35793,#29312,#29313);
#25578=AXIS2_PLACEMENT_3D('',#35796,#29316,#29317);
#25579=AXIS2_PLACEMENT_3D('',#35800,#29320,#29321);
#25580=AXIS2_PLACEMENT_3D('',#35801,#29322,#29323);
#25581=AXIS2_PLACEMENT_3D('',#35803,#29325,#29326);
#25582=AXIS2_PLACEMENT_3D('',#35806,#29327,#29328);
#25583=AXIS2_PLACEMENT_3D('',#35809,#29331,#29332);
#25584=AXIS2_PLACEMENT_3D('',#35811,#29334,#29335);
#25585=AXIS2_PLACEMENT_3D('',#35812,#29336,#29337);
#25586=AXIS2_PLACEMENT_3D('',#35813,#29338,#29339);
#25587=AXIS2_PLACEMENT_3D('',#35814,#29340,#29341);
#25588=AXIS2_PLACEMENT_3D('',#35815,#29342,#29343);
#25589=AXIS2_PLACEMENT_3D('',#35816,#29344,#29345);
#25590=AXIS2_PLACEMENT_3D('',#35817,#29346,#29347);
#25591=AXIS2_PLACEMENT_3D('',#35819,#29349,#29350);
#25592=AXIS2_PLACEMENT_3D('',#35820,#29351,#29352);
#25593=AXIS2_PLACEMENT_3D('',#35821,#29353,#29354);
#25594=AXIS2_PLACEMENT_3D('',#35822,#29355,#29356);
#25595=AXIS2_PLACEMENT_3D('',#35824,#29358,#29359);
#25596=AXIS2_PLACEMENT_3D('',#35825,#29360,#29361);
#25597=AXIS2_PLACEMENT_3D('',#35826,#29362,#29363);
#25598=AXIS2_PLACEMENT_3D('',#35827,#29364,#29365);
#25599=AXIS2_PLACEMENT_3D('',#35828,#29366,#29367);
#25600=AXIS2_PLACEMENT_3D('',#35829,#29368,#29369);
#25601=AXIS2_PLACEMENT_3D('',#35830,#29370,#29371);
#25602=AXIS2_PLACEMENT_3D('',#35831,#29372,#29373);
#25603=AXIS2_PLACEMENT_3D('',#35832,#29374,#29375);
#25604=AXIS2_PLACEMENT_3D('',#35833,#29376,#29377);
#25605=AXIS2_PLACEMENT_3D('',#35834,#29378,#29379);
#25606=AXIS2_PLACEMENT_3D('',#35835,#29380,#29381);
#25607=AXIS2_PLACEMENT_3D('',#35836,#29382,#29383);
#25608=AXIS2_PLACEMENT_3D('',#35837,#29384,#29385);
#25609=AXIS2_PLACEMENT_3D('',#35838,#29386,#29387);
#25610=AXIS2_PLACEMENT_3D('',#35839,#29388,#29389);
#25611=AXIS2_PLACEMENT_3D('',#35840,#29390,#29391);
#25612=AXIS2_PLACEMENT_3D('',#35841,#29392,#29393);
#25613=AXIS2_PLACEMENT_3D('',#35842,#29394,#29395);
#25614=AXIS2_PLACEMENT_3D('',#35843,#29396,#29397);
#25615=AXIS2_PLACEMENT_3D('',#35844,#29398,#29399);
#25616=AXIS2_PLACEMENT_3D('',#35845,#29400,#29401);
#25617=AXIS2_PLACEMENT_3D('',#35846,#29402,#29403);
#25618=AXIS2_PLACEMENT_3D('',#35847,#29404,#29405);
#25619=AXIS2_PLACEMENT_3D('',#35848,#29406,#29407);
#25620=AXIS2_PLACEMENT_3D('',#35849,#29408,#29409);
#25621=AXIS2_PLACEMENT_3D('',#35850,#29410,#29411);
#25622=AXIS2_PLACEMENT_3D('',#35851,#29412,#29413);
#25623=AXIS2_PLACEMENT_3D('',#35852,#29414,#29415);
#25624=AXIS2_PLACEMENT_3D('',#35853,#29416,#29417);
#25625=AXIS2_PLACEMENT_3D('',#35854,#29418,#29419);
#25626=AXIS2_PLACEMENT_3D('',#35857,#29421,#29422);
#25627=AXIS2_PLACEMENT_3D('',#35858,#29423,#29424);
#25628=AXIS2_PLACEMENT_3D('',#35860,#29425,#29426);
#25629=AXIS2_PLACEMENT_3D('',#35861,#29427,#29428);
#25630=AXIS2_PLACEMENT_3D('',#35863,#29430,#29431);
#27891=DIRECTION('axis',(0.,0.,1.));
#27892=DIRECTION('refdir',(1.,0.,0.));
#27893=DIRECTION('center_axis',(0.,0.,1.));
#27894=DIRECTION('ref_axis',(1.,0.,0.));
#27895=DIRECTION('',(-0.857167300702118,-1.04972719113863E-16,0.515038074910044));
#27896=DIRECTION('center_axis',(0.,0.,1.));
#27897=DIRECTION('ref_axis',(1.,0.,0.));
#27898=DIRECTION('center_axis',(0.,0.,1.));
#27899=DIRECTION('ref_axis',(1.,0.,0.));
#27900=DIRECTION('',(0.,0.,1.));
#27901=DIRECTION('center_axis',(0.,0.,1.));
#27902=DIRECTION('ref_axis',(1.,0.,0.));
#27903=DIRECTION('center_axis',(0.,0.,1.));
#27904=DIRECTION('ref_axis',(1.,0.,0.));
#27905=DIRECTION('',(-0.707106781186549,-8.65956056235495E-17,0.707106781186546));
#27906=DIRECTION('center_axis',(0.,0.,-1.));
#27907=DIRECTION('ref_axis',(1.,0.,0.));
#27908=DIRECTION('center_axis',(0.,0.,1.));
#27909=DIRECTION('ref_axis',(1.,0.,0.));
#27910=DIRECTION('',(-0.857167300702118,-1.04972719113863E-16,0.515038074910044));
#27911=DIRECTION('center_axis',(0.,0.,1.));
#27912=DIRECTION('ref_axis',(1.,0.,0.));
#27913=DIRECTION('center_axis',(0.,0.,1.));
#27914=DIRECTION('ref_axis',(1.,0.,0.));
#27915=DIRECTION('',(0.,0.,1.));
#27916=DIRECTION('center_axis',(0.,0.,1.));
#27917=DIRECTION('ref_axis',(1.,0.,0.));
#27918=DIRECTION('center_axis',(0.,0.,1.));
#27919=DIRECTION('ref_axis',(1.,0.,0.));
#27920=DIRECTION('',(-0.707106781186549,-8.65956056235495E-17,0.707106781186546));
#27921=DIRECTION('center_axis',(0.,0.,-1.));
#27922=DIRECTION('ref_axis',(1.,0.,0.));
#27923=DIRECTION('center_axis',(0.,0.,-1.));
#27924=DIRECTION('ref_axis',(-1.,0.,0.));
#27925=DIRECTION('',(0.857167300702116,-1.04972719113862E-16,-0.515038074910048));
#27926=DIRECTION('center_axis',(0.,0.,-1.));
#27927=DIRECTION('ref_axis',(1.,0.,0.));
#27928=DIRECTION('center_axis',(0.,0.,-1.));
#27929=DIRECTION('ref_axis',(-1.,0.,0.));
#27930=DIRECTION('',(0.,0.,-1.));
#27931=DIRECTION('center_axis',(0.,0.,-1.));
#27932=DIRECTION('ref_axis',(1.,0.,0.));
#27933=DIRECTION('center_axis',(0.,0.,-1.));
#27934=DIRECTION('ref_axis',(-1.,0.,0.));
#27935=DIRECTION('',(0.707106781186549,-8.65956056235495E-17,-0.707106781186546));
#27936=DIRECTION('center_axis',(0.,0.,1.));
#27937=DIRECTION('ref_axis',(-1.,0.,0.));
#27938=DIRECTION('center_axis',(0.,0.,-1.));
#27939=DIRECTION('ref_axis',(-1.,0.,0.));
#27940=DIRECTION('',(0.857167300702115,-1.04972719113862E-16,-0.51503807491005));
#27941=DIRECTION('center_axis',(0.,0.,-1.));
#27942=DIRECTION('ref_axis',(1.,0.,0.));
#27943=DIRECTION('center_axis',(0.,0.,-1.));
#27944=DIRECTION('ref_axis',(-1.,0.,0.));
#27945=DIRECTION('',(0.,0.,-1.));
#27946=DIRECTION('center_axis',(0.,0.,-1.));
#27947=DIRECTION('ref_axis',(1.,0.,0.));
#27948=DIRECTION('center_axis',(0.,0.,-1.));
#27949=DIRECTION('ref_axis',(-1.,0.,0.));
#27950=DIRECTION('',(0.707106781186549,-8.65956056235495E-17,-0.707106781186546));
#27951=DIRECTION('center_axis',(0.,0.,1.));
#27952=DIRECTION('ref_axis',(-1.,0.,0.));
#27953=DIRECTION('center_axis',(0.,0.,-1.));
#27954=DIRECTION('ref_axis',(-1.,0.,0.));
#27955=DIRECTION('',(0.857167300702115,-1.04972719113862E-16,-0.515038074910049));
#27956=DIRECTION('center_axis',(0.,0.,-1.));
#27957=DIRECTION('ref_axis',(1.,0.,0.));
#27958=DIRECTION('center_axis',(0.,0.,-1.));
#27959=DIRECTION('ref_axis',(-1.,0.,0.));
#27960=DIRECTION('',(0.,0.,-1.));
#27961=DIRECTION('center_axis',(0.,0.,-1.));
#27962=DIRECTION('ref_axis',(1.,0.,0.));
#27963=DIRECTION('center_axis',(0.,0.,-1.));
#27964=DIRECTION('ref_axis',(-1.,0.,0.));
#27965=DIRECTION('',(0.707106781186549,-8.65956056235495E-17,-0.707106781186546));
#27966=DIRECTION('center_axis',(0.,0.,1.));
#27967=DIRECTION('ref_axis',(-1.,0.,0.));
#27968=DIRECTION('center_axis',(0.,0.,-1.));
#27969=DIRECTION('ref_axis',(1.,0.,0.));
#27970=DIRECTION('center_axis',(0.,0.,1.));
#27971=DIRECTION('ref_axis',(1.,0.,0.));
#27972=DIRECTION('',(0.316227766016828,3.87267321454026E-17,0.948683298050517));
#27973=DIRECTION('center_axis',(0.,0.,1.));
#27974=DIRECTION('ref_axis',(1.,0.,0.));
#27975=DIRECTION('center_axis',(0.,0.,1.));
#27976=DIRECTION('ref_axis',(1.,0.,0.));
#27977=DIRECTION('',(0.,0.,1.));
#27978=DIRECTION('center_axis',(0.,0.,1.));
#27979=DIRECTION('ref_axis',(1.,0.,0.));
#27980=DIRECTION('center_axis',(0.,0.,1.));
#27981=DIRECTION('ref_axis',(1.,0.,0.));
#27982=DIRECTION('',(-0.70710678118656,-8.65956056235509E-17,0.707106781186535));
#27983=DIRECTION('center_axis',(0.,0.,1.));
#27984=DIRECTION('ref_axis',(1.,0.,0.));
#27985=DIRECTION('center_axis',(0.,0.,-1.));
#27986=DIRECTION('ref_axis',(-1.,0.,0.));
#27987=DIRECTION('center_axis',(0.,0.,1.));
#27988=DIRECTION('ref_axis',(1.,0.,0.));
#27989=DIRECTION('center_axis',(0.,0.,1.));
#27990=DIRECTION('ref_axis',(1.,0.,0.));
#27991=DIRECTION('',(0.,0.,1.));
#27992=DIRECTION('center_axis',(0.,0.,-1.));
#27993=DIRECTION('ref_axis',(1.,0.,0.));
#27994=DIRECTION('center_axis',(0.,0.,-1.));
#27995=DIRECTION('ref_axis',(1.,0.,0.));
#27996=DIRECTION('center_axis',(0.,0.,1.));
#27997=DIRECTION('ref_axis',(1.,0.,0.));
#27998=DIRECTION('',(0.316227766016838,3.87267321454039E-17,0.948683298050514));
#27999=DIRECTION('center_axis',(0.,0.,1.));
#28000=DIRECTION('ref_axis',(1.,0.,0.));
#28001=DIRECTION('center_axis',(0.,0.,1.));
#28002=DIRECTION('ref_axis',(1.,0.,0.));
#28003=DIRECTION('',(0.,0.,1.));
#28004=DIRECTION('center_axis',(0.,0.,1.));
#28005=DIRECTION('ref_axis',(1.,0.,0.));
#28006=DIRECTION('center_axis',(0.,0.,1.));
#28007=DIRECTION('ref_axis',(1.,0.,0.));
#28008=DIRECTION('',(-0.707106781186573,-8.65956056235524E-17,0.707106781186522));
#28009=DIRECTION('center_axis',(0.,0.,1.));
#28010=DIRECTION('ref_axis',(1.,0.,0.));
#28011=DIRECTION('center_axis',(0.,0.,-1.));
#28012=DIRECTION('ref_axis',(-1.,0.,0.));
#28013=DIRECTION('center_axis',(0.,0.,1.));
#28014=DIRECTION('ref_axis',(1.,0.,0.));
#28015=DIRECTION('center_axis',(0.,0.,1.));
#28016=DIRECTION('ref_axis',(1.,0.,0.));
#28017=DIRECTION('',(0.,0.,1.));
#28018=DIRECTION('center_axis',(0.,0.,-1.));
#28019=DIRECTION('ref_axis',(1.,0.,0.));
#28020=DIRECTION('center_axis',(0.,0.,-1.));
#28021=DIRECTION('ref_axis',(1.,0.,0.));
#28022=DIRECTION('center_axis',(0.,0.,1.));
#28023=DIRECTION('ref_axis',(1.,0.,0.));
#28024=DIRECTION('',(0.316227766016835,3.87267321454036E-17,0.948683298050515));
#28025=DIRECTION('center_axis',(0.,0.,1.));
#28026=DIRECTION('ref_axis',(1.,0.,0.));
#28027=DIRECTION('center_axis',(0.,0.,1.));
#28028=DIRECTION('ref_axis',(1.,0.,0.));
#28029=DIRECTION('',(0.,0.,1.));
#28030=DIRECTION('center_axis',(0.,0.,1.));
#28031=DIRECTION('ref_axis',(1.,0.,0.));
#28032=DIRECTION('center_axis',(0.,0.,1.));
#28033=DIRECTION('ref_axis',(1.,0.,0.));
#28034=DIRECTION('',(-0.70710678118657,-8.6595605623552E-17,0.707106781186526));
#28035=DIRECTION('center_axis',(0.,0.,1.));
#28036=DIRECTION('ref_axis',(1.,0.,0.));
#28037=DIRECTION('center_axis',(0.,0.,-1.));
#28038=DIRECTION('ref_axis',(-1.,0.,0.));
#28039=DIRECTION('center_axis',(0.,0.,1.));
#28040=DIRECTION('ref_axis',(1.,0.,0.));
#28041=DIRECTION('center_axis',(0.,0.,1.));
#28042=DIRECTION('ref_axis',(1.,0.,0.));
#28043=DIRECTION('',(0.,0.,1.));
#28044=DIRECTION('center_axis',(0.,0.,-1.));
#28045=DIRECTION('ref_axis',(1.,0.,0.));
#28046=DIRECTION('center_axis',(0.,0.,-1.));
#28047=DIRECTION('ref_axis',(1.,0.,0.));
#28048=DIRECTION('center_axis',(0.,0.,1.));
#28049=DIRECTION('ref_axis',(1.,0.,0.));
#28050=DIRECTION('',(0.316227766016833,3.87267321454033E-17,0.948683298050515));
#28051=DIRECTION('center_axis',(0.,0.,1.));
#28052=DIRECTION('ref_axis',(1.,0.,0.));
#28053=DIRECTION('center_axis',(0.,0.,1.));
#28054=DIRECTION('ref_axis',(1.,0.,0.));
#28055=DIRECTION('',(0.,0.,1.));
#28056=DIRECTION('center_axis',(0.,0.,1.));
#28057=DIRECTION('ref_axis',(1.,0.,0.));
#28058=DIRECTION('center_axis',(0.,0.,1.));
#28059=DIRECTION('ref_axis',(1.,0.,0.));
#28060=DIRECTION('',(-0.707106781186566,-8.65956056235516E-17,0.707106781186529));
#28061=DIRECTION('center_axis',(0.,0.,1.));
#28062=DIRECTION('ref_axis',(1.,0.,0.));
#28063=DIRECTION('center_axis',(0.,0.,-1.));
#28064=DIRECTION('ref_axis',(-1.,0.,0.));
#28065=DIRECTION('center_axis',(0.,0.,1.));
#28066=DIRECTION('ref_axis',(1.,0.,0.));
#28067=DIRECTION('center_axis',(0.,0.,1.));
#28068=DIRECTION('ref_axis',(1.,0.,0.));
#28069=DIRECTION('',(0.,0.,1.));
#28070=DIRECTION('center_axis',(0.,0.,-1.));
#28071=DIRECTION('ref_axis',(1.,0.,0.));
#28072=DIRECTION('center_axis',(0.,0.,-1.));
#28073=DIRECTION('ref_axis',(1.,0.,0.));
#28074=DIRECTION('center_axis',(0.,0.,1.));
#28075=DIRECTION('ref_axis',(1.,0.,0.));
#28076=DIRECTION('',(0.316227766016833,3.87267321454033E-17,0.948683298050515));
#28077=DIRECTION('center_axis',(0.,0.,1.));
#28078=DIRECTION('ref_axis',(1.,0.,0.));
#28079=DIRECTION('center_axis',(0.,0.,1.));
#28080=DIRECTION('ref_axis',(1.,0.,0.));
#28081=DIRECTION('',(0.,0.,1.));
#28082=DIRECTION('center_axis',(0.,0.,1.));
#28083=DIRECTION('ref_axis',(1.,0.,0.));
#28084=DIRECTION('center_axis',(0.,0.,1.));
#28085=DIRECTION('ref_axis',(1.,0.,0.));
#28086=DIRECTION('',(-0.707106781186566,-8.65956056235516E-17,0.707106781186529));
#28087=DIRECTION('center_axis',(0.,0.,1.));
#28088=DIRECTION('ref_axis',(1.,0.,0.));
#28089=DIRECTION('center_axis',(0.,0.,-1.));
#28090=DIRECTION('ref_axis',(-1.,0.,0.));
#28091=DIRECTION('center_axis',(0.,0.,1.));
#28092=DIRECTION('ref_axis',(1.,0.,0.));
#28093=DIRECTION('center_axis',(0.,0.,1.));
#28094=DIRECTION('ref_axis',(1.,0.,0.));
#28095=DIRECTION('',(0.,0.,1.));
#28096=DIRECTION('center_axis',(0.,0.,-1.));
#28097=DIRECTION('ref_axis',(1.,0.,0.));
#28098=DIRECTION('center_axis',(0.,0.,-1.));
#28099=DIRECTION('ref_axis',(1.,0.,0.));
#28100=DIRECTION('center_axis',(0.,0.,1.));
#28101=DIRECTION('ref_axis',(1.,0.,0.));
#28102=DIRECTION('',(0.316227766016828,3.87267321454026E-17,0.948683298050517));
#28103=DIRECTION('center_axis',(0.,0.,1.));
#28104=DIRECTION('ref_axis',(1.,0.,0.));
#28105=DIRECTION('center_axis',(0.,0.,1.));
#28106=DIRECTION('ref_axis',(1.,0.,0.));
#28107=DIRECTION('',(0.,0.,1.));
#28108=DIRECTION('center_axis',(0.,0.,1.));
#28109=DIRECTION('ref_axis',(1.,0.,0.));
#28110=DIRECTION('center_axis',(0.,0.,1.));
#28111=DIRECTION('ref_axis',(1.,0.,0.));
#28112=DIRECTION('',(-0.70710678118656,-8.65956056235509E-17,0.707106781186535));
#28113=DIRECTION('center_axis',(0.,0.,1.));
#28114=DIRECTION('ref_axis',(1.,0.,0.));
#28115=DIRECTION('center_axis',(0.,0.,-1.));
#28116=DIRECTION('ref_axis',(-1.,0.,0.));
#28117=DIRECTION('center_axis',(0.,0.,1.));
#28118=DIRECTION('ref_axis',(1.,0.,0.));
#28119=DIRECTION('center_axis',(0.,0.,1.));
#28120=DIRECTION('ref_axis',(1.,0.,0.));
#28121=DIRECTION('',(0.,0.,1.));
#28122=DIRECTION('center_axis',(0.,0.,-1.));
#28123=DIRECTION('ref_axis',(1.,0.,0.));
#28124=DIRECTION('center_axis',(0.,0.,-1.));
#28125=DIRECTION('ref_axis',(1.,0.,0.));
#28126=DIRECTION('center_axis',(0.,0.,1.));
#28127=DIRECTION('ref_axis',(1.,0.,0.));
#28128=DIRECTION('',(0.316227766016838,3.87267321454039E-17,0.948683298050514));
#28129=DIRECTION('center_axis',(0.,0.,1.));
#28130=DIRECTION('ref_axis',(1.,0.,0.));
#28131=DIRECTION('center_axis',(0.,0.,1.));
#28132=DIRECTION('ref_axis',(1.,0.,0.));
#28133=DIRECTION('',(0.,0.,1.));
#28134=DIRECTION('center_axis',(0.,0.,1.));
#28135=DIRECTION('ref_axis',(1.,0.,0.));
#28136=DIRECTION('center_axis',(0.,0.,1.));
#28137=DIRECTION('ref_axis',(1.,0.,0.));
#28138=DIRECTION('',(-0.707106781186573,-8.65956056235524E-17,0.707106781186522));
#28139=DIRECTION('center_axis',(0.,0.,1.));
#28140=DIRECTION('ref_axis',(1.,0.,0.));
#28141=DIRECTION('center_axis',(0.,0.,-1.));
#28142=DIRECTION('ref_axis',(-1.,0.,0.));
#28143=DIRECTION('center_axis',(0.,0.,1.));
#28144=DIRECTION('ref_axis',(1.,0.,0.));
#28145=DIRECTION('center_axis',(0.,0.,1.));
#28146=DIRECTION('ref_axis',(1.,0.,0.));
#28147=DIRECTION('',(0.,0.,1.));
#28148=DIRECTION('center_axis',(0.,0.,-1.));
#28149=DIRECTION('ref_axis',(1.,0.,0.));
#28150=DIRECTION('center_axis',(0.,0.,-1.));
#28151=DIRECTION('ref_axis',(1.,0.,0.));
#28152=DIRECTION('center_axis',(0.,0.,1.));
#28153=DIRECTION('ref_axis',(1.,0.,0.));
#28154=DIRECTION('',(0.316227766016833,3.87267321454033E-17,0.948683298050516));
#28155=DIRECTION('center_axis',(0.,0.,1.));
#28156=DIRECTION('ref_axis',(1.,0.,0.));
#28157=DIRECTION('center_axis',(0.,0.,1.));
#28158=DIRECTION('ref_axis',(1.,0.,0.));
#28159=DIRECTION('',(0.,0.,1.));
#28160=DIRECTION('center_axis',(0.,0.,1.));
#28161=DIRECTION('ref_axis',(1.,0.,0.));
#28162=DIRECTION('center_axis',(0.,0.,1.));
#28163=DIRECTION('ref_axis',(1.,0.,0.));
#28164=DIRECTION('',(-0.707106781186566,-8.65956056235516E-17,0.707106781186529));
#28165=DIRECTION('center_axis',(0.,0.,1.));
#28166=DIRECTION('ref_axis',(1.,0.,0.));
#28167=DIRECTION('center_axis',(0.,0.,-1.));
#28168=DIRECTION('ref_axis',(-1.,0.,0.));
#28169=DIRECTION('center_axis',(0.,0.,1.));
#28170=DIRECTION('ref_axis',(1.,0.,0.));
#28171=DIRECTION('center_axis',(0.,0.,1.));
#28172=DIRECTION('ref_axis',(1.,0.,0.));
#28173=DIRECTION('',(0.,0.,1.));
#28174=DIRECTION('center_axis',(0.,0.,-1.));
#28175=DIRECTION('ref_axis',(1.,0.,0.));
#28176=DIRECTION('center_axis',(0.,0.,-1.));
#28177=DIRECTION('ref_axis',(1.,0.,0.));
#28178=DIRECTION('center_axis',(0.,0.,1.));
#28179=DIRECTION('ref_axis',(1.,0.,0.));
#28180=DIRECTION('',(0.316227766016833,3.87267321454033E-17,0.948683298050515));
#28181=DIRECTION('center_axis',(0.,0.,1.));
#28182=DIRECTION('ref_axis',(1.,0.,0.));
#28183=DIRECTION('center_axis',(0.,0.,1.));
#28184=DIRECTION('ref_axis',(1.,0.,0.));
#28185=DIRECTION('',(0.,0.,1.));
#28186=DIRECTION('center_axis',(0.,0.,1.));
#28187=DIRECTION('ref_axis',(1.,0.,0.));
#28188=DIRECTION('center_axis',(0.,0.,1.));
#28189=DIRECTION('ref_axis',(1.,0.,0.));
#28190=DIRECTION('',(-0.707106781186566,-8.65956056235516E-17,0.707106781186529));
#28191=DIRECTION('center_axis',(0.,0.,1.));
#28192=DIRECTION('ref_axis',(1.,0.,0.));
#28193=DIRECTION('center_axis',(0.,0.,-1.));
#28194=DIRECTION('ref_axis',(-1.,0.,0.));
#28195=DIRECTION('center_axis',(0.,0.,1.));
#28196=DIRECTION('ref_axis',(1.,0.,0.));
#28197=DIRECTION('center_axis',(0.,0.,1.));
#28198=DIRECTION('ref_axis',(1.,0.,0.));
#28199=DIRECTION('',(0.,0.,1.));
#28200=DIRECTION('center_axis',(0.,0.,-1.));
#28201=DIRECTION('ref_axis',(1.,0.,0.));
#28202=DIRECTION('center_axis',(0.,0.,-1.));
#28203=DIRECTION('ref_axis',(1.,0.,0.));
#28204=DIRECTION('center_axis',(0.,0.,1.));
#28205=DIRECTION('ref_axis',(1.,0.,0.));
#28206=DIRECTION('',(0.316227766016835,3.87267321454036E-17,0.948683298050515));
#28207=DIRECTION('center_axis',(0.,0.,1.));
#28208=DIRECTION('ref_axis',(1.,0.,0.));
#28209=DIRECTION('center_axis',(0.,0.,1.));
#28210=DIRECTION('ref_axis',(1.,0.,0.));
#28211=DIRECTION('',(0.,0.,1.));
#28212=DIRECTION('center_axis',(0.,0.,1.));
#28213=DIRECTION('ref_axis',(1.,0.,0.));
#28214=DIRECTION('center_axis',(0.,0.,1.));
#28215=DIRECTION('ref_axis',(1.,0.,0.));
#28216=DIRECTION('',(-0.70710678118657,-8.6595605623552E-17,0.707106781186526));
#28217=DIRECTION('center_axis',(0.,0.,1.));
#28218=DIRECTION('ref_axis',(1.,0.,0.));
#28219=DIRECTION('center_axis',(0.,0.,-1.));
#28220=DIRECTION('ref_axis',(-1.,0.,0.));
#28221=DIRECTION('center_axis',(0.,0.,1.));
#28222=DIRECTION('ref_axis',(1.,0.,0.));
#28223=DIRECTION('center_axis',(0.,0.,1.));
#28224=DIRECTION('ref_axis',(1.,0.,0.));
#28225=DIRECTION('',(0.,0.,1.));
#28226=DIRECTION('center_axis',(0.,0.,-1.));
#28227=DIRECTION('ref_axis',(1.,0.,0.));
#28228=DIRECTION('center_axis',(0.,0.,-1.));
#28229=DIRECTION('ref_axis',(1.,0.,0.));
#28230=DIRECTION('center_axis',(0.,0.,1.));
#28231=DIRECTION('ref_axis',(1.,0.,0.));
#28232=DIRECTION('',(0.316227766016833,3.87267321454033E-17,0.948683298050515));
#28233=DIRECTION('center_axis',(0.,0.,1.));
#28234=DIRECTION('ref_axis',(1.,0.,0.));
#28235=DIRECTION('center_axis',(0.,0.,1.));
#28236=DIRECTION('ref_axis',(1.,0.,0.));
#28237=DIRECTION('',(0.,0.,1.));
#28238=DIRECTION('center_axis',(0.,0.,1.));
#28239=DIRECTION('ref_axis',(1.,0.,0.));
#28240=DIRECTION('center_axis',(0.,0.,1.));
#28241=DIRECTION('ref_axis',(1.,0.,0.));
#28242=DIRECTION('',(-0.707106781186566,-8.65956056235516E-17,0.707106781186529));
#28243=DIRECTION('center_axis',(0.,0.,1.));
#28244=DIRECTION('ref_axis',(1.,0.,0.));
#28245=DIRECTION('center_axis',(0.,0.,-1.));
#28246=DIRECTION('ref_axis',(-1.,0.,0.));
#28247=DIRECTION('center_axis',(0.,0.,1.));
#28248=DIRECTION('ref_axis',(1.,0.,0.));
#28249=DIRECTION('center_axis',(0.,0.,1.));
#28250=DIRECTION('ref_axis',(1.,0.,0.));
#28251=DIRECTION('',(0.,0.,1.));
#28252=DIRECTION('center_axis',(0.,0.,-1.));
#28253=DIRECTION('ref_axis',(1.,0.,0.));
#28254=DIRECTION('center_axis',(0.,0.,-1.));
#28255=DIRECTION('ref_axis',(1.,0.,0.));
#28256=DIRECTION('center_axis',(0.,0.,1.));
#28257=DIRECTION('ref_axis',(1.,0.,0.));
#28258=DIRECTION('',(0.316227766016828,3.87267321454026E-17,0.948683298050517));
#28259=DIRECTION('center_axis',(0.,0.,1.));
#28260=DIRECTION('ref_axis',(1.,0.,0.));
#28261=DIRECTION('center_axis',(0.,0.,1.));
#28262=DIRECTION('ref_axis',(1.,0.,0.));
#28263=DIRECTION('',(0.,0.,1.));
#28264=DIRECTION('center_axis',(0.,0.,1.));
#28265=DIRECTION('ref_axis',(1.,0.,0.));
#28266=DIRECTION('center_axis',(0.,0.,1.));
#28267=DIRECTION('ref_axis',(1.,0.,0.));
#28268=DIRECTION('',(-0.70710678118656,-8.65956056235509E-17,0.707106781186535));
#28269=DIRECTION('center_axis',(0.,0.,1.));
#28270=DIRECTION('ref_axis',(1.,0.,0.));
#28271=DIRECTION('center_axis',(0.,0.,-1.));
#28272=DIRECTION('ref_axis',(-1.,0.,0.));
#28273=DIRECTION('center_axis',(0.,0.,1.));
#28274=DIRECTION('ref_axis',(1.,0.,0.));
#28275=DIRECTION('center_axis',(0.,0.,1.));
#28276=DIRECTION('ref_axis',(1.,0.,0.));
#28277=DIRECTION('',(0.,0.,1.));
#28278=DIRECTION('center_axis',(0.,0.,-1.));
#28279=DIRECTION('ref_axis',(1.,0.,0.));
#28280=DIRECTION('center_axis',(0.,0.,-1.));
#28281=DIRECTION('ref_axis',(-1.,0.,0.));
#28282=DIRECTION('center_axis',(0.,0.,-1.));
#28283=DIRECTION('ref_axis',(-1.,0.,0.));
#28284=DIRECTION('',(-0.707106781186555,8.65956056235503E-17,0.70710678118654));
#28285=DIRECTION('center_axis',(0.,0.,1.));
#28286=DIRECTION('ref_axis',(-1.,0.,0.));
#28287=DIRECTION('center_axis',(0.,0.,1.));
#28288=DIRECTION('ref_axis',(-1.,0.,0.));
#28289=DIRECTION('center_axis',(0.,0.,1.));
#28290=DIRECTION('ref_axis',(1.,0.,0.));
#28291=DIRECTION('center_axis',(0.,0.,-1.));
#28292=DIRECTION('ref_axis',(-1.,0.,0.));
#28293=DIRECTION('center_axis',(0.,0.,-1.));
#28294=DIRECTION('ref_axis',(-1.,0.,0.));
#28295=DIRECTION('',(0.,0.,-1.));
#28296=DIRECTION('center_axis',(0.,0.,-1.));
#28297=DIRECTION('ref_axis',(-1.,0.,0.));
#28298=DIRECTION('center_axis',(0.,0.,1.));
#28299=DIRECTION('ref_axis',(1.,0.,0.));
#28300=DIRECTION('center_axis',(0.,0.,1.));
#28301=DIRECTION('ref_axis',(-1.,0.,0.));
#28302=DIRECTION('',(0.707106781186555,-8.65956056235503E-17,0.70710678118654));
#28303=DIRECTION('center_axis',(0.,0.,1.));
#28304=DIRECTION('ref_axis',(-1.,0.,0.));
#28305=DIRECTION('center_axis',(0.,0.,1.));
#28306=DIRECTION('ref_axis',(1.,0.,0.));
#28307=DIRECTION('center_axis',(0.,0.,1.));
#28308=DIRECTION('ref_axis',(1.,0.,0.));
#28309=DIRECTION('center_axis',(0.,0.,1.));
#28310=DIRECTION('ref_axis',(-1.,0.,0.));
#28311=DIRECTION('center_axis',(0.,0.,-1.));
#28312=DIRECTION('ref_axis',(-1.,0.,0.));
#28313=DIRECTION('center_axis',(0.,0.,-1.));
#28314=DIRECTION('ref_axis',(-1.,0.,0.));
#28315=DIRECTION('',(-0.707106781186558,-8.65956056235506E-17,-0.707106781186537));
#28316=DIRECTION('center_axis',(0.,0.,1.));
#28317=DIRECTION('ref_axis',(-1.,0.,0.));
#28318=DIRECTION('center_axis',(0.,0.,1.));
#28319=DIRECTION('ref_axis',(1.,0.,0.));
#28320=DIRECTION('center_axis',(0.,0.,1.));
#28321=DIRECTION('ref_axis',(-1.,0.,0.));
#28322=DIRECTION('center_axis',(0.,0.,1.));
#28323=DIRECTION('ref_axis',(-1.,0.,0.));
#28324=DIRECTION('',(0.,0.,-1.));
#28325=DIRECTION('center_axis',(0.,0.,-1.));
#28326=DIRECTION('ref_axis',(-1.,0.,0.));
#28327=DIRECTION('center_axis',(0.,0.,1.));
#28328=DIRECTION('ref_axis',(1.,0.,0.));
#28329=DIRECTION('center_axis',(0.,0.,-1.));
#28330=DIRECTION('ref_axis',(-1.,0.,0.));
#28331=DIRECTION('center_axis',(0.,0.,-1.));
#28332=DIRECTION('ref_axis',(-1.,0.,0.));
#28333=DIRECTION('',(0.707106781186558,8.65956056235506E-17,-0.707106781186537));
#28334=DIRECTION('center_axis',(0.,0.,1.));
#28335=DIRECTION('ref_axis',(1.,0.,0.));
#28336=DIRECTION('',(0.5,-0.866025403784439,0.));
#28337=DIRECTION('center_axis',(0.,0.,1.));
#28338=DIRECTION('ref_axis',(0.866025403784439,-0.499999999999999,0.));
#28339=DIRECTION('',(-1.,0.,0.));
#28340=DIRECTION('center_axis',(0.,0.,1.));
#28341=DIRECTION('ref_axis',(1.,0.,0.));
#28342=DIRECTION('center_axis',(0.,0.,1.));
#28343=DIRECTION('ref_axis',(-0.425897586725943,0.904771377542978,0.));
#28344=DIRECTION('center_axis',(0.,0.,1.));
#28345=DIRECTION('ref_axis',(1.,0.,0.));
#28346=DIRECTION('',(1.,0.,0.));
#28347=DIRECTION('center_axis',(0.,0.,1.));
#28348=DIRECTION('ref_axis',(0.866025403784438,0.500000000000002,0.));
#28349=DIRECTION('',(-0.5,-0.866025403784439,0.));
#28350=DIRECTION('center_axis',(0.,0.,1.));
#28351=DIRECTION('ref_axis',(-0.425897586725943,-0.904771377542978,0.));
#28352=DIRECTION('',(0.5,0.866025403784439,0.));
#28353=DIRECTION('center_axis',(0.,0.,1.));
#28354=DIRECTION('ref_axis',(0.,1.,0.));
#28355=DIRECTION('',(0.5,-0.866025403784439,0.));
#28356=DIRECTION('center_axis',(0.,0.,1.));
#28357=DIRECTION('ref_axis',(0.570606204206288,-0.821223818286642,0.));
#28358=DIRECTION('center_axis',(0.,0.,1.));
#28359=DIRECTION('ref_axis',(1.,0.,0.));
#28360=DIRECTION('center_axis',(0.,0.,1.));
#28361=DIRECTION('ref_axis',(1.,0.,0.));
#28362=DIRECTION('center_axis',(0.,0.,1.));
#28363=DIRECTION('ref_axis',(0.570606204206288,0.821223818286642,0.));
#28364=DIRECTION('',(-0.5,-0.866025403784439,0.));
#28365=DIRECTION('center_axis',(0.,0.,1.));
#28366=DIRECTION('ref_axis',(0.,-1.,0.));
#28367=DIRECTION('',(-0.5,0.866025403784439,0.));
#28368=DIRECTION('',(1.,0.,0.));
#28369=DIRECTION('center_axis',(0.,0.,1.));
#28370=DIRECTION('ref_axis',(0.86602540378444,0.499999999999997,0.));
#28371=DIRECTION('',(-0.5,-0.866025403784439,0.));
#28372=DIRECTION('center_axis',(0.,0.,1.));
#28373=DIRECTION('ref_axis',(1.,0.,0.));
#28374=DIRECTION('center_axis',(0.,0.,1.));
#28375=DIRECTION('ref_axis',(-0.996503790932232,0.0835475592563362,0.));
#28376=DIRECTION('center_axis',(0.,0.,1.));
#28377=DIRECTION('ref_axis',(1.,0.,0.));
#28378=DIRECTION('',(0.5,-0.866025403784439,0.));
#28379=DIRECTION('center_axis',(0.,0.,1.));
#28380=DIRECTION('ref_axis',(0.866025403784437,-0.500000000000003,0.));
#28381=DIRECTION('',(-1.,0.,0.));
#28382=DIRECTION('center_axis',(0.,0.,1.));
#28383=DIRECTION('ref_axis',(-0.996503790932232,-0.0835475592563325,0.));
#28384=DIRECTION('',(-0.5,0.866025403784439,0.));
#28385=DIRECTION('center_axis',(0.,0.,1.));
#28386=DIRECTION('ref_axis',(-0.866025403784437,0.500000000000003,0.));
#28387=DIRECTION('',(1.,0.,0.));
#28388=DIRECTION('center_axis',(0.,0.,1.));
#28389=DIRECTION('ref_axis',(0.996503790932232,0.0835475592563325,0.));
#28390=DIRECTION('center_axis',(0.,0.,1.));
#28391=DIRECTION('ref_axis',(1.,0.,0.));
#28392=DIRECTION('center_axis',(0.,0.,1.));
#28393=DIRECTION('ref_axis',(1.,0.,0.));
#28394=DIRECTION('center_axis',(0.,0.,1.));
#28395=DIRECTION('ref_axis',(0.996503790932232,-0.0835475592563362,0.));
#28396=DIRECTION('',(-1.,0.,0.));
#28397=DIRECTION('center_axis',(0.,0.,1.));
#28398=DIRECTION('ref_axis',(-0.86602540378444,-0.499999999999997,0.));
#28399=DIRECTION('',(0.5,0.866025403784439,0.));
#28400=DIRECTION('',(0.5,0.866025403784439,0.));
#28401=DIRECTION('center_axis',(0.,0.,1.));
#28402=DIRECTION('ref_axis',(0.,1.,0.));
#28403=DIRECTION('',(0.5,-0.866025403784439,0.));
#28404=DIRECTION('center_axis',(0.,0.,1.));
#28405=DIRECTION('ref_axis',(1.,0.,0.));
#28406=DIRECTION('center_axis',(0.,0.,1.));
#28407=DIRECTION('ref_axis',(-0.570606204206288,-0.821223818286642,0.));
#28408=DIRECTION('center_axis',(0.,0.,1.));
#28409=DIRECTION('ref_axis',(1.,0.,0.));
#28410=DIRECTION('',(-0.5,-0.866025403784439,0.));
#28411=DIRECTION('center_axis',(0.,0.,1.));
#28412=DIRECTION('ref_axis',(0.,-1.,0.));
#28413=DIRECTION('',(-0.5,0.866025403784439,0.));
#28414=DIRECTION('center_axis',(0.,0.,1.));
#28415=DIRECTION('ref_axis',(-0.570606204206288,0.821223818286642,0.));
#28416=DIRECTION('',(-1.,0.,0.));
#28417=DIRECTION('center_axis',(0.,0.,1.));
#28418=DIRECTION('ref_axis',(-0.866025403784438,-0.500000000000002,0.));
#28419=DIRECTION('',(0.5,0.866025403784439,0.));
#28420=DIRECTION('center_axis',(0.,0.,1.));
#28421=DIRECTION('ref_axis',(0.425897586725943,0.904771377542978,0.));
#28422=DIRECTION('center_axis',(0.,0.,1.));
#28423=DIRECTION('ref_axis',(1.,0.,0.));
#28424=DIRECTION('center_axis',(0.,0.,1.));
#28425=DIRECTION('ref_axis',(1.,0.,0.));
#28426=DIRECTION('center_axis',(0.,0.,1.));
#28427=DIRECTION('ref_axis',(0.425897586725943,-0.904771377542978,0.));
#28428=DIRECTION('',(-0.5,0.866025403784439,0.));
#28429=DIRECTION('center_axis',(0.,0.,1.));
#28430=DIRECTION('ref_axis',(-0.866025403784439,0.499999999999999,0.));
#28431=DIRECTION('',(1.,0.,0.));
#28432=DIRECTION('',(-1.,0.,0.));
#28433=DIRECTION('center_axis',(0.,0.,1.));
#28434=DIRECTION('ref_axis',(-0.866025403784441,-0.499999999999996,0.));
#28435=DIRECTION('',(0.5,0.866025403784439,0.));
#28436=DIRECTION('center_axis',(0.,0.,1.));
#28437=DIRECTION('ref_axis',(0.,1.,0.));
#28438=DIRECTION('',(0.5,-0.866025403784439,0.));
#28439=DIRECTION('center_axis',(0.,0.,1.));
#28440=DIRECTION('ref_axis',(0.86602540378444,-0.499999999999997,0.));
#28441=DIRECTION('',(-1.,0.,0.));
#28442=DIRECTION('center_axis',(0.,0.,1.));
#28443=DIRECTION('ref_axis',(-0.86602540378444,-0.499999999999997,0.));
#28444=DIRECTION('',(0.5,0.866025403784439,0.));
#28445=DIRECTION('center_axis',(0.,0.,1.));
#28446=DIRECTION('ref_axis',(3.70074341541719E-15,1.,0.));
#28447=DIRECTION('',(0.5,-0.866025403784439,0.));
#28448=DIRECTION('center_axis',(0.,0.,1.));
#28449=DIRECTION('ref_axis',(0.866025403784439,-0.499999999999999,0.));
#28450=DIRECTION('',(-1.,0.,0.));
#28451=DIRECTION('center_axis',(0.,0.,1.));
#28452=DIRECTION('ref_axis',(-0.86602540378444,-0.499999999999998,0.));
#28453=DIRECTION('',(0.5,0.866025403784439,0.));
#28454=DIRECTION('center_axis',(0.,0.,1.));
#28455=DIRECTION('ref_axis',(-1.85037170770859E-15,1.,0.));
#28456=DIRECTION('',(0.5,-0.866025403784439,0.));
#28457=DIRECTION('center_axis',(0.,0.,1.));
#28458=DIRECTION('ref_axis',(0.86602540378444,-0.499999999999997,0.));
#28459=DIRECTION('',(-0.5,-0.866025403784439,0.));
#28460=DIRECTION('center_axis',(0.,0.,1.));
#28461=DIRECTION('ref_axis',(0.,-1.,0.));
#28462=DIRECTION('',(-0.5,0.866025403784439,0.));
#28463=DIRECTION('center_axis',(0.,0.,1.));
#28464=DIRECTION('ref_axis',(-0.86602540378444,0.499999999999997,0.));
#28465=DIRECTION('',(1.,0.,0.));
#28466=DIRECTION('center_axis',(0.,0.,1.));
#28467=DIRECTION('ref_axis',(0.866025403784439,0.499999999999999,0.));
#28468=DIRECTION('',(-1.,0.,0.));
#28469=DIRECTION('center_axis',(0.,0.,1.));
#28470=DIRECTION('ref_axis',(-0.86602540378444,-0.499999999999997,0.));
#28471=DIRECTION('',(0.5,0.866025403784439,0.));
#28472=DIRECTION('center_axis',(0.,0.,1.));
#28473=DIRECTION('ref_axis',(0.,1.,0.));
#28474=DIRECTION('',(0.5,-0.866025403784439,0.));
#28475=DIRECTION('center_axis',(0.,0.,1.));
#28476=DIRECTION('ref_axis',(0.86602540378444,-0.499999999999997,0.));
#28477=DIRECTION('',(-0.5,-0.866025403784439,0.));
#28478=DIRECTION('center_axis',(0.,0.,1.));
#28479=DIRECTION('ref_axis',(0.,-1.,0.));
#28480=DIRECTION('',(-0.5,0.866025403784439,0.));
#28481=DIRECTION('center_axis',(0.,0.,1.));
#28482=DIRECTION('ref_axis',(-0.86602540378444,0.499999999999997,0.));
#28483=DIRECTION('',(1.,0.,0.));
#28484=DIRECTION('center_axis',(0.,0.,1.));
#28485=DIRECTION('ref_axis',(0.86602540378444,0.499999999999997,0.));
#28486=DIRECTION('',(-1.,0.,0.));
#28487=DIRECTION('center_axis',(0.,0.,1.));
#28488=DIRECTION('ref_axis',(-0.866025403784439,-0.499999999999999,0.));
#28489=DIRECTION('',(0.5,0.866025403784439,0.));
#28490=DIRECTION('center_axis',(0.,0.,1.));
#28491=DIRECTION('ref_axis',(0.,1.,0.));
#28492=DIRECTION('',(0.5,-0.866025403784439,0.));
#28493=DIRECTION('center_axis',(0.,0.,1.));
#28494=DIRECTION('ref_axis',(0.86602540378444,-0.499999999999997,0.));
#28495=DIRECTION('',(-0.5,-0.866025403784439,0.));
#28496=DIRECTION('center_axis',(0.,0.,1.));
#28497=DIRECTION('ref_axis',(1.85037170770859E-15,-1.,0.));
#28498=DIRECTION('',(-0.5,0.866025403784439,0.));
#28499=DIRECTION('center_axis',(0.,0.,1.));
#28500=DIRECTION('ref_axis',(-0.86602540378444,0.499999999999997,0.));
#28501=DIRECTION('',(1.,0.,0.));
#28502=DIRECTION('center_axis',(0.,0.,1.));
#28503=DIRECTION('ref_axis',(0.86602540378444,0.499999999999998,0.));
#28504=DIRECTION('',(-0.5,-0.866025403784439,0.));
#28505=DIRECTION('center_axis',(0.,0.,1.));
#28506=DIRECTION('ref_axis',(-3.70074341541719E-15,-1.,0.));
#28507=DIRECTION('',(-0.5,0.866025403784439,0.));
#28508=DIRECTION('center_axis',(0.,0.,1.));
#28509=DIRECTION('ref_axis',(-0.866025403784439,0.499999999999999,0.));
#28510=DIRECTION('',(1.,0.,0.));
#28511=DIRECTION('center_axis',(0.,0.,1.));
#28512=DIRECTION('ref_axis',(0.86602540378444,0.499999999999997,0.));
#28513=DIRECTION('',(-0.5,-0.866025403784439,0.));
#28514=DIRECTION('center_axis',(0.,0.,1.));
#28515=DIRECTION('ref_axis',(0.,-1.,0.));
#28516=DIRECTION('',(-0.5,0.866025403784439,0.));
#28517=DIRECTION('center_axis',(0.,0.,1.));
#28518=DIRECTION('ref_axis',(-0.86602540378444,0.499999999999997,0.));
#28519=DIRECTION('',(1.,0.,0.));
#28520=DIRECTION('center_axis',(0.,0.,1.));
#28521=DIRECTION('ref_axis',(0.866025403784441,0.499999999999996,0.));
#28522=DIRECTION('',(-1.,0.,0.));
#28523=DIRECTION('center_axis',(0.,0.,1.));
#28524=DIRECTION('ref_axis',(-0.866025403784441,-0.499999999999996,0.));
#28525=DIRECTION('',(0.5,0.866025403784439,0.));
#28526=DIRECTION('center_axis',(0.,0.,1.));
#28527=DIRECTION('ref_axis',(0.,1.,0.));
#28528=DIRECTION('',(0.5,-0.866025403784439,0.));
#28529=DIRECTION('center_axis',(0.,0.,1.));
#28530=DIRECTION('ref_axis',(0.86602540378444,-0.499999999999997,0.));
#28531=DIRECTION('',(-1.,0.,0.));
#28532=DIRECTION('center_axis',(0.,0.,1.));
#28533=DIRECTION('ref_axis',(-0.866025403784439,-0.499999999999999,0.));
#28534=DIRECTION('',(0.5,0.866025403784439,0.));
#28535=DIRECTION('center_axis',(0.,0.,1.));
#28536=DIRECTION('ref_axis',(0.,1.,0.));
#28537=DIRECTION('',(0.5,-0.866025403784439,0.));
#28538=DIRECTION('center_axis',(0.,0.,1.));
#28539=DIRECTION('ref_axis',(0.866025403784439,-0.5,0.));
#28540=DIRECTION('',(-0.5,-0.866025403784439,0.));
#28541=DIRECTION('center_axis',(0.,0.,1.));
#28542=DIRECTION('ref_axis',(0.,-1.,0.));
#28543=DIRECTION('',(-0.5,0.866025403784439,0.));
#28544=DIRECTION('center_axis',(0.,0.,1.));
#28545=DIRECTION('ref_axis',(-0.866025403784438,0.500000000000002,0.));
#28546=DIRECTION('',(1.,0.,0.));
#28547=DIRECTION('center_axis',(0.,0.,1.));
#28548=DIRECTION('ref_axis',(0.866025403784439,0.5,0.));
#28549=DIRECTION('',(-1.,0.,0.));
#28550=DIRECTION('center_axis',(0.,0.,1.));
#28551=DIRECTION('ref_axis',(-0.86602540378444,-0.499999999999997,0.));
#28552=DIRECTION('',(0.5,0.866025403784439,0.));
#28553=DIRECTION('center_axis',(0.,0.,1.));
#28554=DIRECTION('ref_axis',(-6.93889390390722E-16,1.,0.));
#28555=DIRECTION('',(0.5,-0.866025403784439,0.));
#28556=DIRECTION('center_axis',(0.,0.,1.));
#28557=DIRECTION('ref_axis',(0.866025403784439,-0.5,0.));
#28558=DIRECTION('',(-0.5,-0.866025403784439,0.));
#28559=DIRECTION('center_axis',(0.,0.,1.));
#28560=DIRECTION('ref_axis',(6.93889390390722E-16,-1.,0.));
#28561=DIRECTION('',(-0.5,0.866025403784439,0.));
#28562=DIRECTION('center_axis',(0.,0.,1.));
#28563=DIRECTION('ref_axis',(-0.866025403784439,0.5,0.));
#28564=DIRECTION('',(1.,0.,0.));
#28565=DIRECTION('center_axis',(0.,0.,1.));
#28566=DIRECTION('ref_axis',(0.86602540378444,0.499999999999997,0.));
#28567=DIRECTION('',(-1.,0.,0.));
#28568=DIRECTION('center_axis',(0.,0.,1.));
#28569=DIRECTION('ref_axis',(-0.866025403784439,-0.5,0.));
#28570=DIRECTION('',(0.5,0.866025403784439,0.));
#28571=DIRECTION('center_axis',(0.,0.,1.));
#28572=DIRECTION('ref_axis',(0.,1.,0.));
#28573=DIRECTION('',(0.5,-0.866025403784439,0.));
#28574=DIRECTION('center_axis',(0.,0.,1.));
#28575=DIRECTION('ref_axis',(0.866025403784438,-0.500000000000002,0.));
#28576=DIRECTION('',(-0.5,-0.866025403784439,0.));
#28577=DIRECTION('center_axis',(0.,0.,1.));
#28578=DIRECTION('ref_axis',(0.,-1.,0.));
#28579=DIRECTION('',(-0.5,0.866025403784439,0.));
#28580=DIRECTION('center_axis',(0.,0.,1.));
#28581=DIRECTION('ref_axis',(-0.866025403784439,0.5,0.));
#28582=DIRECTION('',(1.,0.,0.));
#28583=DIRECTION('center_axis',(0.,0.,1.));
#28584=DIRECTION('ref_axis',(0.866025403784439,0.499999999999999,0.));
#28585=DIRECTION('',(-0.5,-0.866025403784439,0.));
#28586=DIRECTION('center_axis',(0.,0.,1.));
#28587=DIRECTION('ref_axis',(0.,-1.,0.));
#28588=DIRECTION('',(-0.5,0.866025403784439,0.));
#28589=DIRECTION('center_axis',(0.,0.,1.));
#28590=DIRECTION('ref_axis',(-0.86602540378444,0.499999999999997,0.));
#28591=DIRECTION('',(1.,0.,0.));
#28592=DIRECTION('center_axis',(0.,0.,1.));
#28593=DIRECTION('ref_axis',(0.866025403784441,0.499999999999996,0.));
#28594=DIRECTION('center_axis',(0.,0.,1.));
#28595=DIRECTION('ref_axis',(1.,0.,0.));
#28596=DIRECTION('center_axis',(0.,0.,1.));
#28597=DIRECTION('ref_axis',(0.425897586725943,0.904771377542978,0.));
#28598=DIRECTION('',(0.,0.,-1.));
#28599=DIRECTION('center_axis',(0.,0.,1.));
#28600=DIRECTION('ref_axis',(0.425897586725943,0.904771377542978,0.));
#28601=DIRECTION('',(0.,0.,1.));
#28602=DIRECTION('center_axis',(0.,0.,-1.));
#28603=DIRECTION('ref_axis',(-0.866025403784439,0.499999999999999,0.));
#28604=DIRECTION('center_axis',(0.,0.,1.));
#28605=DIRECTION('ref_axis',(-0.866025403784439,0.499999999999999,0.));
#28606=DIRECTION('',(0.,0.,1.));
#28607=DIRECTION('',(0.,0.,-1.));
#28608=DIRECTION('center_axis',(0.,1.,0.));
#28609=DIRECTION('ref_axis',(1.,0.,0.));
#28610=DIRECTION('',(1.,0.,0.));
#28611=DIRECTION('',(0.,0.,1.));
#28612=DIRECTION('center_axis',(0.,0.,-1.));
#28613=DIRECTION('ref_axis',(0.425897586725943,-0.904771377542978,0.));
#28614=DIRECTION('center_axis',(0.,0.,1.));
#28615=DIRECTION('ref_axis',(0.425897586725943,-0.904771377542978,0.));
#28616=DIRECTION('',(0.,0.,1.));
#28617=DIRECTION('',(0.,0.,-1.));
#28618=DIRECTION('center_axis',(0.,0.,-1.));
#28619=DIRECTION('ref_axis',(-1.,0.,0.));
#28620=DIRECTION('',(-0.5,0.866025403784439,0.));
#28621=DIRECTION('center_axis',(0.,0.,1.));
#28622=DIRECTION('ref_axis',(1.,0.,0.));
#28623=DIRECTION('center_axis',(0.,0.,-1.));
#28624=DIRECTION('ref_axis',(-0.86602540378444,0.499999999999997,0.));
#28625=DIRECTION('center_axis',(0.,0.,1.));
#28626=DIRECTION('ref_axis',(-0.86602540378444,0.499999999999997,0.));
#28627=DIRECTION('',(0.,0.,1.));
#28628=DIRECTION('',(0.,0.,-1.));
#28629=DIRECTION('center_axis',(0.,1.,0.));
#28630=DIRECTION('ref_axis',(1.,0.,0.));
#28631=DIRECTION('',(1.,0.,0.));
#28632=DIRECTION('',(0.,0.,-1.));
#28633=DIRECTION('center_axis',(0.,0.,-1.));
#28634=DIRECTION('ref_axis',(0.,-1.,0.));
#28635=DIRECTION('center_axis',(0.,0.,1.));
#28636=DIRECTION('ref_axis',(0.,-1.,0.));
#28637=DIRECTION('',(0.,0.,1.));
#28638=DIRECTION('',(0.,0.,-1.));
#28639=DIRECTION('center_axis',(0.,0.,-1.));
#28640=DIRECTION('ref_axis',(-1.,0.,0.));
#28641=DIRECTION('',(-0.5,0.866025403784439,0.));
#28642=DIRECTION('',(-0.5,-0.866025403784439,0.));
#28643=DIRECTION('center_axis',(0.,0.,1.));
#28644=DIRECTION('ref_axis',(0.866025403784441,0.499999999999996,0.));
#28645=DIRECTION('center_axis',(0.866025403784439,-0.5,0.));
#28646=DIRECTION('ref_axis',(-0.5,-0.866025403784439,0.));
#28647=DIRECTION('',(0.,0.,1.));
#28648=DIRECTION('center_axis',(0.,0.,-1.));
#28649=DIRECTION('ref_axis',(0.866025403784441,0.499999999999996,0.));
#28650=DIRECTION('center_axis',(0.,0.,-1.));
#28651=DIRECTION('ref_axis',(-0.866025403784439,0.5,0.));
#28652=DIRECTION('center_axis',(0.,0.,1.));
#28653=DIRECTION('ref_axis',(-0.866025403784439,0.5,0.));
#28654=DIRECTION('',(0.,0.,1.));
#28655=DIRECTION('',(0.,0.,-1.));
#28656=DIRECTION('center_axis',(0.,1.,0.));
#28657=DIRECTION('ref_axis',(1.,0.,0.));
#28658=DIRECTION('',(1.,0.,0.));
#28659=DIRECTION('',(0.,0.,-1.));
#28660=DIRECTION('center_axis',(0.,0.,-1.));
#28661=DIRECTION('ref_axis',(0.,-1.,0.));
#28662=DIRECTION('center_axis',(0.,0.,1.));
#28663=DIRECTION('ref_axis',(0.,-1.,0.));
#28664=DIRECTION('',(0.,0.,1.));
#28665=DIRECTION('',(0.,0.,-1.));
#28666=DIRECTION('center_axis',(0.,0.,-1.));
#28667=DIRECTION('ref_axis',(-1.,0.,0.));
#28668=DIRECTION('',(-0.5,0.866025403784439,0.));
#28669=DIRECTION('',(-0.5,-0.866025403784439,0.));
#28670=DIRECTION('center_axis',(0.,0.,1.));
#28671=DIRECTION('ref_axis',(0.866025403784439,0.499999999999999,0.));
#28672=DIRECTION('center_axis',(0.866025403784439,-0.5,0.));
#28673=DIRECTION('ref_axis',(-0.5,-0.866025403784439,0.));
#28674=DIRECTION('',(0.,0.,1.));
#28675=DIRECTION('center_axis',(0.,0.,-1.));
#28676=DIRECTION('ref_axis',(0.866025403784439,0.499999999999999,0.));
#28677=DIRECTION('center_axis',(0.,0.,1.));
#28678=DIRECTION('ref_axis',(0.996503790932232,0.0835475592563325,0.));
#28679=DIRECTION('',(0.,0.,-1.));
#28680=DIRECTION('center_axis',(0.,0.,1.));
#28681=DIRECTION('ref_axis',(0.996503790932232,0.0835475592563325,0.));
#28682=DIRECTION('',(0.,0.,1.));
#28683=DIRECTION('center_axis',(0.,0.,-1.));
#28684=DIRECTION('ref_axis',(0.,1.,0.));
#28685=DIRECTION('center_axis',(0.,0.,1.));
#28686=DIRECTION('ref_axis',(0.,1.,0.));
#28687=DIRECTION('',(0.,0.,1.));
#28688=DIRECTION('',(0.,0.,-1.));
#28689=DIRECTION('center_axis',(0.866025403784439,0.5,0.));
#28690=DIRECTION('ref_axis',(0.5,-0.866025403784439,0.));
#28691=DIRECTION('',(0.5,-0.866025403784439,0.));
#28692=DIRECTION('',(0.,0.,-1.));
#28693=DIRECTION('center_axis',(0.,0.,-1.));
#28694=DIRECTION('ref_axis',(-0.866025403784439,-0.5,0.));
#28695=DIRECTION('center_axis',(0.,0.,1.));
#28696=DIRECTION('ref_axis',(-0.866025403784439,-0.5,0.));
#28697=DIRECTION('',(0.,0.,1.));
#28698=DIRECTION('',(0.,0.,-1.));
#28699=DIRECTION('center_axis',(0.,0.,-1.));
#28700=DIRECTION('ref_axis',(-1.,0.,0.));
#28701=DIRECTION('',(0.5,0.866025403784439,0.));
#28702=DIRECTION('',(-1.,0.,0.));
#28703=DIRECTION('center_axis',(0.,0.,1.));
#28704=DIRECTION('ref_axis',(0.866025403784438,-0.500000000000002,0.));
#28705=DIRECTION('center_axis',(0.,-1.,0.));
#28706=DIRECTION('ref_axis',(-1.,0.,0.));
#28707=DIRECTION('',(0.,0.,1.));
#28708=DIRECTION('center_axis',(0.,0.,-1.));
#28709=DIRECTION('ref_axis',(0.866025403784438,-0.500000000000002,0.));
#28710=DIRECTION('center_axis',(0.,0.,-1.));
#28711=DIRECTION('ref_axis',(-0.866025403784439,0.5,0.));
#28712=DIRECTION('center_axis',(0.,0.,1.));
#28713=DIRECTION('ref_axis',(-0.866025403784439,0.5,0.));
#28714=DIRECTION('',(0.,0.,1.));
#28715=DIRECTION('',(0.,0.,-1.));
#28716=DIRECTION('center_axis',(0.,1.,0.));
#28717=DIRECTION('ref_axis',(1.,0.,0.));
#28718=DIRECTION('',(1.,0.,0.));
#28719=DIRECTION('',(0.,0.,-1.));
#28720=DIRECTION('center_axis',(0.,0.,-1.));
#28721=DIRECTION('ref_axis',(6.93889390390722E-16,-1.,0.));
#28722=DIRECTION('center_axis',(0.,0.,1.));
#28723=DIRECTION('ref_axis',(6.93889390390722E-16,-1.,0.));
#28724=DIRECTION('',(0.,0.,1.));
#28725=DIRECTION('',(0.,0.,-1.));
#28726=DIRECTION('center_axis',(0.,0.,-1.));
#28727=DIRECTION('ref_axis',(-1.,0.,0.));
#28728=DIRECTION('',(-0.5,0.866025403784439,0.));
#28729=DIRECTION('',(-0.5,-0.866025403784439,0.));
#28730=DIRECTION('center_axis',(0.,0.,1.));
#28731=DIRECTION('ref_axis',(0.86602540378444,0.499999999999997,0.));
#28732=DIRECTION('center_axis',(0.866025403784439,-0.5,0.));
#28733=DIRECTION('ref_axis',(-0.5,-0.866025403784439,0.));
#28734=DIRECTION('',(0.,0.,1.));
#28735=DIRECTION('center_axis',(0.,0.,-1.));
#28736=DIRECTION('ref_axis',(0.86602540378444,0.499999999999997,0.));
#28737=DIRECTION('center_axis',(0.,0.,-1.));
#28738=DIRECTION('ref_axis',(0.86602540378444,0.499999999999997,0.));
#28739=DIRECTION('center_axis',(0.,0.,1.));
#28740=DIRECTION('ref_axis',(0.86602540378444,0.499999999999997,0.));
#28741=DIRECTION('',(0.,0.,1.));
#28742=DIRECTION('',(0.,0.,-1.));
#28743=DIRECTION('center_axis',(0.866025403784439,-0.5,0.));
#28744=DIRECTION('ref_axis',(-0.5,-0.866025403784439,0.));
#28745=DIRECTION('',(-0.5,-0.866025403784439,0.));
#28746=DIRECTION('',(0.,0.,1.));
#28747=DIRECTION('center_axis',(0.,0.,-1.));
#28748=DIRECTION('ref_axis',(-0.86602540378444,-0.499999999999997,0.));
#28749=DIRECTION('center_axis',(0.,0.,1.));
#28750=DIRECTION('ref_axis',(-0.86602540378444,-0.499999999999997,0.));
#28751=DIRECTION('',(0.,0.,1.));
#28752=DIRECTION('',(0.,0.,-1.));
#28753=DIRECTION('center_axis',(0.,0.,-1.));
#28754=DIRECTION('ref_axis',(-1.,0.,0.));
#28755=DIRECTION('',(-1.,0.,0.));
#28756=DIRECTION('center_axis',(0.,0.,1.));
#28757=DIRECTION('ref_axis',(0.996503790932232,-0.0835475592563362,0.));
#28758=DIRECTION('center_axis',(0.,0.,1.));
#28759=DIRECTION('ref_axis',(1.,0.,0.));
#28760=DIRECTION('',(0.5,0.866025403784439,0.));
#28761=DIRECTION('center_axis',(0.,-1.,0.));
#28762=DIRECTION('ref_axis',(-1.,0.,0.));
#28763=DIRECTION('',(0.,0.,1.));
#28764=DIRECTION('center_axis',(0.,0.,-1.));
#28765=DIRECTION('ref_axis',(0.996503790932232,-0.0835475592563362,0.));
#28766=DIRECTION('',(0.,0.,-1.));
#28767=DIRECTION('center_axis',(0.,0.,-1.));
#28768=DIRECTION('ref_axis',(-6.93889390390722E-16,1.,0.));
#28769=DIRECTION('center_axis',(0.,0.,1.));
#28770=DIRECTION('ref_axis',(-6.93889390390722E-16,1.,0.));
#28771=DIRECTION('',(0.,0.,1.));
#28772=DIRECTION('',(0.,0.,-1.));
#28773=DIRECTION('center_axis',(0.866025403784439,0.5,0.));
#28774=DIRECTION('ref_axis',(0.5,-0.866025403784439,0.));
#28775=DIRECTION('',(0.5,-0.866025403784439,0.));
#28776=DIRECTION('',(0.,0.,-1.));
#28777=DIRECTION('center_axis',(0.,0.,-1.));
#28778=DIRECTION('ref_axis',(-0.86602540378444,-0.499999999999997,0.));
#28779=DIRECTION('center_axis',(0.,0.,1.));
#28780=DIRECTION('ref_axis',(-0.86602540378444,-0.499999999999997,0.));
#28781=DIRECTION('',(0.,0.,1.));
#28782=DIRECTION('',(0.,0.,-1.));
#28783=DIRECTION('center_axis',(0.,0.,-1.));
#28784=DIRECTION('ref_axis',(-1.,0.,0.));
#28785=DIRECTION('',(0.5,0.866025403784439,0.));
#28786=DIRECTION('',(-1.,0.,0.));
#28787=DIRECTION('center_axis',(0.,0.,1.));
#28788=DIRECTION('ref_axis',(0.866025403784439,-0.5,0.));
#28789=DIRECTION('center_axis',(0.,-1.,0.));
#28790=DIRECTION('ref_axis',(-1.,0.,0.));
#28791=DIRECTION('',(0.,0.,1.));
#28792=DIRECTION('center_axis',(0.,0.,-1.));
#28793=DIRECTION('ref_axis',(0.866025403784439,-0.5,0.));
#28794=DIRECTION('center_axis',(0.,0.,-1.));
#28795=DIRECTION('ref_axis',(-0.866025403784438,0.500000000000002,0.));
#28796=DIRECTION('center_axis',(0.,0.,1.));
#28797=DIRECTION('ref_axis',(-0.866025403784438,0.500000000000002,0.));
#28798=DIRECTION('',(0.,0.,1.));
#28799=DIRECTION('',(0.,0.,-1.));
#28800=DIRECTION('center_axis',(0.,1.,0.));
#28801=DIRECTION('ref_axis',(1.,0.,0.));
#28802=DIRECTION('',(1.,0.,0.));
#28803=DIRECTION('',(0.,0.,-1.));
#28804=DIRECTION('center_axis',(0.,0.,-1.));
#28805=DIRECTION('ref_axis',(0.,-1.,0.));
#28806=DIRECTION('center_axis',(0.,0.,1.));
#28807=DIRECTION('ref_axis',(0.,-1.,0.));
#28808=DIRECTION('',(0.,0.,1.));
#28809=DIRECTION('',(0.,0.,-1.));
#28810=DIRECTION('center_axis',(0.,0.,-1.));
#28811=DIRECTION('ref_axis',(-1.,0.,0.));
#28812=DIRECTION('',(-0.5,0.866025403784439,0.));
#28813=DIRECTION('',(-0.5,-0.866025403784439,0.));
#28814=DIRECTION('center_axis',(0.,0.,1.));
#28815=DIRECTION('ref_axis',(0.866025403784439,0.5,0.));
#28816=DIRECTION('center_axis',(0.866025403784439,-0.5,0.));
#28817=DIRECTION('ref_axis',(-0.5,-0.866025403784439,0.));
#28818=DIRECTION('',(0.,0.,1.));
#28819=DIRECTION('center_axis',(0.,0.,-1.));
#28820=DIRECTION('ref_axis',(0.866025403784439,0.5,0.));
#28821=DIRECTION('center_axis',(0.,0.,1.));
#28822=DIRECTION('ref_axis',(-0.996503790932232,-0.0835475592563325,0.));
#28823=DIRECTION('',(0.,0.,-1.));
#28824=DIRECTION('center_axis',(0.,0.,1.));
#28825=DIRECTION('ref_axis',(-0.996503790932232,-0.0835475592563325,0.));
#28826=DIRECTION('',(0.,0.,1.));
#28827=DIRECTION('center_axis',(0.,0.,-1.));
#28828=DIRECTION('ref_axis',(-1.,0.,0.));
#28829=DIRECTION('',(-1.,0.,0.));
#28830=DIRECTION('center_axis',(0.,0.,1.));
#28831=DIRECTION('ref_axis',(0.866025403784437,-0.500000000000003,0.));
#28832=DIRECTION('',(0.5,-0.866025403784439,0.));
#28833=DIRECTION('center_axis',(0.,0.,1.));
#28834=DIRECTION('ref_axis',(1.,0.,0.));
#28835=DIRECTION('center_axis',(0.,-1.,0.));
#28836=DIRECTION('ref_axis',(-1.,0.,0.));
#28837=DIRECTION('',(0.,0.,1.));
#28838=DIRECTION('center_axis',(0.,0.,-1.));
#28839=DIRECTION('ref_axis',(0.866025403784437,-0.500000000000003,0.));
#28840=DIRECTION('',(0.,0.,-1.));
#28841=DIRECTION('center_axis',(0.866025403784439,0.5,0.));
#28842=DIRECTION('ref_axis',(0.5,-0.866025403784439,0.));
#28843=DIRECTION('',(0.,0.,-1.));
#28844=DIRECTION('center_axis',(0.,0.,-1.));
#28845=DIRECTION('ref_axis',(0.,1.,0.));
#28846=DIRECTION('center_axis',(0.,0.,1.));
#28847=DIRECTION('ref_axis',(0.,1.,0.));
#28848=DIRECTION('',(0.,0.,1.));
#28849=DIRECTION('',(0.,0.,-1.));
#28850=DIRECTION('center_axis',(0.866025403784439,0.5,0.));
#28851=DIRECTION('ref_axis',(0.5,-0.866025403784439,0.));
#28852=DIRECTION('',(0.5,-0.866025403784439,0.));
#28853=DIRECTION('',(0.,0.,-1.));
#28854=DIRECTION('center_axis',(0.,0.,-1.));
#28855=DIRECTION('ref_axis',(-0.866025403784439,-0.499999999999999,0.));
#28856=DIRECTION('center_axis',(0.,0.,1.));
#28857=DIRECTION('ref_axis',(-0.866025403784439,-0.499999999999999,0.));
#28858=DIRECTION('',(0.,0.,1.));
#28859=DIRECTION('',(0.,0.,-1.));
#28860=DIRECTION('center_axis',(0.,0.,-1.));
#28861=DIRECTION('ref_axis',(-1.,0.,0.));
#28862=DIRECTION('',(0.5,0.866025403784439,0.));
#28863=DIRECTION('',(-1.,0.,0.));
#28864=DIRECTION('center_axis',(0.,0.,1.));
#28865=DIRECTION('ref_axis',(0.866025403784439,-0.5,0.));
#28866=DIRECTION('center_axis',(0.,-1.,0.));
#28867=DIRECTION('ref_axis',(-1.,0.,0.));
#28868=DIRECTION('',(0.,0.,1.));
#28869=DIRECTION('center_axis',(0.,0.,-1.));
#28870=DIRECTION('ref_axis',(0.866025403784439,-0.5,0.));
#28871=DIRECTION('center_axis',(0.,0.,-1.));
#28872=DIRECTION('ref_axis',(0.,1.,0.));
#28873=DIRECTION('center_axis',(0.,0.,1.));
#28874=DIRECTION('ref_axis',(0.,1.,0.));
#28875=DIRECTION('',(0.,0.,1.));
#28876=DIRECTION('',(0.,0.,-1.));
#28877=DIRECTION('center_axis',(0.866025403784439,0.5,0.));
#28878=DIRECTION('ref_axis',(0.5,-0.866025403784439,0.));
#28879=DIRECTION('',(0.5,-0.866025403784439,0.));
#28880=DIRECTION('',(0.,0.,-1.));
#28881=DIRECTION('center_axis',(0.,0.,-1.));
#28882=DIRECTION('ref_axis',(-0.866025403784441,-0.499999999999996,0.));
#28883=DIRECTION('center_axis',(0.,0.,1.));
#28884=DIRECTION('ref_axis',(-0.866025403784441,-0.499999999999996,0.));
#28885=DIRECTION('',(0.,0.,1.));
#28886=DIRECTION('',(0.,0.,-1.));
#28887=DIRECTION('center_axis',(0.,0.,-1.));
#28888=DIRECTION('ref_axis',(-1.,0.,0.));
#28889=DIRECTION('',(0.5,0.866025403784439,0.));
#28890=DIRECTION('',(-1.,0.,0.));
#28891=DIRECTION('center_axis',(0.,0.,1.));
#28892=DIRECTION('ref_axis',(0.86602540378444,-0.499999999999997,0.));
#28893=DIRECTION('center_axis',(0.,-1.,0.));
#28894=DIRECTION('ref_axis',(-1.,0.,0.));
#28895=DIRECTION('',(0.,0.,1.));
#28896=DIRECTION('center_axis',(0.,0.,-1.));
#28897=DIRECTION('ref_axis',(0.86602540378444,-0.499999999999997,0.));
#28898=DIRECTION('center_axis',(0.,0.,-1.));
#28899=DIRECTION('ref_axis',(0.866025403784439,-0.499999999999999,0.));
#28900=DIRECTION('center_axis',(0.,0.,1.));
#28901=DIRECTION('ref_axis',(0.866025403784439,-0.499999999999999,0.));
#28902=DIRECTION('',(0.,0.,1.));
#28903=DIRECTION('',(0.,0.,-1.));
#28904=DIRECTION('center_axis',(0.,-1.,0.));
#28905=DIRECTION('ref_axis',(-1.,0.,0.));
#28906=DIRECTION('',(-1.,0.,0.));
#28907=DIRECTION('',(0.,0.,1.));
#28908=DIRECTION('center_axis',(0.,0.,-1.));
#28909=DIRECTION('ref_axis',(0.,-1.,0.));
#28910=DIRECTION('center_axis',(0.,0.,1.));
#28911=DIRECTION('ref_axis',(0.,-1.,0.));
#28912=DIRECTION('',(0.,0.,1.));
#28913=DIRECTION('',(0.,0.,-1.));
#28914=DIRECTION('center_axis',(0.,0.,-1.));
#28915=DIRECTION('ref_axis',(-1.,0.,0.));
#28916=DIRECTION('',(-0.5,-0.866025403784439,0.));
#28917=DIRECTION('center_axis',(0.,0.,1.));
#28918=DIRECTION('ref_axis',(0.570606204206288,0.821223818286642,0.));
#28919=DIRECTION('center_axis',(0.,0.,1.));
#28920=DIRECTION('ref_axis',(1.,0.,0.));
#28921=DIRECTION('',(-0.5,0.866025403784439,0.));
#28922=DIRECTION('center_axis',(0.866025403784439,-0.5,0.));
#28923=DIRECTION('ref_axis',(-0.5,-0.866025403784439,0.));
#28924=DIRECTION('',(0.,0.,1.));
#28925=DIRECTION('center_axis',(0.,0.,-1.));
#28926=DIRECTION('ref_axis',(0.570606204206288,0.821223818286642,0.));
#28927=DIRECTION('',(0.,0.,-1.));
#28928=DIRECTION('center_axis',(0.,0.,-1.));
#28929=DIRECTION('ref_axis',(-0.86602540378444,0.499999999999997,0.));
#28930=DIRECTION('center_axis',(0.,0.,1.));
#28931=DIRECTION('ref_axis',(-0.86602540378444,0.499999999999997,0.));
#28932=DIRECTION('',(0.,0.,1.));
#28933=DIRECTION('',(0.,0.,-1.));
#28934=DIRECTION('center_axis',(0.,1.,0.));
#28935=DIRECTION('ref_axis',(1.,0.,0.));
#28936=DIRECTION('',(1.,0.,0.));
#28937=DIRECTION('',(0.,0.,-1.));
#28938=DIRECTION('center_axis',(0.,0.,-1.));
#28939=DIRECTION('ref_axis',(0.,-1.,0.));
#28940=DIRECTION('center_axis',(0.,0.,1.));
#28941=DIRECTION('ref_axis',(0.,-1.,0.));
#28942=DIRECTION('',(0.,0.,1.));
#28943=DIRECTION('',(0.,0.,-1.));
#28944=DIRECTION('center_axis',(0.,0.,-1.));
#28945=DIRECTION('ref_axis',(-1.,0.,0.));
#28946=DIRECTION('',(-0.5,0.866025403784439,0.));
#28947=DIRECTION('',(-0.5,-0.866025403784439,0.));
#28948=DIRECTION('center_axis',(0.,0.,1.));
#28949=DIRECTION('ref_axis',(0.866025403784441,0.499999999999996,0.));
#28950=DIRECTION('center_axis',(0.866025403784439,-0.5,0.));
#28951=DIRECTION('ref_axis',(-0.5,-0.866025403784439,0.));
#28952=DIRECTION('',(0.,0.,1.));
#28953=DIRECTION('center_axis',(0.,0.,-1.));
#28954=DIRECTION('ref_axis',(0.866025403784441,0.499999999999996,0.));
#28955=DIRECTION('center_axis',(0.,0.,-1.));
#28956=DIRECTION('ref_axis',(-0.866025403784439,0.499999999999999,0.));
#28957=DIRECTION('center_axis',(0.,0.,1.));
#28958=DIRECTION('ref_axis',(-0.866025403784439,0.499999999999999,0.));
#28959=DIRECTION('',(0.,0.,1.));
#28960=DIRECTION('',(0.,0.,-1.));
#28961=DIRECTION('center_axis',(0.,1.,0.));
#28962=DIRECTION('ref_axis',(1.,0.,0.));
#28963=DIRECTION('',(1.,0.,0.));
#28964=DIRECTION('',(0.,0.,-1.));
#28965=DIRECTION('center_axis',(0.,0.,-1.));
#28966=DIRECTION('ref_axis',(-3.70074341541719E-15,-1.,0.));
#28967=DIRECTION('center_axis',(0.,0.,1.));
#28968=DIRECTION('ref_axis',(-3.70074341541719E-15,-1.,0.));
#28969=DIRECTION('',(0.,0.,1.));
#28970=DIRECTION('',(0.,0.,-1.));
#28971=DIRECTION('center_axis',(0.,0.,-1.));
#28972=DIRECTION('ref_axis',(-1.,0.,0.));
#28973=DIRECTION('',(-0.5,0.866025403784439,0.));
#28974=DIRECTION('',(-0.5,-0.866025403784439,0.));
#28975=DIRECTION('center_axis',(0.,0.,1.));
#28976=DIRECTION('ref_axis',(0.86602540378444,0.499999999999997,0.));
#28977=DIRECTION('center_axis',(0.866025403784439,-0.5,0.));
#28978=DIRECTION('ref_axis',(-0.5,-0.866025403784439,0.));
#28979=DIRECTION('',(0.,0.,1.));
#28980=DIRECTION('center_axis',(0.,0.,-1.));
#28981=DIRECTION('ref_axis',(0.86602540378444,0.499999999999997,0.));
#28982=DIRECTION('center_axis',(0.,0.,-1.));
#28983=DIRECTION('ref_axis',(-0.86602540378444,0.499999999999997,0.));
#28984=DIRECTION('center_axis',(0.,0.,1.));
#28985=DIRECTION('ref_axis',(-0.86602540378444,0.499999999999997,0.));
#28986=DIRECTION('',(0.,0.,1.));
#28987=DIRECTION('',(0.,0.,-1.));
#28988=DIRECTION('center_axis',(0.,1.,0.));
#28989=DIRECTION('ref_axis',(1.,0.,0.));
#28990=DIRECTION('',(1.,0.,0.));
#28991=DIRECTION('',(0.,0.,-1.));
#28992=DIRECTION('center_axis',(0.,0.,-1.));
#28993=DIRECTION('ref_axis',(1.85037170770859E-15,-1.,0.));
#28994=DIRECTION('center_axis',(0.,0.,1.));
#28995=DIRECTION('ref_axis',(1.85037170770859E-15,-1.,0.));
#28996=DIRECTION('',(0.,0.,1.));
#28997=DIRECTION('',(0.,0.,-1.));
#28998=DIRECTION('center_axis',(0.,0.,-1.));
#28999=DIRECTION('ref_axis',(-1.,0.,0.));
#29000=DIRECTION('',(-0.5,0.866025403784439,0.));
#29001=DIRECTION('',(-0.5,-0.866025403784439,0.));
#29002=DIRECTION('center_axis',(0.,0.,1.));
#29003=DIRECTION('ref_axis',(0.86602540378444,0.499999999999998,0.));
#29004=DIRECTION('center_axis',(0.866025403784439,-0.5,0.));
#29005=DIRECTION('ref_axis',(-0.5,-0.866025403784439,0.));
#29006=DIRECTION('',(0.,0.,1.));
#29007=DIRECTION('center_axis',(0.,0.,-1.));
#29008=DIRECTION('ref_axis',(0.86602540378444,0.499999999999998,0.));
#29009=DIRECTION('center_axis',(0.,0.,1.));
#29010=DIRECTION('ref_axis',(0.570606204206288,-0.821223818286642,0.));
#29011=DIRECTION('',(0.,0.,-1.));
#29012=DIRECTION('center_axis',(0.,0.,1.));
#29013=DIRECTION('ref_axis',(0.570606204206288,-0.821223818286642,0.));
#29014=DIRECTION('',(0.,0.,1.));
#29015=DIRECTION('center_axis',(0.,0.,-1.));
#29016=DIRECTION('ref_axis',(0.,1.,0.));
#29017=DIRECTION('center_axis',(0.,0.,1.));
#29018=DIRECTION('ref_axis',(0.,1.,0.));
#29019=DIRECTION('',(0.,0.,1.));
#29020=DIRECTION('',(0.,0.,-1.));
#29021=DIRECTION('center_axis',(0.866025403784439,0.5,0.));
#29022=DIRECTION('ref_axis',(0.5,-0.866025403784439,0.));
#29023=DIRECTION('',(0.5,-0.866025403784439,0.));
#29024=DIRECTION('',(0.,0.,-1.));
#29025=DIRECTION('center_axis',(0.,0.,-1.));
#29026=DIRECTION('ref_axis',(-0.866025403784439,-0.499999999999999,0.));
#29027=DIRECTION('center_axis',(0.,0.,1.));
#29028=DIRECTION('ref_axis',(-0.866025403784439,-0.499999999999999,0.));
#29029=DIRECTION('',(0.,0.,1.));
#29030=DIRECTION('',(0.,0.,-1.));
#29031=DIRECTION('center_axis',(0.,0.,-1.));
#29032=DIRECTION('ref_axis',(-1.,0.,0.));
#29033=DIRECTION('',(0.5,0.866025403784439,0.));
#29034=DIRECTION('',(-1.,0.,0.));
#29035=DIRECTION('center_axis',(0.,0.,1.));
#29036=DIRECTION('ref_axis',(0.86602540378444,-0.499999999999997,0.));
#29037=DIRECTION('center_axis',(0.,-1.,0.));
#29038=DIRECTION('ref_axis',(-1.,0.,0.));
#29039=DIRECTION('',(0.,0.,1.));
#29040=DIRECTION('center_axis',(0.,0.,-1.));
#29041=DIRECTION('ref_axis',(0.86602540378444,-0.499999999999997,0.));
#29042=DIRECTION('center_axis',(0.,0.,-1.));
#29043=DIRECTION('ref_axis',(-0.86602540378444,0.499999999999997,0.));
#29044=DIRECTION('center_axis',(0.,0.,1.));
#29045=DIRECTION('ref_axis',(-0.86602540378444,0.499999999999997,0.));
#29046=DIRECTION('',(0.,0.,1.));
#29047=DIRECTION('',(0.,0.,-1.));
#29048=DIRECTION('center_axis',(0.,1.,0.));
#29049=DIRECTION('ref_axis',(1.,0.,0.));
#29050=DIRECTION('',(1.,0.,0.));
#29051=DIRECTION('',(0.,0.,-1.));
#29052=DIRECTION('center_axis',(0.,0.,-1.));
#29053=DIRECTION('ref_axis',(0.,-1.,0.));
#29054=DIRECTION('center_axis',(0.,0.,1.));
#29055=DIRECTION('ref_axis',(0.,-1.,0.));
#29056=DIRECTION('',(0.,0.,1.));
#29057=DIRECTION('',(0.,0.,-1.));
#29058=DIRECTION('center_axis',(0.,0.,-1.));
#29059=DIRECTION('ref_axis',(-1.,0.,0.));
#29060=DIRECTION('',(-0.5,0.866025403784439,0.));
#29061=DIRECTION('',(-0.5,-0.866025403784439,0.));
#29062=DIRECTION('center_axis',(0.,0.,1.));
#29063=DIRECTION('ref_axis',(0.86602540378444,0.499999999999997,0.));
#29064=DIRECTION('center_axis',(0.866025403784439,-0.5,0.));
#29065=DIRECTION('ref_axis',(-0.5,-0.866025403784439,0.));
#29066=DIRECTION('',(0.,0.,1.));
#29067=DIRECTION('center_axis',(0.,0.,-1.));
#29068=DIRECTION('ref_axis',(0.86602540378444,0.499999999999997,0.));
#29069=DIRECTION('center_axis',(0.,0.,1.));
#29070=DIRECTION('ref_axis',(-0.425897586725943,-0.904771377542978,0.));
#29071=DIRECTION('',(0.,0.,-1.));
#29072=DIRECTION('center_axis',(0.,0.,1.));
#29073=DIRECTION('ref_axis',(-0.425897586725943,-0.904771377542978,0.));
#29074=DIRECTION('',(0.,0.,1.));
#29075=DIRECTION('center_axis',(0.,0.,-1.));
#29076=DIRECTION('ref_axis',(-1.,0.,0.));
#29077=DIRECTION('',(-0.5,-0.866025403784439,0.));
#29078=DIRECTION('center_axis',(0.,0.,1.));
#29079=DIRECTION('ref_axis',(0.866025403784438,0.500000000000002,0.));
#29080=DIRECTION('',(1.,0.,0.));
#29081=DIRECTION('center_axis',(0.,0.,1.));
#29082=DIRECTION('ref_axis',(1.,0.,0.));
#29083=DIRECTION('center_axis',(0.866025403784439,-0.5,0.));
#29084=DIRECTION('ref_axis',(-0.5,-0.866025403784439,0.));
#29085=DIRECTION('',(0.,0.,1.));
#29086=DIRECTION('center_axis',(0.,0.,-1.));
#29087=DIRECTION('ref_axis',(0.866025403784438,0.500000000000002,0.));
#29088=DIRECTION('',(0.,0.,-1.));
#29089=DIRECTION('center_axis',(0.,1.,0.));
#29090=DIRECTION('ref_axis',(1.,0.,0.));
#29091=DIRECTION('',(0.,0.,-1.));
#29092=DIRECTION('center_axis',(0.,0.,-1.));
#29093=DIRECTION('ref_axis',(0.,1.,0.));
#29094=DIRECTION('center_axis',(0.,0.,1.));
#29095=DIRECTION('ref_axis',(0.,1.,0.));
#29096=DIRECTION('',(0.,0.,1.));
#29097=DIRECTION('',(0.,0.,-1.));
#29098=DIRECTION('center_axis',(0.866025403784439,0.5,0.));
#29099=DIRECTION('ref_axis',(0.5,-0.866025403784439,0.));
#29100=DIRECTION('',(0.5,-0.866025403784439,0.));
#29101=DIRECTION('',(0.,0.,-1.));
#29102=DIRECTION('center_axis',(0.,0.,-1.));
#29103=DIRECTION('ref_axis',(-0.86602540378444,-0.499999999999997,0.));
#29104=DIRECTION('center_axis',(0.,0.,1.));
#29105=DIRECTION('ref_axis',(-0.86602540378444,-0.499999999999997,0.));
#29106=DIRECTION('',(0.,0.,1.));
#29107=DIRECTION('',(0.,0.,-1.));
#29108=DIRECTION('center_axis',(0.,0.,-1.));
#29109=DIRECTION('ref_axis',(-1.,0.,0.));
#29110=DIRECTION('',(0.5,0.866025403784439,0.));
#29111=DIRECTION('',(-1.,0.,0.));
#29112=DIRECTION('center_axis',(0.,0.,1.));
#29113=DIRECTION('ref_axis',(0.86602540378444,-0.499999999999997,0.));
#29114=DIRECTION('center_axis',(0.,-1.,0.));
#29115=DIRECTION('ref_axis',(-1.,0.,0.));
#29116=DIRECTION('',(0.,0.,1.));
#29117=DIRECTION('center_axis',(0.,0.,-1.));
#29118=DIRECTION('ref_axis',(0.86602540378444,-0.499999999999997,0.));
#29119=DIRECTION('center_axis',(0.,0.,-1.));
#29120=DIRECTION('ref_axis',(-0.86602540378444,0.499999999999997,0.));
#29121=DIRECTION('center_axis',(0.,0.,1.));
#29122=DIRECTION('ref_axis',(-0.86602540378444,0.499999999999997,0.));
#29123=DIRECTION('',(0.,0.,1.));
#29124=DIRECTION('',(0.,0.,-1.));
#29125=DIRECTION('center_axis',(0.,1.,0.));
#29126=DIRECTION('ref_axis',(1.,0.,0.));
#29127=DIRECTION('',(1.,0.,0.));
#29128=DIRECTION('',(0.,0.,-1.));
#29129=DIRECTION('center_axis',(0.,0.,-1.));
#29130=DIRECTION('ref_axis',(0.,-1.,0.));
#29131=DIRECTION('center_axis',(0.,0.,1.));
#29132=DIRECTION('ref_axis',(0.,-1.,0.));
#29133=DIRECTION('',(0.,0.,1.));
#29134=DIRECTION('',(0.,0.,-1.));
#29135=DIRECTION('center_axis',(0.,0.,-1.));
#29136=DIRECTION('ref_axis',(-1.,0.,0.));
#29137=DIRECTION('',(-0.5,0.866025403784439,0.));
#29138=DIRECTION('',(-0.5,-0.866025403784439,0.));
#29139=DIRECTION('center_axis',(0.,0.,1.));
#29140=DIRECTION('ref_axis',(0.866025403784439,0.499999999999999,0.));
#29141=DIRECTION('center_axis',(0.866025403784439,-0.5,0.));
#29142=DIRECTION('ref_axis',(-0.5,-0.866025403784439,0.));
#29143=DIRECTION('',(0.,0.,1.));
#29144=DIRECTION('center_axis',(0.,0.,-1.));
#29145=DIRECTION('ref_axis',(0.866025403784439,0.499999999999999,0.));
#29146=DIRECTION('center_axis',(0.,0.,1.));
#29147=DIRECTION('ref_axis',(-0.570606204206288,0.821223818286642,0.));
#29148=DIRECTION('',(0.,0.,-1.));
#29149=DIRECTION('center_axis',(0.,0.,1.));
#29150=DIRECTION('ref_axis',(-0.570606204206288,0.821223818286642,0.));
#29151=DIRECTION('',(0.,0.,1.));
#29152=DIRECTION('center_axis',(0.,0.,-1.));
#29153=DIRECTION('ref_axis',(0.,-1.,0.));
#29154=DIRECTION('center_axis',(0.,0.,1.));
#29155=DIRECTION('ref_axis',(0.,-1.,0.));
#29156=DIRECTION('',(0.,0.,1.));
#29157=DIRECTION('',(0.,0.,-1.));
#29158=DIRECTION('center_axis',(0.,0.,-1.));
#29159=DIRECTION('ref_axis',(-1.,0.,0.));
#29160=DIRECTION('',(-0.5,0.866025403784439,0.));
#29161=DIRECTION('',(-0.5,-0.866025403784439,0.));
#29162=DIRECTION('center_axis',(0.,0.,1.));
#29163=DIRECTION('ref_axis',(1.,0.,0.));
#29164=DIRECTION('center_axis',(0.866025403784439,-0.5,0.));
#29165=DIRECTION('ref_axis',(-0.5,-0.866025403784439,0.));
#29166=DIRECTION('',(0.,0.,-1.));
#29167=DIRECTION('center_axis',(0.,0.,-1.));
#29168=DIRECTION('ref_axis',(-1.85037170770859E-15,1.,0.));
#29169=DIRECTION('center_axis',(0.,0.,1.));
#29170=DIRECTION('ref_axis',(-1.85037170770859E-15,1.,0.));
#29171=DIRECTION('',(0.,0.,1.));
#29172=DIRECTION('',(0.,0.,-1.));
#29173=DIRECTION('center_axis',(0.866025403784439,0.5,0.));
#29174=DIRECTION('ref_axis',(0.5,-0.866025403784439,0.));
#29175=DIRECTION('',(0.5,-0.866025403784439,0.));
#29176=DIRECTION('',(0.,0.,-1.));
#29177=DIRECTION('center_axis',(0.,0.,-1.));
#29178=DIRECTION('ref_axis',(-0.86602540378444,-0.499999999999998,0.));
#29179=DIRECTION('center_axis',(0.,0.,1.));
#29180=DIRECTION('ref_axis',(-0.86602540378444,-0.499999999999998,0.));
#29181=DIRECTION('',(0.,0.,1.));
#29182=DIRECTION('',(0.,0.,-1.));
#29183=DIRECTION('center_axis',(0.,0.,-1.));
#29184=DIRECTION('ref_axis',(-1.,0.,0.));
#29185=DIRECTION('',(0.5,0.866025403784439,0.));
#29186=DIRECTION('',(-1.,0.,0.));
#29187=DIRECTION('center_axis',(0.,0.,1.));
#29188=DIRECTION('ref_axis',(0.86602540378444,-0.499999999999997,0.));
#29189=DIRECTION('center_axis',(0.,-1.,0.));
#29190=DIRECTION('ref_axis',(-1.,0.,0.));
#29191=DIRECTION('',(0.,0.,1.));
#29192=DIRECTION('center_axis',(0.,0.,-1.));
#29193=DIRECTION('ref_axis',(0.86602540378444,-0.499999999999997,0.));
#29194=DIRECTION('center_axis',(0.,0.,-1.));
#29195=DIRECTION('ref_axis',(3.70074341541719E-15,1.,0.));
#29196=DIRECTION('center_axis',(0.,0.,1.));
#29197=DIRECTION('ref_axis',(3.70074341541719E-15,1.,0.));
#29198=DIRECTION('',(0.,0.,1.));
#29199=DIRECTION('',(0.,0.,-1.));
#29200=DIRECTION('center_axis',(0.866025403784439,0.5,0.));
#29201=DIRECTION('ref_axis',(0.5,-0.866025403784439,0.));
#29202=DIRECTION('',(0.5,-0.866025403784439,0.));
#29203=DIRECTION('',(0.,0.,-1.));
#29204=DIRECTION('center_axis',(0.,0.,-1.));
#29205=DIRECTION('ref_axis',(-0.86602540378444,-0.499999999999997,0.));
#29206=DIRECTION('center_axis',(0.,0.,1.));
#29207=DIRECTION('ref_axis',(-0.86602540378444,-0.499999999999997,0.));
#29208=DIRECTION('',(0.,0.,1.));
#29209=DIRECTION('',(0.,0.,-1.));
#29210=DIRECTION('center_axis',(0.,0.,-1.));
#29211=DIRECTION('ref_axis',(-1.,0.,0.));
#29212=DIRECTION('',(0.5,0.866025403784439,0.));
#29213=DIRECTION('',(-1.,0.,0.));
#29214=DIRECTION('center_axis',(0.,0.,1.));
#29215=DIRECTION('ref_axis',(0.866025403784439,-0.499999999999999,0.));
#29216=DIRECTION('center_axis',(0.,-1.,0.));
#29217=DIRECTION('ref_axis',(-1.,0.,0.));
#29218=DIRECTION('',(0.,0.,1.));
#29219=DIRECTION('center_axis',(0.,0.,-1.));
#29220=DIRECTION('ref_axis',(0.866025403784439,-0.499999999999999,0.));
#29221=DIRECTION('center_axis',(0.,0.,-1.));
#29222=DIRECTION('ref_axis',(0.,1.,0.));
#29223=DIRECTION('center_axis',(0.,0.,1.));
#29224=DIRECTION('ref_axis',(0.,1.,0.));
#29225=DIRECTION('',(0.,0.,1.));
#29226=DIRECTION('',(0.,0.,-1.));
#29227=DIRECTION('center_axis',(0.866025403784439,0.5,0.));
#29228=DIRECTION('ref_axis',(0.5,-0.866025403784439,0.));
#29229=DIRECTION('',(0.5,-0.866025403784439,0.));
#29230=DIRECTION('',(0.,0.,-1.));
#29231=DIRECTION('center_axis',(0.,0.,-1.));
#29232=DIRECTION('ref_axis',(-0.866025403784441,-0.499999999999996,0.));
#29233=DIRECTION('center_axis',(0.,0.,1.));
#29234=DIRECTION('ref_axis',(-0.866025403784441,-0.499999999999996,0.));
#29235=DIRECTION('',(0.,0.,1.));
#29236=DIRECTION('',(0.,0.,-1.));
#29237=DIRECTION('center_axis',(0.,0.,-1.));
#29238=DIRECTION('ref_axis',(-1.,0.,0.));
#29239=DIRECTION('',(0.5,0.866025403784439,0.));
#29240=DIRECTION('',(-1.,0.,0.));
#29241=DIRECTION('center_axis',(0.,0.,1.));
#29242=DIRECTION('ref_axis',(0.86602540378444,-0.499999999999997,0.));
#29243=DIRECTION('center_axis',(0.,-1.,0.));
#29244=DIRECTION('ref_axis',(-1.,0.,0.));
#29245=DIRECTION('',(0.,0.,1.));
#29246=DIRECTION('center_axis',(0.,0.,-1.));
#29247=DIRECTION('ref_axis',(0.86602540378444,-0.499999999999997,0.));
#29248=DIRECTION('center_axis',(0.,0.,-1.));
#29249=DIRECTION('ref_axis',(-0.866025403784438,-0.500000000000002,0.));
#29250=DIRECTION('center_axis',(0.,0.,1.));
#29251=DIRECTION('ref_axis',(-0.866025403784438,-0.500000000000002,0.));
#29252=DIRECTION('',(0.,0.,1.));
#29253=DIRECTION('',(0.,0.,-1.));
#29254=DIRECTION('center_axis',(0.,0.,-1.));
#29255=DIRECTION('ref_axis',(-1.,0.,0.));
#29256=DIRECTION('',(0.5,0.866025403784439,0.));
#29257=DIRECTION('',(-1.,0.,0.));
#29258=DIRECTION('center_axis',(0.,0.,1.));
#29259=DIRECTION('ref_axis',(1.,0.,0.));
#29260=DIRECTION('center_axis',(0.,-1.,0.));
#29261=DIRECTION('ref_axis',(-1.,0.,0.));
#29262=DIRECTION('',(0.,0.,-1.));
#29263=DIRECTION('center_axis',(0.,0.,-1.));
#29264=DIRECTION('ref_axis',(0.,1.,0.));
#29265=DIRECTION('center_axis',(0.,0.,1.));
#29266=DIRECTION('ref_axis',(0.,1.,0.));
#29267=DIRECTION('',(0.,0.,1.));
#29268=DIRECTION('',(0.,0.,-1.));
#29269=DIRECTION('center_axis',(0.866025403784439,0.5,0.));
#29270=DIRECTION('ref_axis',(0.5,-0.866025403784439,0.));
#29271=DIRECTION('',(0.5,-0.866025403784439,0.));
#29272=DIRECTION('',(0.,0.,1.));
#29273=DIRECTION('center_axis',(0.,0.,-1.));
#29274=DIRECTION('ref_axis',(-0.570606204206288,-0.821223818286642,0.));
#29275=DIRECTION('center_axis',(0.,0.,1.));
#29276=DIRECTION('ref_axis',(-0.570606204206288,-0.821223818286642,0.));
#29277=DIRECTION('',(0.,0.,1.));
#29278=DIRECTION('',(0.,0.,-1.));
#29279=DIRECTION('center_axis',(0.,0.,-1.));
#29280=DIRECTION('ref_axis',(-1.,0.,0.));
#29281=DIRECTION('',(0.5,0.866025403784439,0.));
#29282=DIRECTION('center_axis',(0.,0.,1.));
#29283=DIRECTION('ref_axis',(1.,0.,0.));
#29284=DIRECTION('center_axis',(0.,0.,-1.));
#29285=DIRECTION('ref_axis',(-0.866025403784437,0.500000000000003,0.));
#29286=DIRECTION('center_axis',(0.,0.,1.));
#29287=DIRECTION('ref_axis',(-0.866025403784437,0.500000000000003,0.));
#29288=DIRECTION('',(0.,0.,1.));
#29289=DIRECTION('',(0.,0.,-1.));
#29290=DIRECTION('center_axis',(0.,0.,-1.));
#29291=DIRECTION('ref_axis',(-1.,0.,0.));
#29292=DIRECTION('',(1.,0.,0.));
#29293=DIRECTION('',(-0.5,0.866025403784439,0.));
#29294=DIRECTION('center_axis',(0.,0.,1.));
#29295=DIRECTION('ref_axis',(1.,0.,0.));
#29296=DIRECTION('center_axis',(-0.866025403784439,-0.5,0.));
#29297=DIRECTION('ref_axis',(-0.5,0.866025403784439,0.));
#29298=DIRECTION('',(0.,0.,-1.));
#29299=DIRECTION('center_axis',(0.,0.,-1.));
#29300=DIRECTION('ref_axis',(-0.996503790932232,0.0835475592563362,0.));
#29301=DIRECTION('center_axis',(0.,0.,1.));
#29302=DIRECTION('ref_axis',(-0.996503790932232,0.0835475592563362,0.));
#29303=DIRECTION('',(0.,0.,1.));
#29304=DIRECTION('',(0.,0.,-1.));
#29305=DIRECTION('center_axis',(0.,0.,-1.));
#29306=DIRECTION('ref_axis',(-1.,0.,0.));
#29307=DIRECTION('',(1.,0.,0.));
#29308=DIRECTION('center_axis',(0.,0.,1.));
#29309=DIRECTION('ref_axis',(1.,0.,0.));
#29310=DIRECTION('center_axis',(0.,0.,-1.));
#29311=DIRECTION('ref_axis',(0.,1.,0.));
#29312=DIRECTION('center_axis',(0.,0.,1.));
#29313=DIRECTION('ref_axis',(0.,1.,0.));
#29314=DIRECTION('',(0.,0.,1.));
#29315=DIRECTION('',(0.,0.,-1.));
#29316=DIRECTION('center_axis',(0.,0.,-1.));
#29317=DIRECTION('ref_axis',(-1.,0.,0.));
#29318=DIRECTION('',(0.5,-0.866025403784439,0.));
#29319=DIRECTION('',(0.5,0.866025403784439,0.));
#29320=DIRECTION('center_axis',(0.,0.,1.));
#29321=DIRECTION('ref_axis',(1.,0.,0.));
#29322=DIRECTION('center_axis',(-0.866025403784439,0.5,0.));
#29323=DIRECTION('ref_axis',(0.5,0.866025403784439,0.));
#29324=DIRECTION('',(0.,0.,-1.));
#29325=DIRECTION('center_axis',(0.,0.,-1.));
#29326=DIRECTION('ref_axis',(-0.425897586725943,0.904771377542978,0.));
#29327=DIRECTION('center_axis',(0.,0.,1.));
#29328=DIRECTION('ref_axis',(-0.425897586725943,0.904771377542978,0.));
#29329=DIRECTION('',(0.,0.,1.));
#29330=DIRECTION('',(0.,0.,-1.));
#29331=DIRECTION('center_axis',(0.,0.,-1.));
#29332=DIRECTION('ref_axis',(-1.,0.,0.));
#29333=DIRECTION('',(0.5,-0.866025403784439,0.));
#29334=DIRECTION('center_axis',(0.,0.,1.));
#29335=DIRECTION('ref_axis',(1.,0.,0.));
#29336=DIRECTION('center_axis',(0.,0.,1.));
#29337=DIRECTION('ref_axis',(1.,0.,0.));
#29338=DIRECTION('center_axis',(0.,0.,1.));
#29339=DIRECTION('ref_axis',(1.,0.,0.));
#29340=DIRECTION('center_axis',(0.,0.,1.));
#29341=DIRECTION('ref_axis',(1.,0.,0.));
#29342=DIRECTION('center_axis',(0.,0.,1.));
#29343=DIRECTION('ref_axis',(1.,0.,0.));
#29344=DIRECTION('center_axis',(0.,0.,1.));
#29345=DIRECTION('ref_axis',(1.,0.,0.));
#29346=DIRECTION('center_axis',(0.,0.,1.));
#29347=DIRECTION('ref_axis',(1.,0.,0.));
#29348=DIRECTION('',(0.,0.,1.));
#29349=DIRECTION('center_axis',(0.,0.,1.));
#29350=DIRECTION('ref_axis',(1.,0.,0.));
#29351=DIRECTION('center_axis',(0.,0.,1.));
#29352=DIRECTION('ref_axis',(1.,0.,0.));
#29353=DIRECTION('center_axis',(0.,0.,1.));
#29354=DIRECTION('ref_axis',(1.,0.,0.));
#29355=DIRECTION('center_axis',(0.,0.,1.));
#29356=DIRECTION('ref_axis',(1.,0.,0.));
#29357=DIRECTION('',(0.,0.,1.));
#29358=DIRECTION('center_axis',(0.,0.,1.));
#29359=DIRECTION('ref_axis',(1.,0.,0.));
#29360=DIRECTION('center_axis',(0.,0.,1.));
#29361=DIRECTION('ref_axis',(1.,0.,0.));
#29362=DIRECTION('center_axis',(-0.866025403784439,0.5,0.));
#29363=DIRECTION('ref_axis',(0.5,0.866025403784439,0.));
#29364=DIRECTION('center_axis',(-0.866025403784439,0.5,0.));
#29365=DIRECTION('ref_axis',(0.5,0.866025403784439,0.));
#29366=DIRECTION('center_axis',(-0.866025403784439,0.5,0.));
#29367=DIRECTION('ref_axis',(0.5,0.866025403784439,0.));
#29368=DIRECTION('center_axis',(-0.866025403784439,0.5,0.));
#29369=DIRECTION('ref_axis',(0.5,0.866025403784439,0.));
#29370=DIRECTION('center_axis',(-0.866025403784439,-0.5,0.));
#29371=DIRECTION('ref_axis',(-0.5,0.866025403784439,0.));
#29372=DIRECTION('center_axis',(-0.866025403784439,-0.5,0.));
#29373=DIRECTION('ref_axis',(-0.5,0.866025403784439,0.));
#29374=DIRECTION('center_axis',(-0.866025403784439,0.5,0.));
#29375=DIRECTION('ref_axis',(0.5,0.866025403784439,0.));
#29376=DIRECTION('center_axis',(-0.866025403784439,-0.5,0.));
#29377=DIRECTION('ref_axis',(-0.5,0.866025403784439,0.));
#29378=DIRECTION('center_axis',(-0.866025403784439,0.5,0.));
#29379=DIRECTION('ref_axis',(0.5,0.866025403784439,0.));
#29380=DIRECTION('center_axis',(0.866025403784439,0.5,0.));
#29381=DIRECTION('ref_axis',(0.5,-0.866025403784439,0.));
#29382=DIRECTION('center_axis',(-0.866025403784439,-0.5,0.));
#29383=DIRECTION('ref_axis',(-0.5,0.866025403784439,0.));
#29384=DIRECTION('center_axis',(-0.866025403784439,-0.5,0.));
#29385=DIRECTION('ref_axis',(-0.5,0.866025403784439,0.));
#29386=DIRECTION('center_axis',(-0.866025403784439,-0.5,0.));
#29387=DIRECTION('ref_axis',(-0.5,0.866025403784439,0.));
#29388=DIRECTION('center_axis',(-0.866025403784439,-0.5,0.));
#29389=DIRECTION('ref_axis',(-0.5,0.866025403784439,0.));
#29390=DIRECTION('center_axis',(0.866025403784439,0.5,0.));
#29391=DIRECTION('ref_axis',(0.5,-0.866025403784439,0.));
#29392=DIRECTION('center_axis',(-0.866025403784439,0.5,0.));
#29393=DIRECTION('ref_axis',(0.5,0.866025403784439,0.));
#29394=DIRECTION('center_axis',(-0.866025403784439,0.5,0.));
#29395=DIRECTION('ref_axis',(0.5,0.866025403784439,0.));
#29396=DIRECTION('center_axis',(-0.866025403784439,-0.5,0.));
#29397=DIRECTION('ref_axis',(-0.5,0.866025403784439,0.));
#29398=DIRECTION('center_axis',(-0.866025403784439,0.5,0.));
#29399=DIRECTION('ref_axis',(0.5,0.866025403784439,0.));
#29400=DIRECTION('center_axis',(-0.866025403784439,0.5,0.));
#29401=DIRECTION('ref_axis',(0.5,0.866025403784439,0.));
#29402=DIRECTION('center_axis',(0.,1.,0.));
#29403=DIRECTION('ref_axis',(1.,0.,0.));
#29404=DIRECTION('center_axis',(-0.866025403784439,-0.5,0.));
#29405=DIRECTION('ref_axis',(-0.5,0.866025403784439,0.));
#29406=DIRECTION('center_axis',(-0.866025403784439,0.5,0.));
#29407=DIRECTION('ref_axis',(0.5,0.866025403784439,0.));
#29408=DIRECTION('center_axis',(0.,1.,0.));
#29409=DIRECTION('ref_axis',(1.,0.,0.));
#29410=DIRECTION('center_axis',(-0.866025403784439,-0.5,0.));
#29411=DIRECTION('ref_axis',(-0.5,0.866025403784439,0.));
#29412=DIRECTION('center_axis',(-0.866025403784439,-0.5,0.));
#29413=DIRECTION('ref_axis',(-0.5,0.866025403784439,0.));
#29414=DIRECTION('center_axis',(-0.866025403784439,-0.5,0.));
#29415=DIRECTION('ref_axis',(-0.5,0.866025403784439,0.));
#29416=DIRECTION('center_axis',(-0.866025403784439,0.5,0.));
#29417=DIRECTION('ref_axis',(0.5,0.866025403784439,0.));
#29418=DIRECTION('center_axis',(0.,0.,1.));
#29419=DIRECTION('ref_axis',(1.,0.,0.));
#29420=DIRECTION('',(0.,0.,-1.));
#29421=DIRECTION('center_axis',(0.,0.,1.));
#29422=DIRECTION('ref_axis',(1.,0.,0.));
#29423=DIRECTION('center_axis',(0.,0.,-1.));
#29424=DIRECTION('ref_axis',(-1.,0.,0.));
#29425=DIRECTION('center_axis',(0.,0.,1.));
#29426=DIRECTION('ref_axis',(1.,0.,0.));
#29427=DIRECTION('center_axis',(0.,0.,1.));
#29428=DIRECTION('ref_axis',(1.,0.,0.));
#29429=DIRECTION('',(0.,0.,-1.));
#29430=DIRECTION('center_axis',(0.,0.,1.));
#29431=DIRECTION('ref_axis',(1.,0.,0.));
#29432=DIRECTION('',(0.,0.,-1.));
#34450=CARTESIAN_POINT('',(0.,0.,0.));
#34451=CARTESIAN_POINT('Origin',(0.,-1.28,12.0684548175011));
#34452=CARTESIAN_POINT('',(0.,-1.28,12.0369096350021));
#34453=CARTESIAN_POINT('',(-0.105,-1.28,12.1));
#34454=CARTESIAN_POINT('',(-0.0525,-1.28,12.0684548175011));
#34455=CARTESIAN_POINT('Origin',(0.,-1.28,12.1));
#34456=CARTESIAN_POINT('Origin',(0.,-1.28,12.325));
#34457=CARTESIAN_POINT('',(-0.105,-1.28,12.55));
#34458=CARTESIAN_POINT('',(-0.105,-1.28,12.325));
#34459=CARTESIAN_POINT('Origin',(0.,-1.28,12.55));
#34460=CARTESIAN_POINT('Origin',(0.,-1.28,12.6));
#34461=CARTESIAN_POINT('',(-0.155,-1.28,12.6));
#34462=CARTESIAN_POINT('',(-0.155,-1.28,12.6));
#34463=CARTESIAN_POINT('Origin',(0.,-1.28,12.6));
#34464=CARTESIAN_POINT('Origin',(0.,1.28,12.0684548175011));
#34465=CARTESIAN_POINT('',(0.,1.28,12.0369096350021));
#34466=CARTESIAN_POINT('',(-0.105,1.28,12.1));
#34467=CARTESIAN_POINT('',(-0.0525,1.28,12.0684548175011));
#34468=CARTESIAN_POINT('Origin',(0.,1.28,12.1));
#34469=CARTESIAN_POINT('Origin',(0.,1.28,12.325));
#34470=CARTESIAN_POINT('',(-0.105,1.28,12.55));
#34471=CARTESIAN_POINT('',(-0.105,1.28,12.325));
#34472=CARTESIAN_POINT('Origin',(0.,1.28,12.55));
#34473=CARTESIAN_POINT('Origin',(0.,1.28,12.6));
#34474=CARTESIAN_POINT('',(-0.155,1.28,12.6));
#34475=CARTESIAN_POINT('',(-0.155,1.28,12.6));
#34476=CARTESIAN_POINT('Origin',(0.,1.28,12.6));
#34477=CARTESIAN_POINT('Origin',(2.94448637286709,-1.7,11.8390559402368));
#34478=CARTESIAN_POINT('',(2.94448637286709,-1.7,11.8781118804736));
#34479=CARTESIAN_POINT('',(3.07448637286709,-1.7,11.8));
#34480=CARTESIAN_POINT('',(3.00948637286709,-1.7,11.8390559402368));
#34481=CARTESIAN_POINT('Origin',(2.94448637286709,-1.7,11.8));
#34482=CARTESIAN_POINT('Origin',(2.94448637286709,-1.7,11.625));
#34483=CARTESIAN_POINT('',(3.07448637286709,-1.7,11.45));
#34484=CARTESIAN_POINT('',(3.07448637286709,-1.7,11.625));
#34485=CARTESIAN_POINT('Origin',(2.94448637286709,-1.7,11.45));
#34486=CARTESIAN_POINT('Origin',(2.94448637286709,-1.7,11.4));
#34487=CARTESIAN_POINT('',(3.12448637286709,-1.7,11.4));
#34488=CARTESIAN_POINT('',(3.12448637286709,-1.7,11.4));
#34489=CARTESIAN_POINT('Origin',(2.94448637286709,-1.7,11.4));
#34490=CARTESIAN_POINT('Origin',(-2.94448637286709,-1.7,11.8390559402368));
#34491=CARTESIAN_POINT('',(-2.94448637286709,-1.7,11.8781118804736));
#34492=CARTESIAN_POINT('',(-2.81448637286709,-1.7,11.8));
#34493=CARTESIAN_POINT('',(-2.87948637286709,-1.7,11.8390559402368));
#34494=CARTESIAN_POINT('Origin',(-2.94448637286709,-1.7,11.8));
#34495=CARTESIAN_POINT('Origin',(-2.94448637286709,-1.7,11.625));
#34496=CARTESIAN_POINT('',(-2.81448637286709,-1.7,11.45));
#34497=CARTESIAN_POINT('',(-2.81448637286709,-1.7,11.625));
#34498=CARTESIAN_POINT('Origin',(-2.94448637286709,-1.7,11.45));
#34499=CARTESIAN_POINT('Origin',(-2.94448637286709,-1.7,11.4));
#34500=CARTESIAN_POINT('',(-2.76448637286709,-1.7,11.4));
#34501=CARTESIAN_POINT('',(-2.76448637286709,-1.7,11.4));
#34502=CARTESIAN_POINT('Origin',(-2.94448637286709,-1.7,11.4));
#34503=CARTESIAN_POINT('Origin',(2.0818995585505E-16,3.4,11.8390559402368));
#34504=CARTESIAN_POINT('',(2.0818995585505E-16,3.4,11.8781118804736));
#34505=CARTESIAN_POINT('',(0.13,3.4,11.8));
#34506=CARTESIAN_POINT('',(0.0650000000000002,3.4,11.8390559402368));
#34507=CARTESIAN_POINT('Origin',(2.0818995585505E-16,3.4,11.8));
#34508=CARTESIAN_POINT('Origin',(2.0818995585505E-16,3.4,11.625));
#34509=CARTESIAN_POINT('',(0.13,3.4,11.45));
#34510=CARTESIAN_POINT('',(0.13,3.4,11.625));
#34511=CARTESIAN_POINT('Origin',(2.0818995585505E-16,3.4,11.45));
#34512=CARTESIAN_POINT('Origin',(2.0818995585505E-16,3.4,11.4));
#34513=CARTESIAN_POINT('',(0.18,3.4,11.4));
#34514=CARTESIAN_POINT('',(0.18,3.4,11.4));
#34515=CARTESIAN_POINT('Origin',(2.0818995585505E-16,3.4,11.4));
#34516=CARTESIAN_POINT('Origin',(4.17279956956878,-1.11809827484289,11.3875));
#34517=CARTESIAN_POINT('',(4.04446623623544,-1.11809827484289,11.4));
#34518=CARTESIAN_POINT('Origin',(4.17279956956878,-1.11809827484289,11.4));
#34519=CARTESIAN_POINT('',(4.05279956956878,-1.11809827484289,11.425));
#34520=CARTESIAN_POINT('',(4.04029956956878,-1.11809827484289,11.3875));
#34521=CARTESIAN_POINT('Origin',(4.17279956956878,-1.11809827484289,11.425));
#34522=CARTESIAN_POINT('Origin',(4.17279956956878,-1.11809827484289,11.8));
#34523=CARTESIAN_POINT('',(4.05279956956878,-1.11809827484289,12.175));
#34524=CARTESIAN_POINT('',(4.05279956956878,-1.11809827484289,11.8));
#34525=CARTESIAN_POINT('Origin',(4.17279956956878,-1.11809827484289,12.175));
#34526=CARTESIAN_POINT('Origin',(4.17279956956878,-1.11809827484289,12.1875));
#34527=CARTESIAN_POINT('',(4.02779956956878,-1.11809827484289,12.2));
#34528=CARTESIAN_POINT('',(4.04029956956878,-1.11809827484289,12.1875));
#34529=CARTESIAN_POINT('Origin',(4.17279956956878,-1.11809827484289,12.2));
#34530=CARTESIAN_POINT('Origin',(4.38279956956878,-1.11809827484289,12.2));
#34531=CARTESIAN_POINT('',(3.96279956956878,-1.11809827484289,12.2));
#34532=CARTESIAN_POINT('Origin',(4.17279956956878,-1.11809827484289,12.2));
#34533=CARTESIAN_POINT('Origin',(4.17279956956878,-1.11809827484289,12.4));
#34534=CARTESIAN_POINT('',(3.96279956956878,-1.11809827484289,12.6));
#34535=CARTESIAN_POINT('',(3.96279956956878,-1.11809827484289,12.4));
#34536=CARTESIAN_POINT('Origin',(4.17279956956878,-1.11809827484289,12.6));
#34537=CARTESIAN_POINT('Origin',(3.05470129472588,-3.05470129472589,11.3875));
#34538=CARTESIAN_POINT('',(2.92636796139255,-3.05470129472589,11.4));
#34539=CARTESIAN_POINT('Origin',(3.05470129472588,-3.05470129472589,11.4));
#34540=CARTESIAN_POINT('',(2.93470129472589,-3.05470129472589,11.425));
#34541=CARTESIAN_POINT('',(2.92220129472588,-3.05470129472589,11.3875));
#34542=CARTESIAN_POINT('Origin',(3.05470129472588,-3.05470129472589,11.425));
#34543=CARTESIAN_POINT('Origin',(3.05470129472588,-3.05470129472589,11.8));
#34544=CARTESIAN_POINT('',(2.93470129472589,-3.05470129472589,12.175));
#34545=CARTESIAN_POINT('',(2.93470129472589,-3.05470129472589,11.8));
#34546=CARTESIAN_POINT('Origin',(3.05470129472588,-3.05470129472589,12.175));
#34547=CARTESIAN_POINT('Origin',(3.05470129472588,-3.05470129472589,12.1875));
#34548=CARTESIAN_POINT('',(2.90970129472588,-3.05470129472589,12.2));
#34549=CARTESIAN_POINT('',(2.92220129472588,-3.05470129472589,12.1875));
#34550=CARTESIAN_POINT('Origin',(3.05470129472588,-3.05470129472589,12.2));
#34551=CARTESIAN_POINT('Origin',(3.26470129472588,-3.05470129472589,12.2));
#34552=CARTESIAN_POINT('',(2.84470129472589,-3.05470129472589,12.2));
#34553=CARTESIAN_POINT('Origin',(3.05470129472588,-3.05470129472589,12.2));
#34554=CARTESIAN_POINT('Origin',(3.05470129472588,-3.05470129472589,12.4));
#34555=CARTESIAN_POINT('',(2.84470129472589,-3.05470129472589,12.6));
#34556=CARTESIAN_POINT('',(2.84470129472589,-3.05470129472589,12.4));
#34557=CARTESIAN_POINT('Origin',(3.05470129472588,-3.05470129472589,12.6));
#34558=CARTESIAN_POINT('Origin',(1.11809827484289,-4.17279956956878,11.3875));
#34559=CARTESIAN_POINT('',(0.989764941509555,-4.17279956956878,11.4));
#34560=CARTESIAN_POINT('Origin',(1.11809827484289,-4.17279956956878,11.4));
#34561=CARTESIAN_POINT('',(0.998098274842888,-4.17279956956878,11.425));
#34562=CARTESIAN_POINT('',(0.985598274842888,-4.17279956956878,11.3875));
#34563=CARTESIAN_POINT('Origin',(1.11809827484289,-4.17279956956878,11.425));
#34564=CARTESIAN_POINT('Origin',(1.11809827484289,-4.17279956956878,11.8));
#34565=CARTESIAN_POINT('',(0.998098274842888,-4.17279956956878,12.175));
#34566=CARTESIAN_POINT('',(0.998098274842888,-4.17279956956878,11.8));
#34567=CARTESIAN_POINT('Origin',(1.11809827484289,-4.17279956956878,12.175));
#34568=CARTESIAN_POINT('Origin',(1.11809827484289,-4.17279956956878,12.1875));
#34569=CARTESIAN_POINT('',(0.973098274842888,-4.17279956956878,12.2));
#34570=CARTESIAN_POINT('',(0.985598274842888,-4.17279956956878,12.1875));
#34571=CARTESIAN_POINT('Origin',(1.11809827484289,-4.17279956956878,12.2));
#34572=CARTESIAN_POINT('Origin',(1.32809827484289,-4.17279956956878,12.2));
#34573=CARTESIAN_POINT('',(0.908098274842888,-4.17279956956878,12.2));
#34574=CARTESIAN_POINT('Origin',(1.11809827484289,-4.17279956956878,12.2));
#34575=CARTESIAN_POINT('Origin',(1.11809827484289,-4.17279956956878,12.4));
#34576=CARTESIAN_POINT('',(0.908098274842888,-4.17279956956878,12.6));
#34577=CARTESIAN_POINT('',(0.908098274842888,-4.17279956956878,12.4));
#34578=CARTESIAN_POINT('Origin',(1.11809827484289,-4.17279956956878,12.6));
#34579=CARTESIAN_POINT('Origin',(-1.11809827484289,-4.17279956956878,11.3875));
#34580=CARTESIAN_POINT('',(-1.24643160817622,-4.17279956956878,11.4));
#34581=CARTESIAN_POINT('Origin',(-1.11809827484289,-4.17279956956878,11.4));
#34582=CARTESIAN_POINT('',(-1.23809827484289,-4.17279956956878,11.425));
#34583=CARTESIAN_POINT('',(-1.25059827484289,-4.17279956956878,11.3875));
#34584=CARTESIAN_POINT('Origin',(-1.11809827484289,-4.17279956956878,11.425));
#34585=CARTESIAN_POINT('Origin',(-1.11809827484289,-4.17279956956878,11.8));
#34586=CARTESIAN_POINT('',(-1.23809827484289,-4.17279956956878,12.175));
#34587=CARTESIAN_POINT('',(-1.23809827484289,-4.17279956956878,11.8));
#34588=CARTESIAN_POINT('Origin',(-1.11809827484289,-4.17279956956878,12.175));
#34589=CARTESIAN_POINT('Origin',(-1.11809827484289,-4.17279956956878,12.1875));
#34590=CARTESIAN_POINT('',(-1.26309827484289,-4.17279956956878,12.2));
#34591=CARTESIAN_POINT('',(-1.25059827484289,-4.17279956956878,12.1875));
#34592=CARTESIAN_POINT('Origin',(-1.11809827484289,-4.17279956956878,12.2));
#34593=CARTESIAN_POINT('Origin',(-0.908098274842889,-4.17279956956878,12.2));
#34594=CARTESIAN_POINT('',(-1.32809827484289,-4.17279956956878,12.2));
#34595=CARTESIAN_POINT('Origin',(-1.11809827484289,-4.17279956956878,12.2));
#34596=CARTESIAN_POINT('Origin',(-1.11809827484289,-4.17279956956878,12.4));
#34597=CARTESIAN_POINT('',(-1.32809827484289,-4.17279956956878,12.6));
#34598=CARTESIAN_POINT('',(-1.32809827484289,-4.17279956956878,12.4));
#34599=CARTESIAN_POINT('Origin',(-1.11809827484289,-4.17279956956878,12.6));
#34600=CARTESIAN_POINT('Origin',(-3.05470129472589,-3.05470129472589,11.3875));
#34601=CARTESIAN_POINT('',(-3.18303462805922,-3.05470129472589,11.4));
#34602=CARTESIAN_POINT('Origin',(-3.05470129472589,-3.05470129472589,11.4));
#34603=CARTESIAN_POINT('',(-3.17470129472589,-3.05470129472589,11.425));
#34604=CARTESIAN_POINT('',(-3.18720129472589,-3.05470129472589,11.3875));
#34605=CARTESIAN_POINT('Origin',(-3.05470129472589,-3.05470129472589,11.425));
#34606=CARTESIAN_POINT('Origin',(-3.05470129472589,-3.05470129472589,11.8));
#34607=CARTESIAN_POINT('',(-3.17470129472589,-3.05470129472589,12.175));
#34608=CARTESIAN_POINT('',(-3.17470129472589,-3.05470129472589,11.8));
#34609=CARTESIAN_POINT('Origin',(-3.05470129472589,-3.05470129472589,12.175));
#34610=CARTESIAN_POINT('Origin',(-3.05470129472589,-3.05470129472589,12.1875));
#34611=CARTESIAN_POINT('',(-3.19970129472589,-3.05470129472589,12.2));
#34612=CARTESIAN_POINT('',(-3.18720129472589,-3.05470129472589,12.1875));
#34613=CARTESIAN_POINT('Origin',(-3.05470129472589,-3.05470129472589,12.2));
#34614=CARTESIAN_POINT('Origin',(-2.84470129472589,-3.05470129472589,12.2));
#34615=CARTESIAN_POINT('',(-3.26470129472589,-3.05470129472589,12.2));
#34616=CARTESIAN_POINT('Origin',(-3.05470129472589,-3.05470129472589,12.2));
#34617=CARTESIAN_POINT('Origin',(-3.05470129472589,-3.05470129472589,12.4));
#34618=CARTESIAN_POINT('',(-3.26470129472589,-3.05470129472589,12.6));
#34619=CARTESIAN_POINT('',(-3.26470129472589,-3.05470129472589,12.4));
#34620=CARTESIAN_POINT('Origin',(-3.05470129472589,-3.05470129472589,12.6));
#34621=CARTESIAN_POINT('Origin',(-4.17279956956878,-1.11809827484289,11.3875));
#34622=CARTESIAN_POINT('',(-4.30113290290211,-1.11809827484289,11.4));
#34623=CARTESIAN_POINT('Origin',(-4.17279956956878,-1.11809827484289,11.4));
#34624=CARTESIAN_POINT('',(-4.29279956956878,-1.11809827484289,11.425));
#34625=CARTESIAN_POINT('',(-4.30529956956878,-1.11809827484289,11.3875));
#34626=CARTESIAN_POINT('Origin',(-4.17279956956878,-1.11809827484289,11.425));
#34627=CARTESIAN_POINT('Origin',(-4.17279956956878,-1.11809827484289,11.8));
#34628=CARTESIAN_POINT('',(-4.29279956956878,-1.11809827484289,12.175));
#34629=CARTESIAN_POINT('',(-4.29279956956878,-1.11809827484289,11.8));
#34630=CARTESIAN_POINT('Origin',(-4.17279956956878,-1.11809827484289,12.175));
#34631=CARTESIAN_POINT('Origin',(-4.17279956956878,-1.11809827484289,12.1875));
#34632=CARTESIAN_POINT('',(-4.31779956956878,-1.11809827484289,12.2));
#34633=CARTESIAN_POINT('',(-4.30529956956878,-1.11809827484289,12.1875));
#34634=CARTESIAN_POINT('Origin',(-4.17279956956878,-1.11809827484289,12.2));
#34635=CARTESIAN_POINT('Origin',(-3.96279956956878,-1.11809827484289,12.2));
#34636=CARTESIAN_POINT('',(-4.38279956956878,-1.11809827484289,12.2));
#34637=CARTESIAN_POINT('Origin',(-4.17279956956878,-1.11809827484289,12.2));
#34638=CARTESIAN_POINT('Origin',(-4.17279956956878,-1.11809827484289,12.4));
#34639=CARTESIAN_POINT('',(-4.38279956956878,-1.11809827484289,12.6));
#34640=CARTESIAN_POINT('',(-4.38279956956878,-1.11809827484289,12.4));
#34641=CARTESIAN_POINT('Origin',(-4.17279956956878,-1.11809827484289,12.6));
#34642=CARTESIAN_POINT('Origin',(-4.17279956956877,1.11809827484289,11.3875));
#34643=CARTESIAN_POINT('',(-4.30113290290211,1.11809827484289,11.4));
#34644=CARTESIAN_POINT('Origin',(-4.17279956956877,1.11809827484289,11.4));
#34645=CARTESIAN_POINT('',(-4.29279956956877,1.11809827484289,11.425));
#34646=CARTESIAN_POINT('',(-4.30529956956878,1.11809827484289,11.3875));
#34647=CARTESIAN_POINT('Origin',(-4.17279956956877,1.11809827484289,11.425));
#34648=CARTESIAN_POINT('Origin',(-4.17279956956877,1.11809827484289,11.8));
#34649=CARTESIAN_POINT('',(-4.29279956956877,1.11809827484289,12.175));
#34650=CARTESIAN_POINT('',(-4.29279956956877,1.11809827484289,11.8));
#34651=CARTESIAN_POINT('Origin',(-4.17279956956877,1.11809827484289,12.175));
#34652=CARTESIAN_POINT('Origin',(-4.17279956956877,1.11809827484289,12.1875));
#34653=CARTESIAN_POINT('',(-4.31779956956878,1.11809827484289,12.2));
#34654=CARTESIAN_POINT('',(-4.30529956956878,1.11809827484289,12.1875));
#34655=CARTESIAN_POINT('Origin',(-4.17279956956877,1.11809827484289,12.2));
#34656=CARTESIAN_POINT('Origin',(-3.96279956956877,1.11809827484289,12.2));
#34657=CARTESIAN_POINT('',(-4.38279956956877,1.11809827484289,12.2));
#34658=CARTESIAN_POINT('Origin',(-4.17279956956877,1.11809827484289,12.2));
#34659=CARTESIAN_POINT('Origin',(-4.17279956956877,1.11809827484289,12.4));
#34660=CARTESIAN_POINT('',(-4.38279956956877,1.11809827484289,12.6));
#34661=CARTESIAN_POINT('',(-4.38279956956877,1.11809827484289,12.4));
#34662=CARTESIAN_POINT('Origin',(-4.17279956956877,1.11809827484289,12.6));
#34663=CARTESIAN_POINT('Origin',(-3.05470129472589,3.05470129472589,11.3875));
#34664=CARTESIAN_POINT('',(-3.18303462805922,3.05470129472589,11.4));
#34665=CARTESIAN_POINT('Origin',(-3.05470129472589,3.05470129472589,11.4));
#34666=CARTESIAN_POINT('',(-3.17470129472588,3.05470129472589,11.425));
#34667=CARTESIAN_POINT('',(-3.18720129472588,3.05470129472589,11.3875));
#34668=CARTESIAN_POINT('Origin',(-3.05470129472589,3.05470129472589,11.425));
#34669=CARTESIAN_POINT('Origin',(-3.05470129472589,3.05470129472589,11.8));
#34670=CARTESIAN_POINT('',(-3.17470129472588,3.05470129472589,12.175));
#34671=CARTESIAN_POINT('',(-3.17470129472588,3.05470129472589,11.8));
#34672=CARTESIAN_POINT('Origin',(-3.05470129472589,3.05470129472589,12.175));
#34673=CARTESIAN_POINT('Origin',(-3.05470129472589,3.05470129472589,12.1875));
#34674=CARTESIAN_POINT('',(-3.19970129472588,3.05470129472589,12.2));
#34675=CARTESIAN_POINT('',(-3.18720129472588,3.05470129472589,12.1875));
#34676=CARTESIAN_POINT('Origin',(-3.05470129472589,3.05470129472589,12.2));
#34677=CARTESIAN_POINT('Origin',(-2.84470129472589,3.05470129472589,12.2));
#34678=CARTESIAN_POINT('',(-3.26470129472589,3.05470129472589,12.2));
#34679=CARTESIAN_POINT('Origin',(-3.05470129472589,3.05470129472589,12.2));
#34680=CARTESIAN_POINT('Origin',(-3.05470129472589,3.05470129472589,12.4));
#34681=CARTESIAN_POINT('',(-3.26470129472589,3.05470129472589,12.6));
#34682=CARTESIAN_POINT('',(-3.26470129472589,3.05470129472589,12.4));
#34683=CARTESIAN_POINT('Origin',(-3.05470129472589,3.05470129472589,12.6));
#34684=CARTESIAN_POINT('Origin',(-1.11809827484289,4.17279956956878,11.3875));
#34685=CARTESIAN_POINT('',(-1.24643160817622,4.17279956956878,11.4));
#34686=CARTESIAN_POINT('Origin',(-1.11809827484289,4.17279956956878,11.4));
#34687=CARTESIAN_POINT('',(-1.23809827484289,4.17279956956878,11.425));
#34688=CARTESIAN_POINT('',(-1.25059827484289,4.17279956956878,11.3875));
#34689=CARTESIAN_POINT('Origin',(-1.11809827484289,4.17279956956878,11.425));
#34690=CARTESIAN_POINT('Origin',(-1.11809827484289,4.17279956956878,11.8));
#34691=CARTESIAN_POINT('',(-1.23809827484289,4.17279956956878,12.175));
#34692=CARTESIAN_POINT('',(-1.23809827484289,4.17279956956878,11.8));
#34693=CARTESIAN_POINT('Origin',(-1.11809827484289,4.17279956956878,12.175));
#34694=CARTESIAN_POINT('Origin',(-1.11809827484289,4.17279956956878,12.1875));
#34695=CARTESIAN_POINT('',(-1.26309827484289,4.17279956956878,12.2));
#34696=CARTESIAN_POINT('',(-1.25059827484289,4.17279956956878,12.1875));
#34697=CARTESIAN_POINT('Origin',(-1.11809827484289,4.17279956956878,12.2));
#34698=CARTESIAN_POINT('Origin',(-0.90809827484289,4.17279956956878,12.2));
#34699=CARTESIAN_POINT('',(-1.32809827484289,4.17279956956878,12.2));
#34700=CARTESIAN_POINT('Origin',(-1.11809827484289,4.17279956956878,12.2));
#34701=CARTESIAN_POINT('Origin',(-1.11809827484289,4.17279956956878,12.4));
#34702=CARTESIAN_POINT('',(-1.32809827484289,4.17279956956878,12.6));
#34703=CARTESIAN_POINT('',(-1.32809827484289,4.17279956956878,12.4));
#34704=CARTESIAN_POINT('Origin',(-1.11809827484289,4.17279956956878,12.6));
#34705=CARTESIAN_POINT('Origin',(1.11809827484289,4.17279956956878,11.3875));
#34706=CARTESIAN_POINT('',(0.989764941509557,4.17279956956878,11.4));
#34707=CARTESIAN_POINT('Origin',(1.11809827484289,4.17279956956878,11.4));
#34708=CARTESIAN_POINT('',(0.99809827484289,4.17279956956878,11.425));
#34709=CARTESIAN_POINT('',(0.98559827484289,4.17279956956878,11.3875));
#34710=CARTESIAN_POINT('Origin',(1.11809827484289,4.17279956956878,11.425));
#34711=CARTESIAN_POINT('Origin',(1.11809827484289,4.17279956956878,11.8));
#34712=CARTESIAN_POINT('',(0.99809827484289,4.17279956956878,12.175));
#34713=CARTESIAN_POINT('',(0.99809827484289,4.17279956956878,11.8));
#34714=CARTESIAN_POINT('Origin',(1.11809827484289,4.17279956956878,12.175));
#34715=CARTESIAN_POINT('Origin',(1.11809827484289,4.17279956956878,12.1875));
#34716=CARTESIAN_POINT('',(0.97309827484289,4.17279956956878,12.2));
#34717=CARTESIAN_POINT('',(0.98559827484289,4.17279956956878,12.1875));
#34718=CARTESIAN_POINT('Origin',(1.11809827484289,4.17279956956878,12.2));
#34719=CARTESIAN_POINT('Origin',(1.32809827484289,4.17279956956878,12.2));
#34720=CARTESIAN_POINT('',(0.90809827484289,4.17279956956878,12.2));
#34721=CARTESIAN_POINT('Origin',(1.11809827484289,4.17279956956878,12.2));
#34722=CARTESIAN_POINT('Origin',(1.11809827484289,4.17279956956878,12.4));
#34723=CARTESIAN_POINT('',(0.90809827484289,4.17279956956878,12.6));
#34724=CARTESIAN_POINT('',(0.90809827484289,4.17279956956878,12.4));
#34725=CARTESIAN_POINT('Origin',(1.11809827484289,4.17279956956878,12.6));
#34726=CARTESIAN_POINT('Origin',(3.05470129472589,3.05470129472589,11.3875));
#34727=CARTESIAN_POINT('',(2.92636796139255,3.05470129472589,11.4));
#34728=CARTESIAN_POINT('Origin',(3.05470129472589,3.05470129472589,11.4));
#34729=CARTESIAN_POINT('',(2.93470129472589,3.05470129472589,11.425));
#34730=CARTESIAN_POINT('',(2.92220129472589,3.05470129472589,11.3875));
#34731=CARTESIAN_POINT('Origin',(3.05470129472589,3.05470129472589,11.425));
#34732=CARTESIAN_POINT('Origin',(3.05470129472589,3.05470129472589,11.8));
#34733=CARTESIAN_POINT('',(2.93470129472589,3.05470129472589,12.175));
#34734=CARTESIAN_POINT('',(2.93470129472589,3.05470129472589,11.8));
#34735=CARTESIAN_POINT('Origin',(3.05470129472589,3.05470129472589,12.175));
#34736=CARTESIAN_POINT('Origin',(3.05470129472589,3.05470129472589,12.1875));
#34737=CARTESIAN_POINT('',(2.90970129472589,3.05470129472589,12.2));
#34738=CARTESIAN_POINT('',(2.92220129472589,3.05470129472589,12.1875));
#34739=CARTESIAN_POINT('Origin',(3.05470129472589,3.05470129472589,12.2));
#34740=CARTESIAN_POINT('Origin',(3.26470129472589,3.05470129472589,12.2));
#34741=CARTESIAN_POINT('',(2.84470129472589,3.05470129472589,12.2));
#34742=CARTESIAN_POINT('Origin',(3.05470129472589,3.05470129472589,12.2));
#34743=CARTESIAN_POINT('Origin',(3.05470129472589,3.05470129472589,12.4));
#34744=CARTESIAN_POINT('',(2.84470129472589,3.05470129472589,12.6));
#34745=CARTESIAN_POINT('',(2.84470129472589,3.05470129472589,12.4));
#34746=CARTESIAN_POINT('Origin',(3.05470129472589,3.05470129472589,12.6));
#34747=CARTESIAN_POINT('Origin',(4.17279956956878,1.11809827484289,11.3875));
#34748=CARTESIAN_POINT('',(4.04446623623544,1.11809827484289,11.4));
#34749=CARTESIAN_POINT('Origin',(4.17279956956878,1.11809827484289,11.4));
#34750=CARTESIAN_POINT('',(4.05279956956878,1.11809827484289,11.425));
#34751=CARTESIAN_POINT('',(4.04029956956878,1.11809827484289,11.3875));
#34752=CARTESIAN_POINT('Origin',(4.17279956956878,1.11809827484289,11.425));
#34753=CARTESIAN_POINT('Origin',(4.17279956956878,1.11809827484289,11.8));
#34754=CARTESIAN_POINT('',(4.05279956956878,1.11809827484289,12.175));
#34755=CARTESIAN_POINT('',(4.05279956956878,1.11809827484289,11.8));
#34756=CARTESIAN_POINT('Origin',(4.17279956956878,1.11809827484289,12.175));
#34757=CARTESIAN_POINT('Origin',(4.17279956956878,1.11809827484289,12.1875));
#34758=CARTESIAN_POINT('',(4.02779956956878,1.11809827484289,12.2));
#34759=CARTESIAN_POINT('',(4.04029956956878,1.11809827484289,12.1875));
#34760=CARTESIAN_POINT('Origin',(4.17279956956878,1.11809827484289,12.2));
#34761=CARTESIAN_POINT('Origin',(4.38279956956878,1.11809827484289,12.2));
#34762=CARTESIAN_POINT('',(3.96279956956878,1.11809827484289,12.2));
#34763=CARTESIAN_POINT('Origin',(4.17279956956878,1.11809827484289,12.2));
#34764=CARTESIAN_POINT('Origin',(4.17279956956878,1.11809827484289,12.4));
#34765=CARTESIAN_POINT('',(3.96279956956878,1.11809827484289,12.6));
#34766=CARTESIAN_POINT('',(3.96279956956878,1.11809827484289,12.4));
#34767=CARTESIAN_POINT('Origin',(4.17279956956878,1.11809827484289,12.6));
#34768=CARTESIAN_POINT('Origin',(0.,0.,11.42));
#34769=CARTESIAN_POINT('',(0.74,-9.06238631369041E-17,11.4));
#34770=CARTESIAN_POINT('Origin',(0.,0.,11.4));
#34771=CARTESIAN_POINT('',(0.7,8.57252759403147E-17,11.44));
#34772=CARTESIAN_POINT('',(0.72,-8.81745695386094E-17,11.42));
#34773=CARTESIAN_POINT('',(-0.7,-8.57252759403147E-17,11.44));
#34774=CARTESIAN_POINT('Origin',(0.,0.,11.44));
#34775=CARTESIAN_POINT('Origin',(0.,0.,11.44));
#34776=CARTESIAN_POINT('Origin',(0.,0.,11.6));
#34777=CARTESIAN_POINT('',(0.7,-8.57252759403147E-17,11.76));
#34778=CARTESIAN_POINT('',(-0.7,-8.57252759403147E-17,11.76));
#34779=CARTESIAN_POINT('Origin',(0.,0.,11.76));
#34780=CARTESIAN_POINT('Origin',(0.,0.,11.76));
#34781=CARTESIAN_POINT('',(-0.7,-8.57252759403147E-17,11.6));
#34782=CARTESIAN_POINT('Origin',(3.8,0.,11.4));
#34783=CARTESIAN_POINT('',(-3.8,-4.65365783675994E-16,11.4));
#34784=CARTESIAN_POINT('Origin',(0.,0.,11.4));
#34785=CARTESIAN_POINT('Origin',(0.,0.,11.78));
#34786=CARTESIAN_POINT('',(0.74,9.06238631369041E-17,11.8));
#34787=CARTESIAN_POINT('',(0.72,-8.81745695386094E-17,11.78));
#34788=CARTESIAN_POINT('Origin',(0.,0.,11.8));
#34789=CARTESIAN_POINT('Origin',(0.7,0.,11.8));
#34790=CARTESIAN_POINT('',(-0.9025,-1.10524373623049E-16,11.8));
#34791=CARTESIAN_POINT('Origin',(0.,0.,11.8));
#34792=CARTESIAN_POINT('Origin',(0.,0.,11.415));
#34793=CARTESIAN_POINT('',(4.6,-5.63337527607782E-16,11.43));
#34794=CARTESIAN_POINT('',(-4.6,-5.63337527607782E-16,11.43));
#34795=CARTESIAN_POINT('Origin',(0.,0.,11.43));
#34796=CARTESIAN_POINT('Origin',(0.,0.,11.43));
#34797=CARTESIAN_POINT('',(4.57,5.5966358721034E-16,11.4));
#34798=CARTESIAN_POINT('',(4.585,5.61500557409061E-16,11.415));
#34799=CARTESIAN_POINT('Origin',(0.,0.,11.4));
#34800=CARTESIAN_POINT('Origin',(0.,0.,12.));
#34801=CARTESIAN_POINT('',(4.6,5.63337527607782E-16,12.57));
#34802=CARTESIAN_POINT('',(-4.6,-5.63337527607782E-16,12.57));
#34803=CARTESIAN_POINT('Origin',(0.,0.,12.57));
#34804=CARTESIAN_POINT('Origin',(0.,0.,12.57));
#34805=CARTESIAN_POINT('',(-4.6,-5.63337527607782E-16,12.));
#34806=CARTESIAN_POINT('Origin',(4.6,0.,11.4));
#34807=CARTESIAN_POINT('',(-4.095,-5.01492864250841E-16,11.4));
#34808=CARTESIAN_POINT('Origin',(0.,0.,11.4));
#34809=CARTESIAN_POINT('Origin',(0.,0.,12.585));
#34810=CARTESIAN_POINT('',(4.57,-5.5966358721034E-16,12.6));
#34811=CARTESIAN_POINT('Origin',(0.,0.,12.6));
#34812=CARTESIAN_POINT('',(4.585,5.61500557409061E-16,12.585));
#34813=CARTESIAN_POINT('Origin',(0.9025,0.,12.6));
#34814=CARTESIAN_POINT('',(-3.83444475923175,-0.338546858194397,12.6));
#34815=CARTESIAN_POINT('',(-3.20429399400242,-1.43,12.6));
#34816=CARTESIAN_POINT('',(-3.36139274484857,-1.15789698172886,12.6));
#34817=CARTESIAN_POINT('',(-3.30821704245656,-1.61,12.6));
#34818=CARTESIAN_POINT('Origin',(-3.30821704245656,-1.49,12.6));
#34819=CARTESIAN_POINT('',(-3.66167994232156,-1.61,12.6));
#34820=CARTESIAN_POINT('',(-1.09893547277415,-1.61,12.6));
#34821=CARTESIAN_POINT('',(-3.989475518093,-0.289974292889239,12.6));
#34822=CARTESIAN_POINT('Origin',(0.,0.,12.6));
#34823=CARTESIAN_POINT('Origin',(-3.93836780768588,-0.398546858194397,12.6));
#34824=CARTESIAN_POINT('',(-3.66167994232156,1.61,12.6));
#34825=CARTESIAN_POINT('',(-3.989475518093,0.289974292889239,12.6));
#34826=CARTESIAN_POINT('Origin',(0.,0.,12.6));
#34827=CARTESIAN_POINT('',(-3.30821704245656,1.61,12.6));
#34828=CARTESIAN_POINT('',(-1.92454635771531,1.61,12.6));
#34829=CARTESIAN_POINT('',(-3.20429399400242,1.43,12.6));
#34830=CARTESIAN_POINT('Origin',(-3.30821704245656,1.49,12.6));
#34831=CARTESIAN_POINT('',(-3.83444475923175,0.338546858194397,12.6));
#34832=CARTESIAN_POINT('',(-2.94858730237799,1.87289698172886,12.6));
#34833=CARTESIAN_POINT('Origin',(-3.93836780768588,0.398546858194397,12.6));
#34834=CARTESIAN_POINT('',(-3.22514087125372,-2.36610785057841,12.6));
#34835=CARTESIAN_POINT('',(-3.04840942132122,-2.06,12.6));
#34836=CARTESIAN_POINT('',(-2.4693865789506,-1.05710301827114,12.6));
#34837=CARTESIAN_POINT('',(-2.84056332441296,-2.06,12.6));
#34838=CARTESIAN_POINT('Origin',(-2.94448637286709,-2.12,12.6));
#34839=CARTESIAN_POINT('',(-2.21041255918363,-3.1514531418056,12.6));
#34840=CARTESIAN_POINT('',(-2.87064501603739,-2.00789698172886,12.6));
#34841=CARTESIAN_POINT('',(-2.24586286313301,-3.31,12.6));
#34842=CARTESIAN_POINT('Origin',(-2.31433560763776,-3.2114531418056,12.6));
#34843=CARTESIAN_POINT('Origin',(0.,0.,12.6));
#34844=CARTESIAN_POINT('',(-2.24586286313301,3.31,12.6));
#34845=CARTESIAN_POINT('',(-3.22514087125372,2.36610785057841,12.6));
#34846=CARTESIAN_POINT('Origin',(0.,0.,12.6));
#34847=CARTESIAN_POINT('',(-2.21041255918363,3.1514531418056,12.6));
#34848=CARTESIAN_POINT('Origin',(-2.31433560763776,3.2114531418056,12.6));
#34849=CARTESIAN_POINT('',(-2.84056332441296,2.06,12.6));
#34850=CARTESIAN_POINT('',(-2.45783957356681,2.72289698172886,12.6));
#34851=CARTESIAN_POINT('',(-3.04840942132122,2.06,12.6));
#34852=CARTESIAN_POINT('Origin',(-2.94448637286709,2.12,12.6));
#34853=CARTESIAN_POINT('',(-2.05658113648002,0.342103018271136,12.6));
#34854=CARTESIAN_POINT('',(-1.62403220004812,-3.49,12.6));
#34855=CARTESIAN_POINT('',(-0.363730669589464,-3.49,12.6));
#34856=CARTESIAN_POINT('',(-0.452303171281764,-3.49,12.6));
#34857=CARTESIAN_POINT('',(-0.259807621135332,-3.67,12.6));
#34858=CARTESIAN_POINT('Origin',(-0.363730669589464,-3.61,12.6));
#34859=CARTESIAN_POINT('',(-0.436539071067832,-3.97610785057841,12.6));
#34860=CARTESIAN_POINT('',(0.732020663705873,-1.95210301827114,12.6));
#34861=CARTESIAN_POINT('',(-1.74361265495999,-3.59997429288924,12.6));
#34862=CARTESIAN_POINT('Origin',(0.,0.,12.6));
#34863=CARTESIAN_POINT('Origin',(-1.62403220004812,-3.61,12.6));
#34864=CARTESIAN_POINT('',(-0.436539071067833,3.97610785057841,12.6));
#34865=CARTESIAN_POINT('',(-1.74361265495999,3.59997429288924,12.6));
#34866=CARTESIAN_POINT('Origin',(0.,0.,12.6));
#34867=CARTESIAN_POINT('',(-0.259807621135332,3.67,12.6));
#34868=CARTESIAN_POINT('',(0.319215221235291,2.66710301827114,12.6));
#34869=CARTESIAN_POINT('',(-0.363730669589465,3.49,12.6));
#34870=CARTESIAN_POINT('Origin',(-0.363730669589464,3.61,12.6));
#34871=CARTESIAN_POINT('',(-1.62403220004812,3.49,12.6));
#34872=CARTESIAN_POINT('',(0.3733077136594,3.49,12.6));
#34873=CARTESIAN_POINT('Origin',(-1.62403220004812,3.61,12.6));
#34874=CARTESIAN_POINT('',(0.436539071067833,-3.97610785057841,12.6));
#34875=CARTESIAN_POINT('',(0.259807621135332,-3.67,12.6));
#34876=CARTESIAN_POINT('',(-0.0935902212352913,-3.05789698172886,12.6));
#34877=CARTESIAN_POINT('',(0.363730669589464,-3.49,12.6));
#34878=CARTESIAN_POINT('Origin',(0.363730669589464,-3.61,12.6));
#34879=CARTESIAN_POINT('',(1.62403220004812,-3.49,12.6));
#34880=CARTESIAN_POINT('',(0.529192286340599,-3.49,12.6));
#34881=CARTESIAN_POINT('',(1.74361265495999,-3.59997429288924,12.6));
#34882=CARTESIAN_POINT('Origin',(1.62403220004812,-3.61,12.6));
#34883=CARTESIAN_POINT('Origin',(0.,0.,12.6));
#34884=CARTESIAN_POINT('',(1.74361265495999,3.59997429288924,12.6));
#34885=CARTESIAN_POINT('',(0.436539071067832,3.97610785057841,12.6));
#34886=CARTESIAN_POINT('Origin',(0.,0.,12.6));
#34887=CARTESIAN_POINT('',(1.62403220004812,3.49,12.6));
#34888=CARTESIAN_POINT('Origin',(1.62403220004812,3.61,12.6));
#34889=CARTESIAN_POINT('',(0.363730669589464,3.49,12.6));
#34890=CARTESIAN_POINT('',(1.35480317128176,3.49,12.6));
#34891=CARTESIAN_POINT('',(0.259807621135332,3.67,12.6));
#34892=CARTESIAN_POINT('Origin',(0.363730669589464,3.61,12.6));
#34893=CARTESIAN_POINT('',(-0.506395663705874,2.34289698172886,12.6));
#34894=CARTESIAN_POINT('',(2.21041255918363,-3.1514531418056,12.6));
#34895=CARTESIAN_POINT('',(2.84056332441296,-2.06,12.6));
#34896=CARTESIAN_POINT('',(2.68346457356681,-2.33210301827114,12.6));
#34897=CARTESIAN_POINT('',(3.04840942132122,-2.06,12.6));
#34898=CARTESIAN_POINT('Origin',(2.94448637286709,-2.12,12.6));
#34899=CARTESIAN_POINT('',(3.22514087125372,-2.36610785057841,12.6));
#34900=CARTESIAN_POINT('',(2.28220613648002,-0.732896981728864,12.6));
#34901=CARTESIAN_POINT('',(2.24586286313301,-3.31,12.6));
#34902=CARTESIAN_POINT('Origin',(0.,0.,12.6));
#34903=CARTESIAN_POINT('Origin',(2.31433560763776,-3.2114531418056,12.6));
#34904=CARTESIAN_POINT('',(3.22514087125372,2.36610785057841,12.6));
#34905=CARTESIAN_POINT('',(2.24586286313301,3.31,12.6));
#34906=CARTESIAN_POINT('Origin',(0.,0.,12.6));
#34907=CARTESIAN_POINT('',(3.04840942132122,2.06,12.6));
#34908=CARTESIAN_POINT('',(2.6950115789506,1.44789698172886,12.6));
#34909=CARTESIAN_POINT('',(2.84056332441296,2.06,12.6));
#34910=CARTESIAN_POINT('Origin',(2.94448637286709,2.12,12.6));
#34911=CARTESIAN_POINT('',(2.21041255918363,3.1514531418056,12.6));
#34912=CARTESIAN_POINT('',(3.09627001603739,1.61710301827114,12.6));
#34913=CARTESIAN_POINT('Origin',(2.31433560763776,3.2114531418056,12.6));
#34914=CARTESIAN_POINT('',(3.66167994232156,-1.61,12.6));
#34915=CARTESIAN_POINT('',(3.30821704245656,-1.61,12.6));
#34916=CARTESIAN_POINT('',(2.82704635771531,-1.61,12.6));
#34917=CARTESIAN_POINT('',(3.20429399400242,-1.43,12.6));
#34918=CARTESIAN_POINT('Origin',(3.30821704245656,-1.49,12.6));
#34919=CARTESIAN_POINT('',(3.83444475923175,-0.338546858194397,12.6));
#34920=CARTESIAN_POINT('',(3.17421230237799,-1.48210301827114,12.6));
#34921=CARTESIAN_POINT('',(3.989475518093,-0.289974292889239,12.6));
#34922=CARTESIAN_POINT('Origin',(3.93836780768588,-0.398546858194397,12.6));
#34923=CARTESIAN_POINT('Origin',(0.,0.,12.6));
#34924=CARTESIAN_POINT('',(3.989475518093,0.289974292889239,12.6));
#34925=CARTESIAN_POINT('',(3.66167994232156,1.61,12.6));
#34926=CARTESIAN_POINT('Origin',(0.,0.,12.6));
#34927=CARTESIAN_POINT('',(3.83444475923175,0.338546858194397,12.6));
#34928=CARTESIAN_POINT('Origin',(3.93836780768588,0.398546858194397,12.6));
#34929=CARTESIAN_POINT('',(3.20429399400242,1.43,12.6));
#34930=CARTESIAN_POINT('',(3.58701774484857,0.767103018271136,12.6));
#34931=CARTESIAN_POINT('',(3.30821704245656,1.61,12.6));
#34932=CARTESIAN_POINT('Origin',(3.30821704245656,1.49,12.6));
#34933=CARTESIAN_POINT('',(2.00143547277415,1.61,12.6));
#34934=CARTESIAN_POINT('',(3.56225116089999,0.09,12.6));
#34935=CARTESIAN_POINT('',(2.32672158483419,0.09,12.6));
#34936=CARTESIAN_POINT('',(2.33629862890413,0.09,12.6));
#34937=CARTESIAN_POINT('',(2.22279853638006,0.27,12.6));
#34938=CARTESIAN_POINT('Origin',(2.32672158483419,0.21,12.6));
#34939=CARTESIAN_POINT('',(2.84056332441296,1.34,12.6));
#34940=CARTESIAN_POINT('',(1.94734298035004,-0.207103018271136,12.6));
#34941=CARTESIAN_POINT('',(3.04840942132122,1.34,12.6));
#34942=CARTESIAN_POINT('Origin',(2.94448637286709,1.28,12.6));
#34943=CARTESIAN_POINT('',(3.66617420935412,0.27,12.6));
#34944=CARTESIAN_POINT('',(3.01832772969679,1.39210301827114,12.6));
#34945=CARTESIAN_POINT('Origin',(3.56225116089999,0.21,12.6));
#34946=CARTESIAN_POINT('',(2.58075570327763,-1.61,12.6));
#34947=CARTESIAN_POINT('',(1.34522612721183,-1.61,12.6));
#34948=CARTESIAN_POINT('',(1.84555090009295,-1.61,12.6));
#34949=CARTESIAN_POINT('',(1.2413030787577,-1.43,12.6));
#34950=CARTESIAN_POINT('Origin',(1.34522612721183,-1.49,12.6));
#34951=CARTESIAN_POINT('',(1.85906786679059,-0.36,12.6));
#34952=CARTESIAN_POINT('',(1.45659525153885,-1.05710301827114,12.6));
#34953=CARTESIAN_POINT('',(2.06691396369886,-0.36,12.6));
#34954=CARTESIAN_POINT('Origin',(1.96299091524473,-0.420000000000001,12.6));
#34955=CARTESIAN_POINT('',(2.68467875173176,-1.43,12.6));
#34956=CARTESIAN_POINT('',(1.79145840766884,0.117103018271136,12.6));
#34957=CARTESIAN_POINT('Origin',(2.58075570327763,-1.49,12.6));
#34958=CARTESIAN_POINT('',(1.59926024565526,-3.31,12.6));
#34959=CARTESIAN_POINT('',(0.363730669589464,-3.31,12.6));
#34960=CARTESIAN_POINT('',(1.35480317128176,-3.31,12.6));
#34961=CARTESIAN_POINT('',(0.259807621135332,-3.13,12.6));
#34962=CARTESIAN_POINT('Origin',(0.363730669589464,-3.19,12.6));
#34963=CARTESIAN_POINT('',(0.877572409168231,-2.06,12.6));
#34964=CARTESIAN_POINT('',(0.965847522727672,-1.90710301827114,12.6));
#34965=CARTESIAN_POINT('',(1.0854185060765,-2.06,12.6));
#34966=CARTESIAN_POINT('Origin',(0.981495457622364,-2.12,12.6));
#34967=CARTESIAN_POINT('',(1.7031832941094,-3.13,12.6));
#34968=CARTESIAN_POINT('',(0.564589085640882,-1.15789698172886,12.6));
#34969=CARTESIAN_POINT('Origin',(1.59926024565526,-3.19,12.6));
#34970=CARTESIAN_POINT('',(2.68467875173176,1.43,12.6));
#34971=CARTESIAN_POINT('',(2.06691396369886,0.36,12.6));
#34972=CARTESIAN_POINT('',(2.20426385013942,0.597896981728864,12.6));
#34973=CARTESIAN_POINT('',(1.85906786679059,0.360000000000001,12.6));
#34974=CARTESIAN_POINT('Origin',(1.96299091524473,0.420000000000001,12.6));
#34975=CARTESIAN_POINT('',(1.2413030787577,1.43,12.6));
#34976=CARTESIAN_POINT('',(1.86940069400944,0.342103018271136,12.6));
#34977=CARTESIAN_POINT('',(1.34522612721183,1.61,12.6));
#34978=CARTESIAN_POINT('Origin',(1.34522612721183,1.49,12.6));
#34979=CARTESIAN_POINT('',(2.58075570327763,1.61,12.6));
#34980=CARTESIAN_POINT('',(1.01994001515178,1.61,12.6));
#34981=CARTESIAN_POINT('Origin',(2.58075570327763,1.49,12.6));
#34982=CARTESIAN_POINT('',(-0.363730669589465,-3.31,12.6));
#34983=CARTESIAN_POINT('',(-1.59926024565526,-3.31,12.6));
#34984=CARTESIAN_POINT('',(0.3733077136594,-3.31,12.6));
#34985=CARTESIAN_POINT('',(-1.7031832941094,-3.13,12.6));
#34986=CARTESIAN_POINT('Origin',(-1.59926024565526,-3.19,12.6));
#34987=CARTESIAN_POINT('',(-1.0854185060765,-2.06,12.6));
#34988=CARTESIAN_POINT('',(-0.751769528111464,-1.48210301827114,12.6));
#34989=CARTESIAN_POINT('',(-0.877572409168231,-2.06,12.6));
#34990=CARTESIAN_POINT('Origin',(-0.981495457622364,-2.12,12.6));
#34991=CARTESIAN_POINT('',(-0.259807621135332,-3.13,12.6));
#34992=CARTESIAN_POINT('',(-1.15302796519825,-1.58289698172886,12.6));
#34993=CARTESIAN_POINT('Origin',(-0.363730669589464,-3.19,12.6));
#34994=CARTESIAN_POINT('',(1.7031832941094,3.13,12.6));
#34995=CARTESIAN_POINT('',(1.0854185060765,2.06,12.6));
#34996=CARTESIAN_POINT('',(0.977394528111464,1.87289698172886,12.6));
#34997=CARTESIAN_POINT('',(0.877572409168231,2.06,12.6));
#34998=CARTESIAN_POINT('Origin',(0.981495457622364,2.12,12.6));
#34999=CARTESIAN_POINT('',(0.259807621135332,3.13,12.6));
#35000=CARTESIAN_POINT('',(1.37865296519825,1.19210301827114,12.6));
#35001=CARTESIAN_POINT('',(0.363730669589464,3.31,12.6));
#35002=CARTESIAN_POINT('Origin',(0.363730669589464,3.19,12.6));
#35003=CARTESIAN_POINT('',(1.59926024565526,3.31,12.6));
#35004=CARTESIAN_POINT('',(0.529192286340599,3.31,12.6));
#35005=CARTESIAN_POINT('Origin',(1.59926024565526,3.19,12.6));
#35006=CARTESIAN_POINT('',(-1.34522612721183,-1.61,12.6));
#35007=CARTESIAN_POINT('',(-2.58075570327763,-1.61,12.6));
#35008=CARTESIAN_POINT('',(-0.117440015151781,-1.61,12.6));
#35009=CARTESIAN_POINT('',(-2.68467875173176,-1.43,12.6));
#35010=CARTESIAN_POINT('Origin',(-2.58075570327763,-1.49,12.6));
#35011=CARTESIAN_POINT('',(-2.06691396369886,-0.360000000000001,12.6));
#35012=CARTESIAN_POINT('',(-1.97863885013942,-0.207103018271136,12.6));
#35013=CARTESIAN_POINT('',(-1.85906786679059,-0.36,12.6));
#35014=CARTESIAN_POINT('Origin',(-1.96299091524473,-0.420000000000001,12.6));
#35015=CARTESIAN_POINT('',(-1.2413030787577,-1.43,12.6));
#35016=CARTESIAN_POINT('',(-1.64377569400944,-0.732896981728864,12.6));
#35017=CARTESIAN_POINT('Origin',(-1.34522612721183,-1.49,12.6));
#35018=CARTESIAN_POINT('',(-0.259807621135332,3.13,12.6));
#35019=CARTESIAN_POINT('',(-0.877572409168231,2.06,12.6));
#35020=CARTESIAN_POINT('',(-0.740222522727672,2.29789698172886,12.6));
#35021=CARTESIAN_POINT('',(-1.0854185060765,2.06,12.6));
#35022=CARTESIAN_POINT('Origin',(-0.981495457622364,2.12,12.6));
#35023=CARTESIAN_POINT('',(-1.7031832941094,3.13,12.6));
#35024=CARTESIAN_POINT('',(-0.338964085640882,0.767103018271136,12.6));
#35025=CARTESIAN_POINT('',(-1.59926024565526,3.31,12.6));
#35026=CARTESIAN_POINT('Origin',(-1.59926024565526,3.19,12.6));
#35027=CARTESIAN_POINT('',(-0.363730669589464,3.31,12.6));
#35028=CARTESIAN_POINT('',(-0.452303171281764,3.31,12.6));
#35029=CARTESIAN_POINT('Origin',(-0.363730669589464,3.19,12.6));
#35030=CARTESIAN_POINT('',(-1.2413030787577,1.43,12.6));
#35031=CARTESIAN_POINT('',(-1.85906786679059,0.360000000000001,12.6));
#35032=CARTESIAN_POINT('',(-1.23097025153885,1.44789698172886,12.6));
#35033=CARTESIAN_POINT('',(-2.06691396369886,0.36,12.6));
#35034=CARTESIAN_POINT('Origin',(-1.96299091524473,0.420000000000001,12.6));
#35035=CARTESIAN_POINT('',(-2.68467875173176,1.43,12.6));
#35036=CARTESIAN_POINT('',(-1.56583340766884,-0.507896981728864,12.6));
#35037=CARTESIAN_POINT('',(-2.58075570327763,1.61,12.6));
#35038=CARTESIAN_POINT('Origin',(-2.58075570327763,1.49,12.6));
#35039=CARTESIAN_POINT('',(-1.34522612721183,1.61,12.6));
#35040=CARTESIAN_POINT('',(-0.943050900092946,1.61,12.6));
#35041=CARTESIAN_POINT('Origin',(-1.34522612721183,1.49,12.6));
#35042=CARTESIAN_POINT('',(-2.22279853638006,-0.27,12.6));
#35043=CARTESIAN_POINT('',(-2.84056332441296,-1.34,12.6));
#35044=CARTESIAN_POINT('',(-1.72171798035004,0.597896981728864,12.6));
#35045=CARTESIAN_POINT('',(-3.04840942132122,-1.34,12.6));
#35046=CARTESIAN_POINT('Origin',(-2.94448637286709,-1.28,12.6));
#35047=CARTESIAN_POINT('',(-3.66617420935412,-0.27,12.6));
#35048=CARTESIAN_POINT('',(-2.79270272969679,-1.78289698172886,12.6));
#35049=CARTESIAN_POINT('',(-3.56225116089999,-0.09,12.6));
#35050=CARTESIAN_POINT('Origin',(-3.56225116089999,-0.21,12.6));
#35051=CARTESIAN_POINT('',(-2.32672158483419,-0.09,12.6));
#35052=CARTESIAN_POINT('',(-1.43379862890413,-0.09,12.6));
#35053=CARTESIAN_POINT('Origin',(-2.32672158483419,-0.21,12.6));
#35054=CARTESIAN_POINT('',(-2.32672158483419,0.09,12.6));
#35055=CARTESIAN_POINT('',(-3.56225116089999,0.09,12.6));
#35056=CARTESIAN_POINT('',(-0.608187743962963,0.09,12.6));
#35057=CARTESIAN_POINT('',(-3.66617420935412,0.27,12.6));
#35058=CARTESIAN_POINT('Origin',(-3.56225116089999,0.21,12.6));
#35059=CARTESIAN_POINT('',(-3.04840942132122,1.34,12.6));
#35060=CARTESIAN_POINT('',(-3.20550817216737,1.06789698172886,12.6));
#35061=CARTESIAN_POINT('',(-2.84056332441296,1.34,12.6));
#35062=CARTESIAN_POINT('Origin',(-2.94448637286709,1.28,12.6));
#35063=CARTESIAN_POINT('',(-2.22279853638006,0.27,12.6));
#35064=CARTESIAN_POINT('',(-2.13452342282062,0.117103018271136,12.6));
#35065=CARTESIAN_POINT('Origin',(-2.32672158483419,0.21,12.6));
#35066=CARTESIAN_POINT('',(-1.34522612721183,1.79,12.6));
#35067=CARTESIAN_POINT('',(-2.58075570327763,1.79,12.6));
#35068=CARTESIAN_POINT('',(-0.117440015151781,1.79,12.6));
#35069=CARTESIAN_POINT('',(-2.68467875173176,1.97,12.6));
#35070=CARTESIAN_POINT('Origin',(-2.58075570327763,1.91,12.6));
#35071=CARTESIAN_POINT('',(-2.06691396369886,3.04,12.6));
#35072=CARTESIAN_POINT('',(-2.71476044335619,1.91789698172886,12.6));
#35073=CARTESIAN_POINT('',(-1.85906786679059,3.04,12.6));
#35074=CARTESIAN_POINT('Origin',(-1.96299091524473,2.98,12.6));
#35075=CARTESIAN_POINT('',(-1.2413030787577,1.97,12.6));
#35076=CARTESIAN_POINT('',(-0.907654100792664,1.39210301827114,12.6));
#35077=CARTESIAN_POINT('Origin',(-1.34522612721183,1.91,12.6));
#35078=CARTESIAN_POINT('',(-1.2413030787577,-1.97,12.6));
#35079=CARTESIAN_POINT('',(-1.85906786679059,-3.04,12.6));
#35080=CARTESIAN_POINT('',(-0.494848658322081,-0.677103018271136,12.6));
#35081=CARTESIAN_POINT('',(-2.06691396369886,-3.04,12.6));
#35082=CARTESIAN_POINT('Origin',(-1.96299091524473,-2.98,12.6));
#35083=CARTESIAN_POINT('',(-2.68467875173176,-1.97,12.6));
#35084=CARTESIAN_POINT('',(-2.30195500088561,-2.63289698172886,12.6));
#35085=CARTESIAN_POINT('',(-2.58075570327763,-1.79,12.6));
#35086=CARTESIAN_POINT('Origin',(-2.58075570327763,-1.91,12.6));
#35087=CARTESIAN_POINT('',(-1.34522612721183,-1.79,12.6));
#35088=CARTESIAN_POINT('',(-0.943050900092946,-1.79,12.6));
#35089=CARTESIAN_POINT('Origin',(-1.34522612721183,-1.91,12.6));
#35090=CARTESIAN_POINT('',(0.617764788032899,1.79,12.6));
#35091=CARTESIAN_POINT('',(-0.6177647880329,1.79,12.6));
#35092=CARTESIAN_POINT('',(0.864055442470582,1.79,12.6));
#35093=CARTESIAN_POINT('',(-0.721687836487032,1.97,12.6));
#35094=CARTESIAN_POINT('Origin',(-0.6177647880329,1.91,12.6));
#35095=CARTESIAN_POINT('',(-0.103923048454133,3.04,12.6));
#35096=CARTESIAN_POINT('',(-0.997143392517056,1.49289698172886,12.6));
#35097=CARTESIAN_POINT('',(0.103923048454133,3.04,12.6));
#35098=CARTESIAN_POINT('Origin',(8.32667268468867E-17,2.98,12.6));
#35099=CARTESIAN_POINT('',(0.721687836487032,1.97,12.6));
#35100=CARTESIAN_POINT('',(0.809962950046473,1.81710301827114,12.6));
#35101=CARTESIAN_POINT('Origin',(0.617764788032899,1.91,12.6));
#35102=CARTESIAN_POINT('',(0.721687836487032,-1.97,12.6));
#35103=CARTESIAN_POINT('',(0.103923048454133,-3.04,12.6));
#35104=CARTESIAN_POINT('',(1.22276839251706,-1.10210301827114,12.6));
#35105=CARTESIAN_POINT('',(-0.103923048454133,-3.04,12.6));
#35106=CARTESIAN_POINT('Origin',(-8.32667268468867E-17,-2.98,12.6));
#35107=CARTESIAN_POINT('',(-0.721687836487032,-1.97,12.6));
#35108=CARTESIAN_POINT('',(-0.584337950046473,-2.20789698172886,12.6));
#35109=CARTESIAN_POINT('',(-0.617764788032899,-1.79,12.6));
#35110=CARTESIAN_POINT('Origin',(-0.617764788032899,-1.91,12.6));
#35111=CARTESIAN_POINT('',(0.6177647880329,-1.79,12.6));
#35112=CARTESIAN_POINT('',(0.0384445575294176,-1.79,12.6));
#35113=CARTESIAN_POINT('Origin',(0.6177647880329,-1.91,12.6));
#35114=CARTESIAN_POINT('',(2.58075570327763,1.79,12.6));
#35115=CARTESIAN_POINT('',(1.34522612721183,1.79,12.6));
#35116=CARTESIAN_POINT('',(1.84555090009295,1.79,12.6));
#35117=CARTESIAN_POINT('',(1.2413030787577,1.97,12.6));
#35118=CARTESIAN_POINT('Origin',(1.34522612721183,1.91,12.6));
#35119=CARTESIAN_POINT('',(1.85906786679059,3.04,12.6));
#35120=CARTESIAN_POINT('',(0.720473658322081,1.06789698172886,12.6));
#35121=CARTESIAN_POINT('',(2.06691396369886,3.04,12.6));
#35122=CARTESIAN_POINT('Origin',(1.96299091524473,2.98,12.6));
#35123=CARTESIAN_POINT('',(2.68467875173176,1.97,12.6));
#35124=CARTESIAN_POINT('',(2.52758000088561,2.24210301827114,12.6));
#35125=CARTESIAN_POINT('Origin',(2.58075570327763,1.91,12.6));
#35126=CARTESIAN_POINT('',(2.68467875173176,-1.97,12.6));
#35127=CARTESIAN_POINT('',(2.06691396369886,-3.04,12.6));
#35128=CARTESIAN_POINT('',(2.94038544335619,-1.52710301827114,12.6));
#35129=CARTESIAN_POINT('',(1.85906786679059,-3.04,12.6));
#35130=CARTESIAN_POINT('Origin',(1.96299091524473,-2.98,12.6));
#35131=CARTESIAN_POINT('',(1.2413030787577,-1.97,12.6));
#35132=CARTESIAN_POINT('',(1.13327910079266,-1.78289698172886,12.6));
#35133=CARTESIAN_POINT('',(1.34522612721183,-1.79,12.6));
#35134=CARTESIAN_POINT('Origin',(1.34522612721183,-1.91,12.6));
#35135=CARTESIAN_POINT('',(2.58075570327763,-1.79,12.6));
#35136=CARTESIAN_POINT('',(1.01994001515178,-1.79,12.6));
#35137=CARTESIAN_POINT('Origin',(2.58075570327763,-1.91,12.6));
#35138=CARTESIAN_POINT('',(3.66617420935412,-0.27,12.6));
#35139=CARTESIAN_POINT('',(3.04840942132122,-1.34,12.6));
#35140=CARTESIAN_POINT('',(3.43113317216737,-0.677103018271136,12.6));
#35141=CARTESIAN_POINT('',(2.84056332441296,-1.34,12.6));
#35142=CARTESIAN_POINT('Origin',(2.94448637286709,-1.28,12.6));
#35143=CARTESIAN_POINT('',(2.22279853638006,-0.27,12.6));
#35144=CARTESIAN_POINT('',(2.36014842282062,-0.507896981728864,12.6));
#35145=CARTESIAN_POINT('',(2.32672158483419,-0.09,12.6));
#35146=CARTESIAN_POINT('Origin',(2.32672158483419,-0.21,12.6));
#35147=CARTESIAN_POINT('',(3.56225116089999,-0.09,12.6));
#35148=CARTESIAN_POINT('',(1.51068774396296,-0.09,12.6));
#35149=CARTESIAN_POINT('Origin',(3.56225116089999,-0.21,12.6));
#35150=CARTESIAN_POINT('',(-0.9025,-1.10524373623049E-16,12.6));
#35151=CARTESIAN_POINT('Origin',(0.,0.,12.6));
#35152=CARTESIAN_POINT('Origin',(3.93836780768588,-0.398546858194397,12.25));
#35153=CARTESIAN_POINT('',(3.83444475923175,-0.338546858194397,11.9));
#35154=CARTESIAN_POINT('',(3.83444475923175,-0.338546858194397,12.25));
#35155=CARTESIAN_POINT('',(3.989475518093,-0.289974292889239,11.9));
#35156=CARTESIAN_POINT('Origin',(3.93836780768588,-0.398546858194397,11.9));
#35157=CARTESIAN_POINT('',(3.989475518093,-0.289974292889239,12.25));
#35158=CARTESIAN_POINT('Origin',(3.30821704245656,1.49,12.6));
#35159=CARTESIAN_POINT('',(3.30821704245656,1.61,11.9));
#35160=CARTESIAN_POINT('',(3.20429399400242,1.43,11.9));
#35161=CARTESIAN_POINT('Origin',(3.30821704245656,1.49,11.9));
#35162=CARTESIAN_POINT('',(3.30821704245656,1.61,12.6));
#35163=CARTESIAN_POINT('',(3.20429399400242,1.43,12.6));
#35164=CARTESIAN_POINT('Origin',(3.10037094554829,1.61,12.6));
#35165=CARTESIAN_POINT('',(3.66167994232156,1.61,11.9));
#35166=CARTESIAN_POINT('',(4.75159271543062,1.61,11.9));
#35167=CARTESIAN_POINT('',(3.66167994232156,1.61,12.25));
#35168=CARTESIAN_POINT('Origin',(3.93836780768588,0.398546858194397,12.25));
#35169=CARTESIAN_POINT('',(3.83444475923175,0.338546858194397,11.9));
#35170=CARTESIAN_POINT('',(3.989475518093,0.289974292889239,11.9));
#35171=CARTESIAN_POINT('Origin',(3.93836780768588,0.398546858194397,11.9));
#35172=CARTESIAN_POINT('',(3.83444475923175,0.338546858194397,12.25));
#35173=CARTESIAN_POINT('',(3.989475518093,0.289974292889239,12.25));
#35174=CARTESIAN_POINT('Origin',(3.92598183048946,0.895,11.9));
#35175=CARTESIAN_POINT('',(3.10037094554829,1.61,11.9));
#35176=CARTESIAN_POINT('Origin',(0.,0.,11.9));
#35177=CARTESIAN_POINT('Origin',(2.32672158483419,-0.21,12.6));
#35178=CARTESIAN_POINT('',(2.32672158483419,-0.09,11.9));
#35179=CARTESIAN_POINT('',(2.22279853638006,-0.27,11.9));
#35180=CARTESIAN_POINT('Origin',(2.32672158483419,-0.21,11.9));
#35181=CARTESIAN_POINT('',(2.32672158483419,-0.09,12.6));
#35182=CARTESIAN_POINT('',(2.22279853638006,-0.27,12.6));
#35183=CARTESIAN_POINT('Origin',(2.11887548792593,-0.09,12.6));
#35184=CARTESIAN_POINT('',(3.56225116089999,-0.09,11.9));
#35185=CARTESIAN_POINT('',(3.77009725780826,-0.09,11.9));
#35186=CARTESIAN_POINT('',(3.56225116089999,-0.09,12.6));
#35187=CARTESIAN_POINT('Origin',(2.94448637286709,-1.28,12.6));
#35188=CARTESIAN_POINT('',(2.84056332441296,-1.34,11.9));
#35189=CARTESIAN_POINT('',(3.04840942132122,-1.34,11.9));
#35190=CARTESIAN_POINT('Origin',(2.94448637286709,-1.28,11.9));
#35191=CARTESIAN_POINT('',(2.84056332441296,-1.34,12.6));
#35192=CARTESIAN_POINT('',(3.04840942132122,-1.34,12.6));
#35193=CARTESIAN_POINT('Origin',(2.94448637286709,-0.805,11.9));
#35194=CARTESIAN_POINT('',(2.11887548792593,-0.09,11.9));
#35195=CARTESIAN_POINT('',(3.66617420935412,-0.27,11.9));
#35196=CARTESIAN_POINT('',(2.94448637286709,-1.52,11.9));
#35197=CARTESIAN_POINT('Origin',(3.56225116089999,-0.21,11.9));
#35198=CARTESIAN_POINT('Origin',(3.77009725780826,-0.0900000000000001,12.6));
#35199=CARTESIAN_POINT('',(3.66617420935412,-0.27,12.6));
#35200=CARTESIAN_POINT('Origin',(3.56225116089999,-0.21,12.6));
#35201=CARTESIAN_POINT('Origin',(1.34522612721183,-1.91,12.6));
#35202=CARTESIAN_POINT('',(1.34522612721183,-1.79,11.9));
#35203=CARTESIAN_POINT('',(1.2413030787577,-1.97,11.9));
#35204=CARTESIAN_POINT('Origin',(1.34522612721183,-1.91,11.9));
#35205=CARTESIAN_POINT('',(1.34522612721183,-1.79,12.6));
#35206=CARTESIAN_POINT('',(1.2413030787577,-1.97,12.6));
#35207=CARTESIAN_POINT('Origin',(1.13738003030356,-1.79,12.6));
#35208=CARTESIAN_POINT('',(2.58075570327763,-1.79,11.9));
#35209=CARTESIAN_POINT('',(2.78860180018589,-1.79,11.9));
#35210=CARTESIAN_POINT('',(2.58075570327763,-1.79,12.6));
#35211=CARTESIAN_POINT('Origin',(1.96299091524473,-2.98,12.6));
#35212=CARTESIAN_POINT('',(1.85906786679059,-3.04,11.9));
#35213=CARTESIAN_POINT('',(2.06691396369886,-3.04,11.9));
#35214=CARTESIAN_POINT('Origin',(1.96299091524473,-2.98,11.9));
#35215=CARTESIAN_POINT('',(1.85906786679059,-3.04,12.6));
#35216=CARTESIAN_POINT('',(2.06691396369886,-3.04,12.6));
#35217=CARTESIAN_POINT('Origin',(1.96299091524473,-2.505,11.9));
#35218=CARTESIAN_POINT('',(1.13738003030356,-1.79,11.9));
#35219=CARTESIAN_POINT('',(2.68467875173176,-1.97,11.9));
#35220=CARTESIAN_POINT('',(1.96299091524473,-3.22,11.9));
#35221=CARTESIAN_POINT('Origin',(2.58075570327763,-1.91,11.9));
#35222=CARTESIAN_POINT('Origin',(2.78860180018589,-1.79,12.6));
#35223=CARTESIAN_POINT('',(2.68467875173176,-1.97,12.6));
#35224=CARTESIAN_POINT('Origin',(2.58075570327763,-1.91,12.6));
#35225=CARTESIAN_POINT('Origin',(1.62403220004812,-3.61,12.25));
#35226=CARTESIAN_POINT('',(1.62403220004812,-3.49,11.9));
#35227=CARTESIAN_POINT('',(1.62403220004812,-3.49,12.25));
#35228=CARTESIAN_POINT('',(1.74361265495999,-3.59997429288924,11.9));
#35229=CARTESIAN_POINT('Origin',(1.62403220004812,-3.61,11.9));
#35230=CARTESIAN_POINT('',(1.74361265495999,-3.59997429288924,12.25));
#35231=CARTESIAN_POINT('Origin',(1.96299091524473,2.98,12.6));
#35232=CARTESIAN_POINT('',(2.06691396369886,3.04,11.9));
#35233=CARTESIAN_POINT('',(1.85906786679059,3.04,11.9));
#35234=CARTESIAN_POINT('Origin',(1.96299091524473,2.98,11.9));
#35235=CARTESIAN_POINT('',(2.06691396369886,3.04,12.6));
#35236=CARTESIAN_POINT('',(1.85906786679059,3.04,12.6));
#35237=CARTESIAN_POINT('Origin',(1.96299091524473,3.22,12.6));
#35238=CARTESIAN_POINT('',(2.68467875173176,1.97,11.9));
#35239=CARTESIAN_POINT('',(2.78860180018589,1.79,11.9));
#35240=CARTESIAN_POINT('',(2.68467875173176,1.97,12.6));
#35241=CARTESIAN_POINT('Origin',(1.34522612721183,1.91,12.6));
#35242=CARTESIAN_POINT('',(1.2413030787577,1.97,11.9));
#35243=CARTESIAN_POINT('',(1.34522612721183,1.79,11.9));
#35244=CARTESIAN_POINT('Origin',(1.34522612721183,1.91,11.9));
#35245=CARTESIAN_POINT('',(1.2413030787577,1.97,12.6));
#35246=CARTESIAN_POINT('',(1.34522612721183,1.79,12.6));
#35247=CARTESIAN_POINT('Origin',(1.96299091524473,2.505,11.9));
#35248=CARTESIAN_POINT('',(1.96299091524473,3.22,11.9));
#35249=CARTESIAN_POINT('',(2.58075570327763,1.79,11.9));
#35250=CARTESIAN_POINT('',(1.13738003030356,1.79,11.9));
#35251=CARTESIAN_POINT('Origin',(2.58075570327763,1.91,11.9));
#35252=CARTESIAN_POINT('Origin',(2.78860180018589,1.79,12.6));
#35253=CARTESIAN_POINT('',(2.58075570327763,1.79,12.6));
#35254=CARTESIAN_POINT('Origin',(2.58075570327763,1.91,12.6));
#35255=CARTESIAN_POINT('Origin',(-0.617764788032899,-1.91,12.6));
#35256=CARTESIAN_POINT('',(-0.617764788032899,-1.79,11.9));
#35257=CARTESIAN_POINT('',(-0.721687836487032,-1.97,11.9));
#35258=CARTESIAN_POINT('Origin',(-0.617764788032899,-1.91,11.9));
#35259=CARTESIAN_POINT('',(-0.617764788032899,-1.79,12.6));
#35260=CARTESIAN_POINT('',(-0.721687836487032,-1.97,12.6));
#35261=CARTESIAN_POINT('Origin',(-0.825610884941165,-1.79,12.6));
#35262=CARTESIAN_POINT('',(0.6177647880329,-1.79,11.9));
#35263=CARTESIAN_POINT('',(0.825610884941165,-1.79,11.9));
#35264=CARTESIAN_POINT('',(0.6177647880329,-1.79,12.6));
#35265=CARTESIAN_POINT('Origin',(-8.32667268468867E-17,-2.98,12.6));
#35266=CARTESIAN_POINT('',(-0.103923048454133,-3.04,11.9));
#35267=CARTESIAN_POINT('',(0.103923048454133,-3.04,11.9));
#35268=CARTESIAN_POINT('Origin',(-8.32667268468867E-17,-2.98,11.9));
#35269=CARTESIAN_POINT('',(-0.103923048454133,-3.04,12.6));
#35270=CARTESIAN_POINT('',(0.103923048454133,-3.04,12.6));
#35271=CARTESIAN_POINT('Origin',(0.,-2.505,11.9));
#35272=CARTESIAN_POINT('',(-0.825610884941165,-1.79,11.9));
#35273=CARTESIAN_POINT('',(0.721687836487032,-1.97,11.9));
#35274=CARTESIAN_POINT('',(0.,-3.22,11.9));
#35275=CARTESIAN_POINT('Origin',(0.6177647880329,-1.91,11.9));
#35276=CARTESIAN_POINT('Origin',(0.825610884941165,-1.79,12.6));
#35277=CARTESIAN_POINT('',(0.721687836487032,-1.97,12.6));
#35278=CARTESIAN_POINT('Origin',(0.6177647880329,-1.91,12.6));
#35279=CARTESIAN_POINT('Origin',(-0.363730669589464,-3.61,12.6));
#35280=CARTESIAN_POINT('',(-0.259807621135332,-3.67,11.9));
#35281=CARTESIAN_POINT('',(-0.363730669589464,-3.49,11.9));
#35282=CARTESIAN_POINT('Origin',(-0.363730669589464,-3.61,11.9));
#35283=CARTESIAN_POINT('',(-0.259807621135332,-3.67,12.6));
#35284=CARTESIAN_POINT('',(-0.363730669589464,-3.49,12.6));
#35285=CARTESIAN_POINT('Origin',(-0.155884572681199,-3.49,12.6));
#35286=CARTESIAN_POINT('',(-0.436539071067832,-3.97610785057841,11.9));
#35287=CARTESIAN_POINT('',(-0.981495457622364,-4.92,11.9));
#35288=CARTESIAN_POINT('',(-0.436539071067832,-3.97610785057841,12.25));
#35289=CARTESIAN_POINT('Origin',(0.363730669589464,3.61,12.6));
#35290=CARTESIAN_POINT('',(0.259807621135332,3.67,11.9));
#35291=CARTESIAN_POINT('',(0.363730669589464,3.49,11.9));
#35292=CARTESIAN_POINT('Origin',(0.363730669589464,3.61,11.9));
#35293=CARTESIAN_POINT('',(0.259807621135332,3.67,12.6));
#35294=CARTESIAN_POINT('',(0.363730669589464,3.49,12.6));
#35295=CARTESIAN_POINT('Origin',(0.981495457622364,4.205,11.9));
#35296=CARTESIAN_POINT('',(1.62403220004812,3.49,11.9));
#35297=CARTESIAN_POINT('',(0.155884572681199,3.49,11.9));
#35298=CARTESIAN_POINT('',(1.74361265495999,3.59997429288924,11.9));
#35299=CARTESIAN_POINT('Origin',(1.62403220004812,3.61,11.9));
#35300=CARTESIAN_POINT('',(0.436539071067832,3.97610785057841,11.9));
#35301=CARTESIAN_POINT('Origin',(0.,0.,11.9));
#35302=CARTESIAN_POINT('',(0.981495457622364,4.92,11.9));
#35303=CARTESIAN_POINT('Origin',(1.80710634256353,3.49,12.6));
#35304=CARTESIAN_POINT('',(1.62403220004812,3.49,12.25));
#35305=CARTESIAN_POINT('Origin',(1.62403220004812,3.61,12.25));
#35306=CARTESIAN_POINT('',(1.74361265495999,3.59997429288924,12.25));
#35307=CARTESIAN_POINT('Origin',(8.32667268468867E-17,2.98,12.6));
#35308=CARTESIAN_POINT('',(0.103923048454133,3.04,11.9));
#35309=CARTESIAN_POINT('',(-0.103923048454133,3.04,11.9));
#35310=CARTESIAN_POINT('Origin',(8.32667268468867E-17,2.98,11.9));
#35311=CARTESIAN_POINT('',(0.103923048454133,3.04,12.6));
#35312=CARTESIAN_POINT('',(-0.103923048454133,3.04,12.6));
#35313=CARTESIAN_POINT('Origin',(0.,3.22,12.6));
#35314=CARTESIAN_POINT('',(0.721687836487032,1.97,11.9));
#35315=CARTESIAN_POINT('',(0.825610884941165,1.79,11.9));
#35316=CARTESIAN_POINT('',(0.721687836487032,1.97,12.6));
#35317=CARTESIAN_POINT('Origin',(-0.6177647880329,1.91,12.6));
#35318=CARTESIAN_POINT('',(-0.721687836487032,1.97,11.9));
#35319=CARTESIAN_POINT('',(-0.6177647880329,1.79,11.9));
#35320=CARTESIAN_POINT('Origin',(-0.6177647880329,1.91,11.9));
#35321=CARTESIAN_POINT('',(-0.721687836487032,1.97,12.6));
#35322=CARTESIAN_POINT('',(-0.6177647880329,1.79,12.6));
#35323=CARTESIAN_POINT('Origin',(0.,2.505,11.9));
#35324=CARTESIAN_POINT('',(0.,3.22,11.9));
#35325=CARTESIAN_POINT('',(0.617764788032899,1.79,11.9));
#35326=CARTESIAN_POINT('',(-0.825610884941165,1.79,11.9));
#35327=CARTESIAN_POINT('Origin',(0.617764788032899,1.91,11.9));
#35328=CARTESIAN_POINT('Origin',(0.825610884941165,1.79,12.6));
#35329=CARTESIAN_POINT('',(0.617764788032899,1.79,12.6));
#35330=CARTESIAN_POINT('Origin',(0.617764788032899,1.91,12.6));
#35331=CARTESIAN_POINT('Origin',(-2.58075570327763,-1.91,12.6));
#35332=CARTESIAN_POINT('',(-2.58075570327763,-1.79,11.9));
#35333=CARTESIAN_POINT('',(-2.68467875173176,-1.97,11.9));
#35334=CARTESIAN_POINT('Origin',(-2.58075570327763,-1.91,11.9));
#35335=CARTESIAN_POINT('',(-2.58075570327763,-1.79,12.6));
#35336=CARTESIAN_POINT('',(-2.68467875173176,-1.97,12.6));
#35337=CARTESIAN_POINT('Origin',(-2.78860180018589,-1.79,12.6));
#35338=CARTESIAN_POINT('',(-1.34522612721183,-1.79,11.9));
#35339=CARTESIAN_POINT('',(-1.13738003030356,-1.79,11.9));
#35340=CARTESIAN_POINT('',(-1.34522612721183,-1.79,12.6));
#35341=CARTESIAN_POINT('Origin',(-1.96299091524473,-2.98,12.6));
#35342=CARTESIAN_POINT('',(-2.06691396369886,-3.04,11.9));
#35343=CARTESIAN_POINT('',(-1.85906786679059,-3.04,11.9));
#35344=CARTESIAN_POINT('Origin',(-1.96299091524473,-2.98,11.9));
#35345=CARTESIAN_POINT('',(-2.06691396369886,-3.04,12.6));
#35346=CARTESIAN_POINT('',(-1.85906786679059,-3.04,12.6));
#35347=CARTESIAN_POINT('Origin',(-1.96299091524473,-2.505,11.9));
#35348=CARTESIAN_POINT('',(-2.78860180018589,-1.79,11.9));
#35349=CARTESIAN_POINT('',(-1.2413030787577,-1.97,11.9));
#35350=CARTESIAN_POINT('',(-1.96299091524473,-3.22,11.9));
#35351=CARTESIAN_POINT('Origin',(-1.34522612721183,-1.91,11.9));
#35352=CARTESIAN_POINT('Origin',(-1.13738003030356,-1.79,12.6));
#35353=CARTESIAN_POINT('',(-1.2413030787577,-1.97,12.6));
#35354=CARTESIAN_POINT('Origin',(-1.34522612721183,-1.91,12.6));
#35355=CARTESIAN_POINT('Origin',(-1.62403220004812,3.61,12.25));
#35356=CARTESIAN_POINT('',(-1.62403220004812,3.49,11.9));
#35357=CARTESIAN_POINT('',(-1.62403220004812,3.49,12.25));
#35358=CARTESIAN_POINT('',(-1.74361265495999,3.59997429288924,11.9));
#35359=CARTESIAN_POINT('Origin',(-1.62403220004812,3.61,11.9));
#35360=CARTESIAN_POINT('',(-1.74361265495999,3.59997429288924,12.25));
#35361=CARTESIAN_POINT('Origin',(-0.981495457622364,4.205,11.9));
#35362=CARTESIAN_POINT('',(-0.363730669589464,3.49,11.9));
#35363=CARTESIAN_POINT('',(-1.80710634256353,3.49,11.9));
#35364=CARTESIAN_POINT('',(-0.259807621135332,3.67,11.9));
#35365=CARTESIAN_POINT('Origin',(-0.363730669589464,3.61,11.9));
#35366=CARTESIAN_POINT('',(-0.436539071067833,3.97610785057841,11.9));
#35367=CARTESIAN_POINT('',(-0.155884572681199,3.49,11.9));
#35368=CARTESIAN_POINT('Origin',(0.,0.,11.9));
#35369=CARTESIAN_POINT('Origin',(-0.155884572681199,3.49,12.6));
#35370=CARTESIAN_POINT('',(-0.363730669589464,3.49,12.6));
#35371=CARTESIAN_POINT('Origin',(-0.363730669589464,3.61,12.6));
#35372=CARTESIAN_POINT('',(-0.259807621135332,3.67,12.6));
#35373=CARTESIAN_POINT('Origin',(-0.981495457622364,4.92,12.6));
#35374=CARTESIAN_POINT('',(-0.436539071067833,3.97610785057841,12.25));
#35375=CARTESIAN_POINT('Origin',(-1.96299091524473,2.98,12.6));
#35376=CARTESIAN_POINT('',(-1.85906786679059,3.04,11.9));
#35377=CARTESIAN_POINT('',(-2.06691396369886,3.04,11.9));
#35378=CARTESIAN_POINT('Origin',(-1.96299091524473,2.98,11.9));
#35379=CARTESIAN_POINT('',(-1.85906786679059,3.04,12.6));
#35380=CARTESIAN_POINT('',(-2.06691396369886,3.04,12.6));
#35381=CARTESIAN_POINT('Origin',(-1.96299091524473,3.22,12.6));
#35382=CARTESIAN_POINT('',(-1.2413030787577,1.97,11.9));
#35383=CARTESIAN_POINT('',(-1.13738003030356,1.79,11.9));
#35384=CARTESIAN_POINT('',(-1.2413030787577,1.97,12.6));
#35385=CARTESIAN_POINT('Origin',(-2.58075570327763,1.91,12.6));
#35386=CARTESIAN_POINT('',(-2.68467875173176,1.97,11.9));
#35387=CARTESIAN_POINT('',(-2.58075570327763,1.79,11.9));
#35388=CARTESIAN_POINT('Origin',(-2.58075570327763,1.91,11.9));
#35389=CARTESIAN_POINT('',(-2.68467875173176,1.97,12.6));
#35390=CARTESIAN_POINT('',(-2.58075570327763,1.79,12.6));
#35391=CARTESIAN_POINT('Origin',(-1.96299091524473,2.505,11.9));
#35392=CARTESIAN_POINT('',(-1.96299091524473,3.22,11.9));
#35393=CARTESIAN_POINT('',(-1.34522612721183,1.79,11.9));
#35394=CARTESIAN_POINT('',(-2.78860180018589,1.79,11.9));
#35395=CARTESIAN_POINT('Origin',(-1.34522612721183,1.91,11.9));
#35396=CARTESIAN_POINT('Origin',(-1.13738003030356,1.79,12.6));
#35397=CARTESIAN_POINT('',(-1.34522612721183,1.79,12.6));
#35398=CARTESIAN_POINT('Origin',(-1.34522612721183,1.91,12.6));
#35399=CARTESIAN_POINT('Origin',(-2.94448637286709,1.28,12.6));
#35400=CARTESIAN_POINT('',(-2.84056332441296,1.34,11.9));
#35401=CARTESIAN_POINT('',(-3.04840942132122,1.34,11.9));
#35402=CARTESIAN_POINT('Origin',(-2.94448637286709,1.28,11.9));
#35403=CARTESIAN_POINT('',(-2.84056332441296,1.34,12.6));
#35404=CARTESIAN_POINT('',(-3.04840942132122,1.34,12.6));
#35405=CARTESIAN_POINT('Origin',(-2.94448637286709,1.52,12.6));
#35406=CARTESIAN_POINT('',(-2.22279853638006,0.27,11.9));
#35407=CARTESIAN_POINT('',(-2.11887548792593,0.09,11.9));
#35408=CARTESIAN_POINT('',(-2.22279853638006,0.27,12.6));
#35409=CARTESIAN_POINT('Origin',(-3.56225116089999,0.21,12.6));
#35410=CARTESIAN_POINT('',(-3.66617420935412,0.27,11.9));
#35411=CARTESIAN_POINT('',(-3.56225116089999,0.09,11.9));
#35412=CARTESIAN_POINT('Origin',(-3.56225116089999,0.21,11.9));
#35413=CARTESIAN_POINT('',(-3.66617420935412,0.27,12.6));
#35414=CARTESIAN_POINT('',(-3.56225116089999,0.09,12.6));
#35415=CARTESIAN_POINT('Origin',(-2.94448637286709,0.805,11.9));
#35416=CARTESIAN_POINT('',(-2.94448637286709,1.52,11.9));
#35417=CARTESIAN_POINT('',(-2.32672158483419,0.09,11.9));
#35418=CARTESIAN_POINT('',(-3.77009725780826,0.09,11.9));
#35419=CARTESIAN_POINT('Origin',(-2.32672158483419,0.21,11.9));
#35420=CARTESIAN_POINT('Origin',(-2.11887548792593,0.09,12.6));
#35421=CARTESIAN_POINT('',(-2.32672158483419,0.09,12.6));
#35422=CARTESIAN_POINT('Origin',(-2.32672158483419,0.21,12.6));
#35423=CARTESIAN_POINT('Origin',(-3.30821704245656,-1.49,12.6));
#35424=CARTESIAN_POINT('',(-3.30821704245656,-1.61,11.9));
#35425=CARTESIAN_POINT('',(-3.20429399400242,-1.43,11.9));
#35426=CARTESIAN_POINT('Origin',(-3.30821704245656,-1.49,11.9));
#35427=CARTESIAN_POINT('',(-3.30821704245656,-1.61,12.6));
#35428=CARTESIAN_POINT('',(-3.20429399400242,-1.43,12.6));
#35429=CARTESIAN_POINT('Origin',(-3.10037094554829,-1.61,12.6));
#35430=CARTESIAN_POINT('',(-3.66167994232156,-1.61,11.9));
#35431=CARTESIAN_POINT('',(-4.75159271543062,-1.61,11.9));
#35432=CARTESIAN_POINT('',(-3.66167994232156,-1.61,12.25));
#35433=CARTESIAN_POINT('Origin',(-2.94448637286709,2.12,12.6));
#35434=CARTESIAN_POINT('',(-3.04840942132122,2.06,11.9));
#35435=CARTESIAN_POINT('',(-2.84056332441296,2.06,11.9));
#35436=CARTESIAN_POINT('Origin',(-2.94448637286709,2.12,11.9));
#35437=CARTESIAN_POINT('',(-3.04840942132122,2.06,12.6));
#35438=CARTESIAN_POINT('',(-2.84056332441296,2.06,12.6));
#35439=CARTESIAN_POINT('Origin',(-2.94448637286709,2.595,11.9));
#35440=CARTESIAN_POINT('',(-2.21041255918363,3.1514531418056,11.9));
#35441=CARTESIAN_POINT('',(-2.94448637286709,1.88,11.9));
#35442=CARTESIAN_POINT('',(-2.24586286313301,3.31,11.9));
#35443=CARTESIAN_POINT('Origin',(-2.31433560763776,3.2114531418056,11.9));
#35444=CARTESIAN_POINT('',(-3.22514087125372,2.36610785057841,11.9));
#35445=CARTESIAN_POINT('Origin',(0.,0.,11.9));
#35446=CARTESIAN_POINT('',(-3.77009725780826,3.31,11.9));
#35447=CARTESIAN_POINT('Origin',(-2.11887548792593,3.31,12.6));
#35448=CARTESIAN_POINT('',(-2.21041255918363,3.1514531418056,12.25));
#35449=CARTESIAN_POINT('Origin',(-2.31433560763776,3.2114531418056,12.25));
#35450=CARTESIAN_POINT('',(-2.24586286313301,3.31,12.25));
#35451=CARTESIAN_POINT('Origin',(-3.56225116089999,-0.21,12.6));
#35452=CARTESIAN_POINT('',(-3.56225116089999,-0.09,11.9));
#35453=CARTESIAN_POINT('',(-3.66617420935412,-0.27,11.9));
#35454=CARTESIAN_POINT('Origin',(-3.56225116089999,-0.21,11.9));
#35455=CARTESIAN_POINT('',(-3.56225116089999,-0.09,12.6));
#35456=CARTESIAN_POINT('',(-3.66617420935412,-0.27,12.6));
#35457=CARTESIAN_POINT('Origin',(-3.77009725780826,-0.09,12.6));
#35458=CARTESIAN_POINT('',(-2.32672158483419,-0.09,11.9));
#35459=CARTESIAN_POINT('',(-2.11887548792593,-0.09,11.9));
#35460=CARTESIAN_POINT('',(-2.32672158483419,-0.09,12.6));
#35461=CARTESIAN_POINT('Origin',(-2.94448637286709,-1.28,12.6));
#35462=CARTESIAN_POINT('',(-3.04840942132122,-1.34,11.9));
#35463=CARTESIAN_POINT('',(-2.84056332441296,-1.34,11.9));
#35464=CARTESIAN_POINT('Origin',(-2.94448637286709,-1.28,11.9));
#35465=CARTESIAN_POINT('',(-3.04840942132122,-1.34,12.6));
#35466=CARTESIAN_POINT('',(-2.84056332441296,-1.34,12.6));
#35467=CARTESIAN_POINT('Origin',(-2.94448637286709,-0.805,11.9));
#35468=CARTESIAN_POINT('',(-3.77009725780826,-0.09,11.9));
#35469=CARTESIAN_POINT('',(-2.22279853638006,-0.27,11.9));
#35470=CARTESIAN_POINT('',(-2.94448637286709,-1.52,11.9));
#35471=CARTESIAN_POINT('Origin',(-2.32672158483419,-0.21,11.9));
#35472=CARTESIAN_POINT('Origin',(-2.11887548792593,-0.0900000000000001,
12.6));
#35473=CARTESIAN_POINT('',(-2.22279853638006,-0.27,12.6));
#35474=CARTESIAN_POINT('Origin',(-2.32672158483419,-0.21,12.6));
#35475=CARTESIAN_POINT('Origin',(-2.58075570327763,1.49,12.6));
#35476=CARTESIAN_POINT('',(-2.58075570327763,1.61,11.9));
#35477=CARTESIAN_POINT('',(-2.68467875173176,1.43,11.9));
#35478=CARTESIAN_POINT('Origin',(-2.58075570327763,1.49,11.9));
#35479=CARTESIAN_POINT('',(-2.58075570327763,1.61,12.6));
#35480=CARTESIAN_POINT('',(-2.68467875173176,1.43,12.6));
#35481=CARTESIAN_POINT('Origin',(-2.78860180018589,1.61,12.6));
#35482=CARTESIAN_POINT('',(-1.34522612721183,1.61,11.9));
#35483=CARTESIAN_POINT('',(-1.13738003030356,1.61,11.9));
#35484=CARTESIAN_POINT('',(-1.34522612721183,1.61,12.6));
#35485=CARTESIAN_POINT('Origin',(-1.96299091524473,0.420000000000001,12.6));
#35486=CARTESIAN_POINT('',(-2.06691396369886,0.360000000000001,11.9));
#35487=CARTESIAN_POINT('',(-1.85906786679059,0.360000000000001,11.9));
#35488=CARTESIAN_POINT('Origin',(-1.96299091524473,0.420000000000001,11.9));
#35489=CARTESIAN_POINT('',(-2.06691396369886,0.36,12.6));
#35490=CARTESIAN_POINT('',(-1.85906786679059,0.360000000000001,12.6));
#35491=CARTESIAN_POINT('Origin',(-1.96299091524473,0.895,11.9));
#35492=CARTESIAN_POINT('',(-2.78860180018589,1.61,11.9));
#35493=CARTESIAN_POINT('',(-1.2413030787577,1.43,11.9));
#35494=CARTESIAN_POINT('',(-1.96299091524473,0.18,11.9));
#35495=CARTESIAN_POINT('Origin',(-1.34522612721183,1.49,11.9));
#35496=CARTESIAN_POINT('Origin',(-1.13738003030356,1.61,12.6));
#35497=CARTESIAN_POINT('',(-1.2413030787577,1.43,12.6));
#35498=CARTESIAN_POINT('Origin',(-1.34522612721183,1.49,12.6));
#35499=CARTESIAN_POINT('Origin',(-1.59926024565526,3.19,12.6));
#35500=CARTESIAN_POINT('',(-1.59926024565526,3.31,11.9));
#35501=CARTESIAN_POINT('',(-1.7031832941094,3.13,11.9));
#35502=CARTESIAN_POINT('Origin',(-1.59926024565526,3.19,11.9));
#35503=CARTESIAN_POINT('',(-1.59926024565526,3.31,12.6));
#35504=CARTESIAN_POINT('',(-1.7031832941094,3.13,12.6));
#35505=CARTESIAN_POINT('Origin',(-1.80710634256353,3.31,12.6));
#35506=CARTESIAN_POINT('',(-0.363730669589464,3.31,11.9));
#35507=CARTESIAN_POINT('',(-0.155884572681199,3.31,11.9));
#35508=CARTESIAN_POINT('',(-0.363730669589464,3.31,12.6));
#35509=CARTESIAN_POINT('Origin',(-0.981495457622364,2.12,12.6));
#35510=CARTESIAN_POINT('',(-1.0854185060765,2.06,11.9));
#35511=CARTESIAN_POINT('',(-0.877572409168231,2.06,11.9));
#35512=CARTESIAN_POINT('Origin',(-0.981495457622364,2.12,11.9));
#35513=CARTESIAN_POINT('',(-1.0854185060765,2.06,12.6));
#35514=CARTESIAN_POINT('',(-0.877572409168231,2.06,12.6));
#35515=CARTESIAN_POINT('Origin',(-0.981495457622364,2.595,11.9));
#35516=CARTESIAN_POINT('',(-1.80710634256353,3.31,11.9));
#35517=CARTESIAN_POINT('',(-0.259807621135332,3.13,11.9));
#35518=CARTESIAN_POINT('',(-0.981495457622364,1.88,11.9));
#35519=CARTESIAN_POINT('Origin',(-0.363730669589464,3.19,11.9));
#35520=CARTESIAN_POINT('Origin',(-0.155884572681199,3.31,12.6));
#35521=CARTESIAN_POINT('',(-0.259807621135332,3.13,12.6));
#35522=CARTESIAN_POINT('Origin',(-0.363730669589464,3.19,12.6));
#35523=CARTESIAN_POINT('Origin',(-2.31433560763776,-3.2114531418056,12.25));
#35524=CARTESIAN_POINT('',(-2.21041255918363,-3.1514531418056,11.9));
#35525=CARTESIAN_POINT('',(-2.21041255918363,-3.1514531418056,12.25));
#35526=CARTESIAN_POINT('',(-2.24586286313301,-3.31,11.9));
#35527=CARTESIAN_POINT('Origin',(-2.31433560763776,-3.2114531418056,11.9));
#35528=CARTESIAN_POINT('',(-2.24586286313301,-3.31,12.25));
#35529=CARTESIAN_POINT('Origin',(-1.96299091524473,-0.420000000000001,12.6));
#35530=CARTESIAN_POINT('',(-1.85906786679059,-0.360000000000001,11.9));
#35531=CARTESIAN_POINT('',(-2.06691396369886,-0.360000000000001,11.9));
#35532=CARTESIAN_POINT('Origin',(-1.96299091524473,-0.420000000000001,11.9));
#35533=CARTESIAN_POINT('',(-1.85906786679059,-0.360000000000001,12.6));
#35534=CARTESIAN_POINT('',(-2.06691396369886,-0.360000000000001,12.6));
#35535=CARTESIAN_POINT('Origin',(-1.96299091524473,-0.18,12.6));
#35536=CARTESIAN_POINT('',(-1.2413030787577,-1.43,11.9));
#35537=CARTESIAN_POINT('',(-1.13738003030356,-1.61,11.9));
#35538=CARTESIAN_POINT('',(-1.2413030787577,-1.43,12.6));
#35539=CARTESIAN_POINT('Origin',(-2.58075570327763,-1.49,12.6));
#35540=CARTESIAN_POINT('',(-2.68467875173176,-1.43,11.9));
#35541=CARTESIAN_POINT('',(-2.58075570327763,-1.61,11.9));
#35542=CARTESIAN_POINT('Origin',(-2.58075570327763,-1.49,11.9));
#35543=CARTESIAN_POINT('',(-2.68467875173176,-1.43,12.6));
#35544=CARTESIAN_POINT('',(-2.58075570327763,-1.61,12.6));
#35545=CARTESIAN_POINT('Origin',(-1.96299091524473,-0.895,11.9));
#35546=CARTESIAN_POINT('',(-1.96299091524473,-0.18,11.9));
#35547=CARTESIAN_POINT('',(-1.34522612721183,-1.61,11.9));
#35548=CARTESIAN_POINT('',(-2.78860180018589,-1.61,11.9));
#35549=CARTESIAN_POINT('Origin',(-1.34522612721183,-1.49,11.9));
#35550=CARTESIAN_POINT('Origin',(-1.13738003030356,-1.61,12.6));
#35551=CARTESIAN_POINT('',(-1.34522612721183,-1.61,12.6));
#35552=CARTESIAN_POINT('Origin',(-1.34522612721183,-1.49,12.6));
#35553=CARTESIAN_POINT('Origin',(0.363730669589464,3.19,12.6));
#35554=CARTESIAN_POINT('',(0.363730669589464,3.31,11.9));
#35555=CARTESIAN_POINT('',(0.259807621135332,3.13,11.9));
#35556=CARTESIAN_POINT('Origin',(0.363730669589464,3.19,11.9));
#35557=CARTESIAN_POINT('',(0.363730669589464,3.31,12.6));
#35558=CARTESIAN_POINT('',(0.259807621135332,3.13,12.6));
#35559=CARTESIAN_POINT('Origin',(0.155884572681199,3.31,12.6));
#35560=CARTESIAN_POINT('',(1.59926024565526,3.31,11.9));
#35561=CARTESIAN_POINT('',(1.80710634256353,3.31,11.9));
#35562=CARTESIAN_POINT('',(1.59926024565526,3.31,12.6));
#35563=CARTESIAN_POINT('Origin',(0.981495457622364,2.12,12.6));
#35564=CARTESIAN_POINT('',(0.877572409168231,2.06,11.9));
#35565=CARTESIAN_POINT('',(1.0854185060765,2.06,11.9));
#35566=CARTESIAN_POINT('Origin',(0.981495457622364,2.12,11.9));
#35567=CARTESIAN_POINT('',(0.877572409168231,2.06,12.6));
#35568=CARTESIAN_POINT('',(1.0854185060765,2.06,12.6));
#35569=CARTESIAN_POINT('Origin',(0.981495457622364,2.595,11.9));
#35570=CARTESIAN_POINT('',(0.155884572681199,3.31,11.9));
#35571=CARTESIAN_POINT('',(1.7031832941094,3.13,11.9));
#35572=CARTESIAN_POINT('',(0.981495457622364,1.88,11.9));
#35573=CARTESIAN_POINT('Origin',(1.59926024565526,3.19,11.9));
#35574=CARTESIAN_POINT('Origin',(1.80710634256353,3.31,12.6));
#35575=CARTESIAN_POINT('',(1.7031832941094,3.13,12.6));
#35576=CARTESIAN_POINT('Origin',(1.59926024565526,3.19,12.6));
#35577=CARTESIAN_POINT('Origin',(-3.93836780768588,0.398546858194397,12.25));
#35578=CARTESIAN_POINT('',(-3.83444475923175,0.338546858194397,11.9));
#35579=CARTESIAN_POINT('',(-3.83444475923175,0.338546858194397,12.25));
#35580=CARTESIAN_POINT('',(-3.989475518093,0.289974292889239,11.9));
#35581=CARTESIAN_POINT('Origin',(-3.93836780768588,0.398546858194397,11.9));
#35582=CARTESIAN_POINT('',(-3.989475518093,0.289974292889239,12.25));
#35583=CARTESIAN_POINT('Origin',(-3.92598183048946,0.895,11.9));
#35584=CARTESIAN_POINT('',(-3.20429399400242,1.43,11.9));
#35585=CARTESIAN_POINT('',(-3.92598183048946,0.18,11.9));
#35586=CARTESIAN_POINT('',(-3.30821704245656,1.61,11.9));
#35587=CARTESIAN_POINT('Origin',(-3.30821704245656,1.49,11.9));
#35588=CARTESIAN_POINT('',(-3.66167994232156,1.61,11.9));
#35589=CARTESIAN_POINT('',(-3.10037094554829,1.61,11.9));
#35590=CARTESIAN_POINT('Origin',(0.,0.,11.9));
#35591=CARTESIAN_POINT('Origin',(-3.10037094554829,1.61,12.6));
#35592=CARTESIAN_POINT('',(-3.20429399400242,1.43,12.6));
#35593=CARTESIAN_POINT('Origin',(-3.30821704245656,1.49,12.6));
#35594=CARTESIAN_POINT('',(-3.30821704245656,1.61,12.6));
#35595=CARTESIAN_POINT('Origin',(-4.75159271543062,1.61,12.6));
#35596=CARTESIAN_POINT('',(-3.66167994232156,1.61,12.25));
#35597=CARTESIAN_POINT('Origin',(-0.981495457622364,-2.12,12.6));
#35598=CARTESIAN_POINT('',(-0.877572409168231,-2.06,11.9));
#35599=CARTESIAN_POINT('',(-1.0854185060765,-2.06,11.9));
#35600=CARTESIAN_POINT('Origin',(-0.981495457622364,-2.12,11.9));
#35601=CARTESIAN_POINT('',(-0.877572409168231,-2.06,12.6));
#35602=CARTESIAN_POINT('',(-1.0854185060765,-2.06,12.6));
#35603=CARTESIAN_POINT('Origin',(-0.981495457622364,-1.88,12.6));
#35604=CARTESIAN_POINT('',(-0.259807621135332,-3.13,11.9));
#35605=CARTESIAN_POINT('',(-0.155884572681199,-3.31,11.9));
#35606=CARTESIAN_POINT('',(-0.259807621135332,-3.13,12.6));
#35607=CARTESIAN_POINT('Origin',(-1.59926024565526,-3.19,12.6));
#35608=CARTESIAN_POINT('',(-1.7031832941094,-3.13,11.9));
#35609=CARTESIAN_POINT('',(-1.59926024565526,-3.31,11.9));
#35610=CARTESIAN_POINT('Origin',(-1.59926024565526,-3.19,11.9));
#35611=CARTESIAN_POINT('',(-1.7031832941094,-3.13,12.6));
#35612=CARTESIAN_POINT('',(-1.59926024565526,-3.31,12.6));
#35613=CARTESIAN_POINT('Origin',(-0.981495457622364,-2.595,11.9));
#35614=CARTESIAN_POINT('',(-0.981495457622364,-1.88,11.9));
#35615=CARTESIAN_POINT('',(-0.363730669589464,-3.31,11.9));
#35616=CARTESIAN_POINT('',(-1.80710634256353,-3.31,11.9));
#35617=CARTESIAN_POINT('Origin',(-0.363730669589464,-3.19,11.9));
#35618=CARTESIAN_POINT('Origin',(-0.155884572681199,-3.31,12.6));
#35619=CARTESIAN_POINT('',(-0.363730669589464,-3.31,12.6));
#35620=CARTESIAN_POINT('Origin',(-0.363730669589464,-3.19,12.6));
#35621=CARTESIAN_POINT('Origin',(1.34522612721183,1.49,12.6));
#35622=CARTESIAN_POINT('',(1.34522612721183,1.61,11.9));
#35623=CARTESIAN_POINT('',(1.2413030787577,1.43,11.9));
#35624=CARTESIAN_POINT('Origin',(1.34522612721183,1.49,11.9));
#35625=CARTESIAN_POINT('',(1.34522612721183,1.61,12.6));
#35626=CARTESIAN_POINT('',(1.2413030787577,1.43,12.6));
#35627=CARTESIAN_POINT('Origin',(1.13738003030356,1.61,12.6));
#35628=CARTESIAN_POINT('',(2.58075570327763,1.61,11.9));
#35629=CARTESIAN_POINT('',(2.78860180018589,1.61,11.9));
#35630=CARTESIAN_POINT('',(2.58075570327763,1.61,12.6));
#35631=CARTESIAN_POINT('Origin',(1.96299091524473,0.420000000000001,12.6));
#35632=CARTESIAN_POINT('',(1.85906786679059,0.360000000000001,11.9));
#35633=CARTESIAN_POINT('',(2.06691396369886,0.360000000000001,11.9));
#35634=CARTESIAN_POINT('Origin',(1.96299091524473,0.420000000000001,11.9));
#35635=CARTESIAN_POINT('',(1.85906786679059,0.360000000000001,12.6));
#35636=CARTESIAN_POINT('',(2.06691396369886,0.360000000000001,12.6));
#35637=CARTESIAN_POINT('Origin',(1.96299091524473,0.895,11.9));
#35638=CARTESIAN_POINT('',(1.13738003030356,1.61,11.9));
#35639=CARTESIAN_POINT('',(2.68467875173176,1.43,11.9));
#35640=CARTESIAN_POINT('',(1.96299091524473,0.18,11.9));
#35641=CARTESIAN_POINT('Origin',(2.58075570327763,1.49,11.9));
#35642=CARTESIAN_POINT('Origin',(2.78860180018589,1.61,12.6));
#35643=CARTESIAN_POINT('',(2.68467875173176,1.43,12.6));
#35644=CARTESIAN_POINT('Origin',(2.58075570327763,1.49,12.6));
#35645=CARTESIAN_POINT('Origin',(2.31433560763776,3.2114531418056,12.25));
#35646=CARTESIAN_POINT('',(2.21041255918363,3.1514531418056,11.9));
#35647=CARTESIAN_POINT('',(2.21041255918363,3.1514531418056,12.25));
#35648=CARTESIAN_POINT('',(2.24586286313301,3.31,11.9));
#35649=CARTESIAN_POINT('Origin',(2.31433560763776,3.2114531418056,11.9));
#35650=CARTESIAN_POINT('',(2.24586286313301,3.31,12.25));
#35651=CARTESIAN_POINT('Origin',(2.94448637286709,2.12,12.6));
#35652=CARTESIAN_POINT('',(2.84056332441296,2.06,11.9));
#35653=CARTESIAN_POINT('',(3.04840942132122,2.06,11.9));
#35654=CARTESIAN_POINT('Origin',(2.94448637286709,2.12,11.9));
#35655=CARTESIAN_POINT('',(2.84056332441296,2.06,12.6));
#35656=CARTESIAN_POINT('',(3.04840942132122,2.06,12.6));
#35657=CARTESIAN_POINT('Origin',(2.94448637286709,2.595,11.9));
#35658=CARTESIAN_POINT('',(2.11887548792593,3.31,11.9));
#35659=CARTESIAN_POINT('',(3.22514087125372,2.36610785057841,11.9));
#35660=CARTESIAN_POINT('',(2.94448637286709,1.88,11.9));
#35661=CARTESIAN_POINT('Origin',(0.,0.,11.9));
#35662=CARTESIAN_POINT('Origin',(3.77009725780826,3.31,12.6));
#35663=CARTESIAN_POINT('',(3.22514087125372,2.36610785057841,12.25));
#35664=CARTESIAN_POINT('Origin',(0.981495457622364,-2.12,12.6));
#35665=CARTESIAN_POINT('',(1.0854185060765,-2.06,11.9));
#35666=CARTESIAN_POINT('',(0.877572409168231,-2.06,11.9));
#35667=CARTESIAN_POINT('Origin',(0.981495457622364,-2.12,11.9));
#35668=CARTESIAN_POINT('',(1.0854185060765,-2.06,12.6));
#35669=CARTESIAN_POINT('',(0.877572409168231,-2.06,12.6));
#35670=CARTESIAN_POINT('Origin',(0.981495457622364,-1.88,12.6));
#35671=CARTESIAN_POINT('',(1.7031832941094,-3.13,11.9));
#35672=CARTESIAN_POINT('',(1.80710634256353,-3.31,11.9));
#35673=CARTESIAN_POINT('',(1.7031832941094,-3.13,12.6));
#35674=CARTESIAN_POINT('Origin',(0.363730669589464,-3.19,12.6));
#35675=CARTESIAN_POINT('',(0.259807621135332,-3.13,11.9));
#35676=CARTESIAN_POINT('',(0.363730669589464,-3.31,11.9));
#35677=CARTESIAN_POINT('Origin',(0.363730669589464,-3.19,11.9));
#35678=CARTESIAN_POINT('',(0.259807621135332,-3.13,12.6));
#35679=CARTESIAN_POINT('',(0.363730669589464,-3.31,12.6));
#35680=CARTESIAN_POINT('Origin',(0.981495457622364,-2.595,11.9));
#35681=CARTESIAN_POINT('',(0.981495457622364,-1.88,11.9));
#35682=CARTESIAN_POINT('',(1.59926024565526,-3.31,11.9));
#35683=CARTESIAN_POINT('',(0.155884572681199,-3.31,11.9));
#35684=CARTESIAN_POINT('Origin',(1.59926024565526,-3.19,11.9));
#35685=CARTESIAN_POINT('Origin',(1.80710634256353,-3.31,12.6));
#35686=CARTESIAN_POINT('',(1.59926024565526,-3.31,12.6));
#35687=CARTESIAN_POINT('Origin',(1.59926024565526,-3.19,12.6));
#35688=CARTESIAN_POINT('Origin',(1.96299091524473,-0.420000000000001,12.6));
#35689=CARTESIAN_POINT('',(2.06691396369886,-0.360000000000001,11.9));
#35690=CARTESIAN_POINT('',(1.85906786679059,-0.360000000000001,11.9));
#35691=CARTESIAN_POINT('Origin',(1.96299091524473,-0.420000000000001,11.9));
#35692=CARTESIAN_POINT('',(2.06691396369886,-0.36,12.6));
#35693=CARTESIAN_POINT('',(1.85906786679059,-0.360000000000001,12.6));
#35694=CARTESIAN_POINT('Origin',(1.96299091524473,-0.18,12.6));
#35695=CARTESIAN_POINT('',(2.68467875173176,-1.43,11.9));
#35696=CARTESIAN_POINT('',(2.78860180018589,-1.61,11.9));
#35697=CARTESIAN_POINT('',(2.68467875173176,-1.43,12.6));
#35698=CARTESIAN_POINT('Origin',(1.34522612721183,-1.49,12.6));
#35699=CARTESIAN_POINT('',(1.2413030787577,-1.43,11.9));
#35700=CARTESIAN_POINT('',(1.34522612721183,-1.61,11.9));
#35701=CARTESIAN_POINT('Origin',(1.34522612721183,-1.49,11.9));
#35702=CARTESIAN_POINT('',(1.2413030787577,-1.43,12.6));
#35703=CARTESIAN_POINT('',(1.34522612721183,-1.61,12.6));
#35704=CARTESIAN_POINT('Origin',(1.96299091524473,-0.895,11.9));
#35705=CARTESIAN_POINT('',(1.96299091524473,-0.18,11.9));
#35706=CARTESIAN_POINT('',(2.58075570327763,-1.61,11.9));
#35707=CARTESIAN_POINT('',(1.13738003030356,-1.61,11.9));
#35708=CARTESIAN_POINT('Origin',(2.58075570327763,-1.49,11.9));
#35709=CARTESIAN_POINT('Origin',(2.78860180018589,-1.61,12.6));
#35710=CARTESIAN_POINT('',(2.58075570327763,-1.61,12.6));
#35711=CARTESIAN_POINT('Origin',(2.58075570327763,-1.49,12.6));
#35712=CARTESIAN_POINT('Origin',(2.94448637286709,1.28,12.6));
#35713=CARTESIAN_POINT('',(3.04840942132122,1.34,11.9));
#35714=CARTESIAN_POINT('',(2.84056332441296,1.34,11.9));
#35715=CARTESIAN_POINT('Origin',(2.94448637286709,1.28,11.9));
#35716=CARTESIAN_POINT('',(3.04840942132122,1.34,12.6));
#35717=CARTESIAN_POINT('',(2.84056332441296,1.34,12.6));
#35718=CARTESIAN_POINT('Origin',(2.94448637286709,1.52,12.6));
#35719=CARTESIAN_POINT('',(3.66617420935412,0.27,11.9));
#35720=CARTESIAN_POINT('',(3.77009725780826,0.09,11.9));
#35721=CARTESIAN_POINT('',(3.66617420935412,0.27,12.6));
#35722=CARTESIAN_POINT('Origin',(2.32672158483419,0.21,12.6));
#35723=CARTESIAN_POINT('',(2.22279853638006,0.27,11.9));
#35724=CARTESIAN_POINT('',(2.32672158483419,0.09,11.9));
#35725=CARTESIAN_POINT('Origin',(2.32672158483419,0.21,11.9));
#35726=CARTESIAN_POINT('',(2.22279853638006,0.27,12.6));
#35727=CARTESIAN_POINT('',(2.32672158483419,0.09,12.6));
#35728=CARTESIAN_POINT('Origin',(2.94448637286709,0.805,11.9));
#35729=CARTESIAN_POINT('',(2.94448637286709,1.52,11.9));
#35730=CARTESIAN_POINT('',(3.56225116089999,0.09,11.9));
#35731=CARTESIAN_POINT('',(2.11887548792593,0.09,11.9));
#35732=CARTESIAN_POINT('Origin',(3.56225116089999,0.21,11.9));
#35733=CARTESIAN_POINT('Origin',(3.77009725780826,0.09,12.6));
#35734=CARTESIAN_POINT('',(3.56225116089999,0.09,12.6));
#35735=CARTESIAN_POINT('Origin',(3.56225116089999,0.21,12.6));
#35736=CARTESIAN_POINT('Origin',(3.30821704245656,-1.49,12.6));
#35737=CARTESIAN_POINT('',(3.20429399400242,-1.43,11.9));
#35738=CARTESIAN_POINT('',(3.30821704245656,-1.61,11.9));
#35739=CARTESIAN_POINT('Origin',(3.30821704245656,-1.49,11.9));
#35740=CARTESIAN_POINT('',(3.20429399400242,-1.43,12.6));
#35741=CARTESIAN_POINT('',(3.30821704245656,-1.61,12.6));
#35742=CARTESIAN_POINT('Origin',(3.92598183048946,-0.895,11.9));
#35743=CARTESIAN_POINT('',(3.92598183048946,-0.18,11.9));
#35744=CARTESIAN_POINT('',(3.66167994232156,-1.61,11.9));
#35745=CARTESIAN_POINT('',(3.10037094554829,-1.61,11.9));
#35746=CARTESIAN_POINT('Origin',(0.,0.,11.9));
#35747=CARTESIAN_POINT('Origin',(4.75159271543062,-1.61,12.6));
#35748=CARTESIAN_POINT('',(3.66167994232156,-1.61,12.25));
#35749=CARTESIAN_POINT('Origin',(2.94448637286709,-2.12,12.6));
#35750=CARTESIAN_POINT('',(3.04840942132122,-2.06,11.9));
#35751=CARTESIAN_POINT('',(2.84056332441296,-2.06,11.9));
#35752=CARTESIAN_POINT('Origin',(2.94448637286709,-2.12,11.9));
#35753=CARTESIAN_POINT('',(3.04840942132122,-2.06,12.6));
#35754=CARTESIAN_POINT('',(2.84056332441296,-2.06,12.6));
#35755=CARTESIAN_POINT('Origin',(2.94448637286709,-1.88,12.6));
#35756=CARTESIAN_POINT('',(3.22514087125372,-2.36610785057841,11.9));
#35757=CARTESIAN_POINT('',(3.77009725780826,-3.31,11.9));
#35758=CARTESIAN_POINT('',(3.22514087125372,-2.36610785057841,12.25));
#35759=CARTESIAN_POINT('Origin',(2.31433560763776,-3.2114531418056,12.25));
#35760=CARTESIAN_POINT('',(2.21041255918363,-3.1514531418056,11.9));
#35761=CARTESIAN_POINT('',(2.24586286313301,-3.31,11.9));
#35762=CARTESIAN_POINT('Origin',(2.31433560763776,-3.2114531418056,11.9));
#35763=CARTESIAN_POINT('',(2.21041255918363,-3.1514531418056,12.25));
#35764=CARTESIAN_POINT('',(2.24586286313301,-3.31,12.25));
#35765=CARTESIAN_POINT('Origin',(2.94448637286709,-2.595,11.9));
#35766=CARTESIAN_POINT('',(2.94448637286709,-1.88,11.9));
#35767=CARTESIAN_POINT('Origin',(0.,0.,11.9));
#35768=CARTESIAN_POINT('Origin',(0.363730669589464,-3.61,12.6));
#35769=CARTESIAN_POINT('',(0.363730669589464,-3.49,11.9));
#35770=CARTESIAN_POINT('',(0.259807621135332,-3.67,11.9));
#35771=CARTESIAN_POINT('Origin',(0.363730669589464,-3.61,11.9));
#35772=CARTESIAN_POINT('',(0.363730669589464,-3.49,12.6));
#35773=CARTESIAN_POINT('',(0.259807621135332,-3.67,12.6));
#35774=CARTESIAN_POINT('Origin',(0.981495457622364,-4.205,11.9));
#35775=CARTESIAN_POINT('',(1.80710634256353,-3.49,11.9));
#35776=CARTESIAN_POINT('',(0.436539071067832,-3.97610785057841,11.9));
#35777=CARTESIAN_POINT('',(0.155884572681199,-3.49,11.9));
#35778=CARTESIAN_POINT('Origin',(0.,0.,11.9));
#35779=CARTESIAN_POINT('Origin',(0.981495457622364,-4.92,12.6));
#35780=CARTESIAN_POINT('',(0.436539071067833,-3.97610785057841,12.25));
#35781=CARTESIAN_POINT('Origin',(-1.62403220004812,-3.61,12.25));
#35782=CARTESIAN_POINT('',(-1.62403220004812,-3.49,11.9));
#35783=CARTESIAN_POINT('',(-1.74361265495999,-3.59997429288924,11.9));
#35784=CARTESIAN_POINT('Origin',(-1.62403220004812,-3.61,11.9));
#35785=CARTESIAN_POINT('',(-1.62403220004812,-3.49,12.25));
#35786=CARTESIAN_POINT('',(-1.74361265495999,-3.59997429288924,12.25));
#35787=CARTESIAN_POINT('Origin',(-0.981495457622364,-4.205,11.9));
#35788=CARTESIAN_POINT('',(-0.155884572681199,-3.49,11.9));
#35789=CARTESIAN_POINT('Origin',(0.,0.,11.9));
#35790=CARTESIAN_POINT('Origin',(-2.94448637286709,-2.12,12.6));
#35791=CARTESIAN_POINT('',(-2.84056332441296,-2.06,11.9));
#35792=CARTESIAN_POINT('',(-3.04840942132122,-2.06,11.9));
#35793=CARTESIAN_POINT('Origin',(-2.94448637286709,-2.12,11.9));
#35794=CARTESIAN_POINT('',(-2.84056332441296,-2.06,12.6));
#35795=CARTESIAN_POINT('',(-3.04840942132122,-2.06,12.6));
#35796=CARTESIAN_POINT('Origin',(-2.94448637286709,-2.595,11.9));
#35797=CARTESIAN_POINT('',(-2.11887548792593,-3.31,11.9));
#35798=CARTESIAN_POINT('',(-3.22514087125372,-2.36610785057841,11.9));
#35799=CARTESIAN_POINT('',(-2.94448637286709,-1.88,11.9));
#35800=CARTESIAN_POINT('Origin',(0.,0.,11.9));
#35801=CARTESIAN_POINT('Origin',(-3.77009725780826,-3.31,12.6));
#35802=CARTESIAN_POINT('',(-3.22514087125372,-2.36610785057841,12.25));
#35803=CARTESIAN_POINT('Origin',(-3.93836780768588,-0.398546858194397,12.25));
#35804=CARTESIAN_POINT('',(-3.83444475923175,-0.338546858194397,11.9));
#35805=CARTESIAN_POINT('',(-3.989475518093,-0.289974292889239,11.9));
#35806=CARTESIAN_POINT('Origin',(-3.93836780768588,-0.398546858194397,11.9));
#35807=CARTESIAN_POINT('',(-3.83444475923175,-0.338546858194397,12.25));
#35808=CARTESIAN_POINT('',(-3.989475518093,-0.289974292889239,12.25));
#35809=CARTESIAN_POINT('Origin',(-3.92598183048946,-0.895,11.9));
#35810=CARTESIAN_POINT('',(-3.10037094554829,-1.61,11.9));
#35811=CARTESIAN_POINT('Origin',(0.,0.,11.9));
#35812=CARTESIAN_POINT('Origin',(0.,0.,12.25));
#35813=CARTESIAN_POINT('Origin',(0.,0.,12.25));
#35814=CARTESIAN_POINT('Origin',(0.,0.,12.25));
#35815=CARTESIAN_POINT('Origin',(0.,0.,12.25));
#35816=CARTESIAN_POINT('Origin',(0.,0.,12.25));
#35817=CARTESIAN_POINT('Origin',(0.,0.,12.25));
#35818=CARTESIAN_POINT('',(0.436539071067832,3.97610785057841,12.25));
#35819=CARTESIAN_POINT('Origin',(0.,0.,12.25));
#35820=CARTESIAN_POINT('Origin',(0.,0.,12.25));
#35821=CARTESIAN_POINT('Origin',(0.,0.,12.25));
#35822=CARTESIAN_POINT('Origin',(0.,0.,12.25));
#35823=CARTESIAN_POINT('',(-3.22514087125372,2.36610785057841,12.25));
#35824=CARTESIAN_POINT('Origin',(0.,0.,12.25));
#35825=CARTESIAN_POINT('Origin',(0.,0.,12.25));
#35826=CARTESIAN_POINT('Origin',(2.11887548792593,-3.31,12.6));
#35827=CARTESIAN_POINT('Origin',(2.11887548792593,0.0900000000000001,12.6));
#35828=CARTESIAN_POINT('Origin',(1.13738003030356,-1.61,12.6));
#35829=CARTESIAN_POINT('Origin',(0.155884572681199,-3.31,12.6));
#35830=CARTESIAN_POINT('Origin',(2.94448637286709,1.88,12.6));
#35831=CARTESIAN_POINT('Origin',(1.96299091524473,0.18,12.6));
#35832=CARTESIAN_POINT('Origin',(-1.80710634256353,-3.31,12.6));
#35833=CARTESIAN_POINT('Origin',(0.981495457622364,1.88,12.6));
#35834=CARTESIAN_POINT('Origin',(-2.78860180018589,-1.61,12.6));
#35835=CARTESIAN_POINT('Origin',(-2.94448637286709,-1.88,12.6));
#35836=CARTESIAN_POINT('Origin',(-0.981495457622364,1.88,12.6));
#35837=CARTESIAN_POINT('Origin',(-1.96299091524473,0.18,12.6));
#35838=CARTESIAN_POINT('Origin',(-2.94448637286709,-1.52,12.6));
#35839=CARTESIAN_POINT('Origin',(-2.94448637286709,1.88,12.6));
#35840=CARTESIAN_POINT('Origin',(-3.92598183048946,-0.18,12.6));
#35841=CARTESIAN_POINT('Origin',(-3.77009725780826,0.0900000000000001,12.6));
#35842=CARTESIAN_POINT('Origin',(-2.78860180018589,1.79,12.6));
#35843=CARTESIAN_POINT('Origin',(-1.96299091524473,-3.22,12.6));
#35844=CARTESIAN_POINT('Origin',(-0.825610884941165,1.79,12.6));
#35845=CARTESIAN_POINT('Origin',(0.155884572681199,3.49,12.6));
#35846=CARTESIAN_POINT('Origin',(-1.80710634256353,-3.49,12.6));
#35847=CARTESIAN_POINT('Origin',(0.,-3.22,12.6));
#35848=CARTESIAN_POINT('Origin',(1.13738003030356,1.79,12.6));
#35849=CARTESIAN_POINT('Origin',(0.155884572681199,-3.49,12.6));
#35850=CARTESIAN_POINT('Origin',(1.96299091524473,-3.22,12.6));
#35851=CARTESIAN_POINT('Origin',(2.94448637286709,-1.52,12.6));
#35852=CARTESIAN_POINT('Origin',(3.92598183048946,0.18,12.6));
#35853=CARTESIAN_POINT('Origin',(3.10037094554829,-1.61,12.6));
#35854=CARTESIAN_POINT('Origin',(0.,0.,11.3));
#35855=CARTESIAN_POINT('',(-3.8,-4.65365783675994E-16,11.2));
#35856=CARTESIAN_POINT('',(-3.8,-4.65365783675994E-16,11.3));
#35857=CARTESIAN_POINT('Origin',(0.,0.,11.2));
#35858=CARTESIAN_POINT('Origin',(4.095,0.,11.2));
#35859=CARTESIAN_POINT('',(-4.095,-5.01492864250841E-16,11.2));
#35860=CARTESIAN_POINT('Origin',(0.,0.,11.2));
#35861=CARTESIAN_POINT('Origin',(0.,0.,11.3));
#35862=CARTESIAN_POINT('',(-4.095,-5.01492864250841E-16,11.3));
#35863=CARTESIAN_POINT('Origin',(0.,0.,12.2));
#35864=CARTESIAN_POINT('',(-0.9025,-1.10524373623049E-16,12.2));
#54962=UNCERTAINTY_MEASURE_WITH_UNIT(LENGTH_MEASURE(0.001),#55003,
'DISTANCE_ACCURACY_VALUE',
'Maximum model space distance between geometric entities at asserted c
onnectivities');
#54980=UNCERTAINTY_MEASURE_WITH_UNIT(LENGTH_MEASURE(0.001),#55003,
'DISTANCE_ACCURACY_VALUE',
'Maximum model space distance between geometric entities at asserted c
onnectivities');
#54984=(
GEOMETRIC_REPRESENTATION_CONTEXT(3)
GLOBAL_UNCERTAINTY_ASSIGNED_CONTEXT((#54962))
GLOBAL_UNIT_ASSIGNED_CONTEXT((#55003,#55005,#55006))
REPRESENTATION_CONTEXT('','3D')
);
#55002=(
GEOMETRIC_REPRESENTATION_CONTEXT(3)
GLOBAL_UNCERTAINTY_ASSIGNED_CONTEXT((#54980))
GLOBAL_UNIT_ASSIGNED_CONTEXT((#55003,#55005,#55006))
REPRESENTATION_CONTEXT('','3D')
);
#55003=(
LENGTH_UNIT()
NAMED_UNIT(*)
SI_UNIT(.CENTI.,.METRE.)
);
#55005=(
NAMED_UNIT(*)
PLANE_ANGLE_UNIT()
SI_UNIT($,.RADIAN.)
);
#55006=(
NAMED_UNIT(*)
SI_UNIT($,.STERADIAN.)
SOLID_ANGLE_UNIT()
);
#55010=SHAPE_DEFINITION_REPRESENTATION(#55031,#55106);
#55031=PRODUCT_DEFINITION_SHAPE('',$,#55128);
#55106=SHAPE_REPRESENTATION('',(#25058),#54984);
#55124=PRODUCT_DEFINITION_CONTEXT('part definition',#55189,'design');
#55128=PRODUCT_DEFINITION('2026-10-18-23-35-54-661',
'03_Isogrid_Motor_Mount_Faceplate',#55149,#55124);
#55149=PRODUCT_DEFINITION_FORMATION('',$,#55194);
#55189=APPLICATION_CONTEXT(
'Core Data for Automotive Mechanical Design Process');
#55190=PRODUCT_CONTEXT('part definition',#55189,'mechanical');
#55194=PRODUCT('2026-10-18-23-35-54-661',
'03_Isogrid_Motor_Mount_Faceplate',$,(#55190));
#55394=COLOUR_RGB('Off White',0.89,0.88,0.83);
#55395=FILL_AREA_STYLE_COLOUR('',#55394);
#55396=FILL_AREA_STYLE('',(#55395));
#55397=SURFACE_STYLE_FILL_AREA(#55396);
#55398=SURFACE_SIDE_STYLE('',(#55397));
#55399=SURFACE_STYLE_USAGE(.BOTH.,#55398);
#55400=PRESENTATION_STYLE_ASSIGNMENT((#55399));
ENDSEC;
END-ISO-10303-21;
